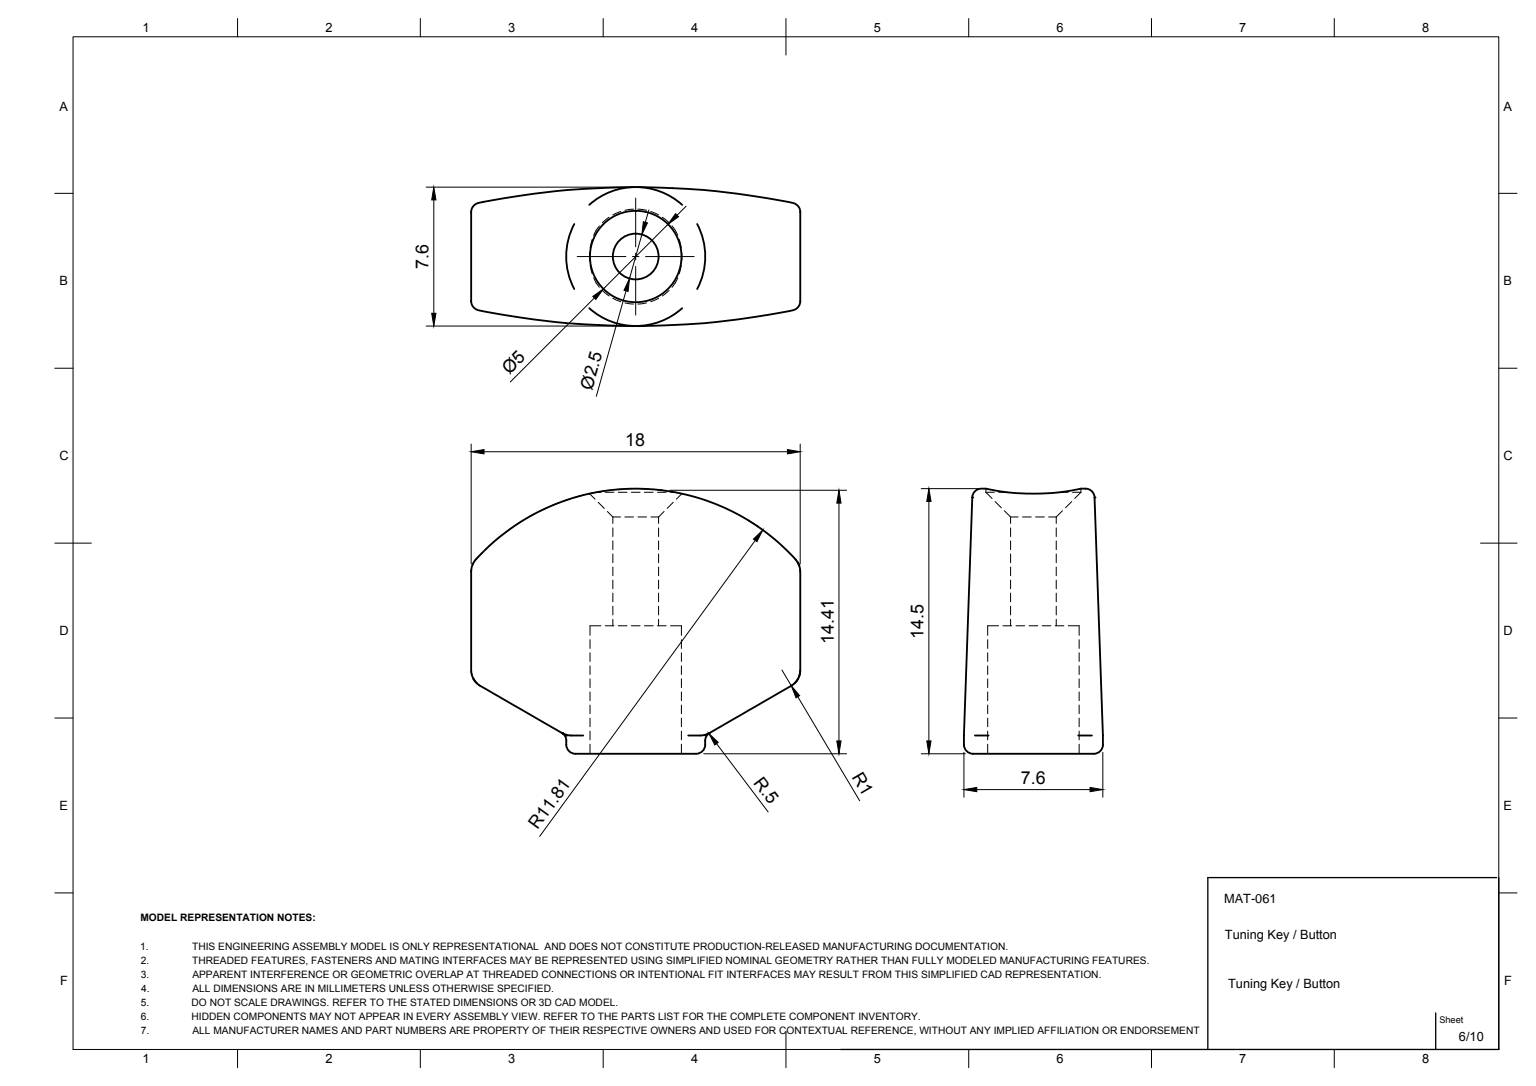
ISO-10303-21;
HEADER;
/* Generated by software containing ST-Developer
 * from STEP Tools, Inc. (www.steptools.com) 
 */

FILE_DESCRIPTION(
/* description */ ('', 'CAx-IF Rec.Pracs.---Representation and Presentation of Product Manufa
cturing Information (PMI)---4.0---2014-10-13'),
/* implementation_level */ '2;1');

FILE_NAME(
/* name */ 'Tuning Key _ Button.step',
/* time_stamp */ '2026-10-28T14:45:12+01:00',
/* author */ (''),
/* organization */ (''),
/* preprocessor_version */ 'ST-DEVELOPER v20.2',
/* originating_system */ 'Autodesk Translation Framework v15.17.0.0',
/* authorisation */ '');

FILE_SCHEMA (('AP242_MANAGED_MODEL_BASED_3D_ENGINEERING_MIM_LF { 1 0 10303 442 2 1 4 }'));
ENDSEC;

DATA;
#10=MECHANICAL_DESIGN_GEOMETRIC_PRESENTATION_REPRESENTATION('',(#263),#52164);
#84=ELLIPSE('',#9778,3.41583409365519,0.299010553745989);
#85=ELLIPSE('',#9779,1.15925578938865,0.129764384341253);
#86=ELLIPSE('',#9810,58.0067380360385,50.6192841142981);
#87=ELLIPSE('',#9813,1.18656669130194,0.53832789407732);
#88=ELLIPSE('',#9814,2.36619692333918,0.2327676175482);
#89=ELLIPSE('',#9837,58.0426595105096,50.6800723424155);
#90=ELLIPSE('',#9844,57.8529892126302,50.3590102148563);
#91=ELLIPSE('',#9882,57.6813518726037,50.0696217347841);
#128=(
BOUNDED_SURFACE()
B_SPLINE_SURFACE(3,3,((#29423,#29424,#29425,#29426,#29427,#29428,#29429,
#29430,#29431,#29432,#29433),(#29434,#29435,#29436,#29437,#29438,#29439,
#29440,#29441,#29442,#29443,#29444),(#29445,#29446,#29447,#29448,#29449,
#29450,#29451,#29452,#29453,#29454,#29455),(#29456,#29457,#29458,#29459,
#29460,#29461,#29462,#29463,#29464,#29465,#29466)),.UNSPECIFIED.,.F.,.F.,
 .F.)
B_SPLINE_SURFACE_WITH_KNOTS((4,4),(4,1,1,1,1,1,1,1,4),(0.,1.),(-0.02986974742742,
0.,0.1596527875626,0.3152888236561,0.4716393647845,0.6325142775716,0.8056128321368,
1.,1.030037265102),.UNSPECIFIED.)
GEOMETRIC_REPRESENTATION_ITEM()
RATIONAL_B_SPLINE_SURFACE(((1.021500558569,1.021500558569,1.021500558569,
1.021500558569,1.021500558569,1.021500558569,1.021500558569,1.021500558569,
1.021500558569,1.021500558569,1.021500558569),(0.9928331471435,0.9928331471435,
0.9928331471435,0.9928331471435,0.9928331471435,0.9928331471435,0.9928331471435,
0.9928331471435,0.9928331471435,0.9928331471435,0.9928331471435),(0.9928331471435,
0.9928331471435,0.9928331471435,0.9928331471435,0.9928331471435,0.9928331471435,
0.9928331471435,0.9928331471435,0.9928331471435,0.9928331471435,0.9928331471435),
(1.021500558569,1.021500558569,1.021500558569,1.021500558569,1.021500558569,
1.021500558569,1.021500558569,1.021500558569,1.021500558569,1.021500558569,
1.021500558569)))
REPRESENTATION_ITEM('')
SURFACE()
);
#129=(
BOUNDED_SURFACE()
B_SPLINE_SURFACE(3,3,((#29522,#29523,#29524,#29525,#29526,#29527,#29528,
#29529,#29530),(#29531,#29532,#29533,#29534,#29535,#29536,#29537,#29538,
#29539),(#29540,#29541,#29542,#29543,#29544,#29545,#29546,#29547,#29548),
(#29549,#29550,#29551,#29552,#29553,#29554,#29555,#29556,#29557)),
 .UNSPECIFIED.,.F.,.F.,.F.)
B_SPLINE_SURFACE_WITH_KNOTS((4,4),(4,1,1,1,1,1,4),(0.,1.),(-0.01572041923322,
0.,0.2489956052111,0.4846339404094,0.7277879443756,1.,1.015767529497),
 .UNSPECIFIED.)
GEOMETRIC_REPRESENTATION_ITEM()
RATIONAL_B_SPLINE_SURFACE(((1.20167030075,1.20167030075,1.20167030075,1.20167030075,
1.20167030075,1.20167030075,1.20167030075,1.20167030075,1.20167030075),
(0.9327765664168,0.9327765664168,0.9327765664168,0.9327765664168,0.9327765664168,
0.9327765664168,0.9327765664168,0.9327765664168,0.9327765664168),(0.9327765664168,
0.9327765664168,0.9327765664168,0.9327765664168,0.9327765664168,0.9327765664168,
0.9327765664168,0.9327765664168,0.9327765664168),(1.20167030075,1.20167030075,
1.20167030075,1.20167030075,1.20167030075,1.20167030075,1.20167030075,1.20167030075,
1.20167030075)))
REPRESENTATION_ITEM('')
SURFACE()
);
#130=(
BOUNDED_SURFACE()
B_SPLINE_SURFACE(3,3,((#29629,#29630,#29631,#29632,#29633,#29634,#29635,
#29636,#29637),(#29638,#29639,#29640,#29641,#29642,#29643,#29644,#29645,
#29646),(#29647,#29648,#29649,#29650,#29651,#29652,#29653,#29654,#29655),
(#29656,#29657,#29658,#29659,#29660,#29661,#29662,#29663,#29664)),
 .UNSPECIFIED.,.F.,.F.,.F.)
B_SPLINE_SURFACE_WITH_KNOTS((4,4),(4,1,1,1,1,1,4),(0.,1.),(-0.05556040640744,
0.,0.2510807745895,0.5005021153997,0.7496749190056,1.,1.055704479788),
 .UNSPECIFIED.)
GEOMETRIC_REPRESENTATION_ITEM()
RATIONAL_B_SPLINE_SURFACE(((1.211236736652,1.211236736652,1.211236736652,
1.211236736652,1.211236736652,1.211236736652,1.211236736652,1.211236736652,
1.211236736652),(0.9295877544494,0.9295877544494,0.9295877544494,0.9295877544494,
0.9295877544494,0.9295877544494,0.9295877544494,0.9295877544494,0.9295877544494),
(0.9295877544494,0.9295877544494,0.9295877544494,0.9295877544494,0.9295877544494,
0.9295877544494,0.9295877544494,0.9295877544494,0.9295877544494),(1.211236736652,
1.211236736652,1.211236736652,1.211236736652,1.211236736652,1.211236736652,
1.211236736652,1.211236736652,1.211236736652)))
REPRESENTATION_ITEM('')
SURFACE()
);
#131=(
BOUNDED_SURFACE()
B_SPLINE_SURFACE(3,3,((#29668,#29669,#29670,#29671,#29672,#29673,#29674,
#29675),(#29676,#29677,#29678,#29679,#29680,#29681,#29682,#29683),(#29684,
#29685,#29686,#29687,#29688,#29689,#29690,#29691),(#29692,#29693,#29694,
#29695,#29696,#29697,#29698,#29699)),.UNSPECIFIED.,.F.,.F.,.F.)
B_SPLINE_SURFACE_WITH_KNOTS((4,4),(4,1,1,1,1,4),(0.,1.),(0.8911674115136,
0.9072696780606,0.9355241084298,0.9657104248281,1.,1.001077582608),
 .UNSPECIFIED.)
GEOMETRIC_REPRESENTATION_ITEM()
RATIONAL_B_SPLINE_SURFACE(((1.199526961773,1.199526961773,1.199526961773,
1.199526961773,1.199526961773,1.199526961773,1.199526961773,1.199526961773),
(0.9334910127424,0.9334910127424,0.9334910127424,0.9334910127424,0.9334910127424,
0.9334910127424,0.9334910127424,0.9334910127424),(0.9334910127424,0.9334910127424,
0.9334910127424,0.9334910127424,0.9334910127424,0.9334910127424,0.9334910127424,
0.9334910127424),(1.199526961773,1.199526961773,1.199526961773,1.199526961773,
1.199526961773,1.199526961773,1.199526961773,1.199526961773)))
REPRESENTATION_ITEM('')
SURFACE()
);
#132=(
BOUNDED_SURFACE()
B_SPLINE_SURFACE(3,3,((#29815,#29816,#29817,#29818,#29819,#29820,#29821,
#29822,#29823,#29824,#29825),(#29826,#29827,#29828,#29829,#29830,#29831,
#29832,#29833,#29834,#29835,#29836),(#29837,#29838,#29839,#29840,#29841,
#29842,#29843,#29844,#29845,#29846,#29847),(#29848,#29849,#29850,#29851,
#29852,#29853,#29854,#29855,#29856,#29857,#29858)),.UNSPECIFIED.,.F.,.F.,
 .F.)
B_SPLINE_SURFACE_WITH_KNOTS((4,4),(4,1,1,1,1,1,1,1,4),(0.,1.),(-0.05042394646536,
0.,0.169599833297,0.3375196990485,0.507342039377,0.6686225111424,0.8285344877041,
1.,1.040577583792),.UNSPECIFIED.)
GEOMETRIC_REPRESENTATION_ITEM()
RATIONAL_B_SPLINE_SURFACE(((1.008087174025,1.008087174025,1.008087174025,
1.008087174025,1.008087174025,1.008087174025,1.008087174025,1.008087174025,
1.008087174025,1.008087174025,1.008087174025),(0.9973042753251,0.9973042753251,
0.9973042753251,0.9973042753251,0.9973042753251,0.9973042753251,0.9973042753251,
0.9973042753251,0.9973042753251,0.9973042753251,0.9973042753251),(0.9973042753251,
0.9973042753251,0.9973042753251,0.9973042753251,0.9973042753251,0.9973042753251,
0.9973042753251,0.9973042753251,0.9973042753251,0.9973042753251,0.9973042753251),
(1.008087174025,1.008087174025,1.008087174025,1.008087174025,1.008087174025,
1.008087174025,1.008087174025,1.008087174025,1.008087174025,1.008087174025,
1.008087174025)))
REPRESENTATION_ITEM('')
SURFACE()
);
#133=(
BOUNDED_SURFACE()
B_SPLINE_SURFACE(3,3,((#29905,#29906,#29907,#29908,#29909,#29910,#29911),
(#29912,#29913,#29914,#29915,#29916,#29917,#29918),(#29919,#29920,#29921,
#29922,#29923,#29924,#29925),(#29926,#29927,#29928,#29929,#29930,#29931,
#29932)),.UNSPECIFIED.,.F.,.F.,.F.)
B_SPLINE_SURFACE_WITH_KNOTS((4,4),(4,1,1,1,4),(0.,1.),(0.112613801722,0.3198611143952,
0.6533271535514,1.,1.02662543373),.UNSPECIFIED.)
GEOMETRIC_REPRESENTATION_ITEM()
RATIONAL_B_SPLINE_SURFACE(((1.133923634678,1.133923634678,1.133923634678,
1.133923634678,1.133923634678,1.133923634678,1.133923634678),(0.9553587884407,
0.9553587884407,0.9553587884407,0.9553587884407,0.9553587884407,0.9553587884407,
0.9553587884407),(0.9553587884407,0.9553587884407,0.9553587884407,0.9553587884407,
0.9553587884407,0.9553587884407,0.9553587884407),(1.133923634678,1.133923634678,
1.133923634678,1.133923634678,1.133923634678,1.133923634678,1.133923634678)))
REPRESENTATION_ITEM('')
SURFACE()
);
#134=(
BOUNDED_SURFACE()
B_SPLINE_SURFACE(3,3,((#30489,#30490,#30491,#30492,#30493,#30494,#30495,
#30496,#30497,#30498,#30499,#30500,#30501,#30502,#30503,#30504,#30505,#30506,
#30507),(#30508,#30509,#30510,#30511,#30512,#30513,#30514,#30515,#30516,
#30517,#30518,#30519,#30520,#30521,#30522,#30523,#30524,#30525,#30526),
(#30527,#30528,#30529,#30530,#30531,#30532,#30533,#30534,#30535,#30536,
#30537,#30538,#30539,#30540,#30541,#30542,#30543,#30544,#30545),(#30546,
#30547,#30548,#30549,#30550,#30551,#30552,#30553,#30554,#30555,#30556,#30557,
#30558,#30559,#30560,#30561,#30562,#30563,#30564)),.UNSPECIFIED.,.F.,.F.,
 .F.)
B_SPLINE_SURFACE_WITH_KNOTS((4,4),(4,1,1,1,1,1,1,1,1,1,1,1,1,1,1,1,4),(0.,
1.),(-0.01076426746052,0.,0.04152389901163,0.08394379225383,0.1302342687653,
0.1804523447143,0.2349355052965,0.2939338029968,0.3580057487009,0.4275129366519,
0.5025423241298,0.5839356639567,0.6731830882241,0.771794295847,0.880557504522,
1.,1.009808133051),.UNSPECIFIED.)
GEOMETRIC_REPRESENTATION_ITEM()
RATIONAL_B_SPLINE_SURFACE(((1.088372924818,1.088372924818,1.088372924818,
1.088372924818,1.088372924818,1.088372924818,1.088372924818,1.088372924818,
1.088372924818,1.088372924818,1.088372924818,1.088372924818,1.088372924818,
1.088372924818,1.088372924818,1.088372924818,1.088372924818,1.088372924818,
1.088372924818),(0.9705423583942,0.9705423583942,0.9705423583942,0.9705423583942,
0.9705423583942,0.9705423583942,0.9705423583942,0.9705423583942,0.9705423583942,
0.9705423583942,0.9705423583942,0.9705423583942,0.9705423583942,0.9705423583942,
0.9705423583942,0.9705423583942,0.9705423583942,0.9705423583942,0.9705423583942),
(0.9705423583942,0.9705423583942,0.9705423583942,0.9705423583942,0.9705423583942,
0.9705423583942,0.9705423583942,0.9705423583942,0.9705423583942,0.9705423583942,
0.9705423583942,0.9705423583942,0.9705423583942,0.9705423583942,0.9705423583942,
0.9705423583942,0.9705423583942,0.9705423583942,0.9705423583942),(1.088372924818,
1.088372924818,1.088372924818,1.088372924818,1.088372924818,1.088372924818,
1.088372924818,1.088372924818,1.088372924818,1.088372924818,1.088372924818,
1.088372924818,1.088372924818,1.088372924818,1.088372924818,1.088372924818,
1.088372924818,1.088372924818,1.088372924818)))
REPRESENTATION_ITEM('')
SURFACE()
);
#135=(
BOUNDED_SURFACE()
B_SPLINE_SURFACE(3,3,((#30667,#30668,#30669,#30670,#30671,#30672,#30673,
#30674,#30675,#30676),(#30677,#30678,#30679,#30680,#30681,#30682,#30683,
#30684,#30685,#30686),(#30687,#30688,#30689,#30690,#30691,#30692,#30693,
#30694,#30695,#30696),(#30697,#30698,#30699,#30700,#30701,#30702,#30703,
#30704,#30705,#30706)),.UNSPECIFIED.,.F.,.F.,.F.)
B_SPLINE_SURFACE_WITH_KNOTS((4,4),(4,1,1,1,1,1,1,4),(0.,1.),(0.03540281776569,
0.1234679415061,0.2632035734035,0.4203296727883,0.5957836491344,0.7892685013705,
1.,1.00911688994),.UNSPECIFIED.)
GEOMETRIC_REPRESENTATION_ITEM()
RATIONAL_B_SPLINE_SURFACE(((1.211236248281,1.211236248281,1.211236248281,
1.211236248281,1.211236248281,1.211236248281,1.211236248281,1.211236248281,
1.211236248281,1.211236248281),(0.9295879172397,0.9295879172397,0.9295879172397,
0.9295879172397,0.9295879172397,0.9295879172397,0.9295879172397,0.9295879172397,
0.9295879172397,0.9295879172397),(0.9295879172397,0.9295879172397,0.9295879172397,
0.9295879172397,0.9295879172397,0.9295879172397,0.9295879172397,0.9295879172397,
0.9295879172397,0.9295879172397),(1.211236248281,1.211236248281,1.211236248281,
1.211236248281,1.211236248281,1.211236248281,1.211236248281,1.211236248281,
1.211236248281,1.211236248281)))
REPRESENTATION_ITEM('')
SURFACE()
);
#136=(
BOUNDED_SURFACE()
B_SPLINE_SURFACE(3,3,((#30720,#30721,#30722,#30723,#30724,#30725,#30726,
#30727,#30728,#30729,#30730,#30731),(#30732,#30733,#30734,#30735,#30736,
#30737,#30738,#30739,#30740,#30741,#30742,#30743),(#30744,#30745,#30746,
#30747,#30748,#30749,#30750,#30751,#30752,#30753,#30754,#30755),(#30756,
#30757,#30758,#30759,#30760,#30761,#30762,#30763,#30764,#30765,#30766,#30767)),
 .UNSPECIFIED.,.F.,.F.,.F.)
B_SPLINE_SURFACE_WITH_KNOTS((4,4),(4,1,1,1,1,1,1,1,1,4),(0.,1.),(-0.1526180119247,
0.,0.1440925301464,0.2801219903111,0.411439159359,0.5434056701394,0.683264528579,
0.8346596058499,1.,1.152833582057),.UNSPECIFIED.)
GEOMETRIC_REPRESENTATION_ITEM()
RATIONAL_B_SPLINE_SURFACE(((1.000094023891,1.000094023891,1.000094023891,
1.000094023891,1.000094023891,1.000094023891,1.000094023891,1.000094023891,
1.000094023891,1.000094023891,1.000094023891,1.000094023891),(0.9999686587029,
0.9999686587029,0.9999686587029,0.9999686587029,0.9999686587029,0.9999686587029,
0.9999686587029,0.9999686587029,0.9999686587029,0.9999686587029,0.9999686587029,
0.9999686587029),(0.9999686587029,0.9999686587029,0.9999686587029,0.9999686587029,
0.9999686587029,0.9999686587029,0.9999686587029,0.9999686587029,0.9999686587029,
0.9999686587029,0.9999686587029,0.9999686587029),(1.000094023891,1.000094023891,
1.000094023891,1.000094023891,1.000094023891,1.000094023891,1.000094023891,
1.000094023891,1.000094023891,1.000094023891,1.000094023891,1.000094023891)))
REPRESENTATION_ITEM('')
SURFACE()
);
#137=(
BOUNDED_SURFACE()
B_SPLINE_SURFACE(3,3,((#30792,#30793,#30794,#30795,#30796,#30797,#30798,
#30799,#30800,#30801),(#30802,#30803,#30804,#30805,#30806,#30807,#30808,
#30809,#30810,#30811),(#30812,#30813,#30814,#30815,#30816,#30817,#30818,
#30819,#30820,#30821),(#30822,#30823,#30824,#30825,#30826,#30827,#30828,
#30829,#30830,#30831)),.UNSPECIFIED.,.F.,.F.,.F.)
B_SPLINE_SURFACE_WITH_KNOTS((4,4),(4,1,1,1,1,1,1,4),(0.,1.),(-0.009053405764055,
0.,0.2128253131464,0.406710340465,0.5817418357976,0.7383188923361,0.8773475428248,
0.9585687317144),.UNSPECIFIED.)
GEOMETRIC_REPRESENTATION_ITEM()
RATIONAL_B_SPLINE_SURFACE(((1.211237524847,1.211237524847,1.211237524847,
1.211237524847,1.211237524847,1.211237524847,1.211237524847,1.211237524847,
1.211237524847,1.211237524847),(0.9295874917176,0.9295874917176,0.9295874917176,
0.9295874917176,0.9295874917176,0.9295874917176,0.9295874917176,0.9295874917176,
0.9295874917176,0.9295874917176),(0.9295874917176,0.9295874917176,0.9295874917176,
0.9295874917176,0.9295874917176,0.9295874917176,0.9295874917176,0.9295874917176,
0.9295874917176,0.9295874917176),(1.211237524847,1.211237524847,1.211237524847,
1.211237524847,1.211237524847,1.211237524847,1.211237524847,1.211237524847,
1.211237524847,1.211237524847)))
REPRESENTATION_ITEM('')
SURFACE()
);
#138=(
BOUNDED_SURFACE()
B_SPLINE_SURFACE(3,3,((#30920,#30921,#30922,#30923,#30924,#30925,#30926,
#30927,#30928,#30929,#30930,#30931,#30932,#30933,#30934,#30935,#30936,#30937),
(#30938,#30939,#30940,#30941,#30942,#30943,#30944,#30945,#30946,#30947,
#30948,#30949,#30950,#30951,#30952,#30953,#30954,#30955),(#30956,#30957,
#30958,#30959,#30960,#30961,#30962,#30963,#30964,#30965,#30966,#30967,#30968,
#30969,#30970,#30971,#30972,#30973),(#30974,#30975,#30976,#30977,#30978,
#30979,#30980,#30981,#30982,#30983,#30984,#30985,#30986,#30987,#30988,#30989,
#30990,#30991)),.UNSPECIFIED.,.F.,.F.,.F.)
B_SPLINE_SURFACE_WITH_KNOTS((4,4),(4,1,1,1,1,1,1,1,1,1,1,1,1,1,1,4),(0.,
1.),(-0.009797090891185,0.,0.1252864769206,0.2381332273305,0.3395214867104,
0.4311702756132,0.514794596407,0.5913458810939,0.661337900673,0.7254151205028,
0.7843391271164,0.8380935847788,0.8886737238569,0.9411160876018,1.,1.010696795736),
 .UNSPECIFIED.)
GEOMETRIC_REPRESENTATION_ITEM()
RATIONAL_B_SPLINE_SURFACE(((1.088374512803,1.088374512803,1.088374512803,
1.088374512803,1.088374512803,1.088374512803,1.088374512803,1.088374512803,
1.088374512803,1.088374512803,1.088374512803,1.088374512803,1.088374512803,
1.088374512803,1.088374512803,1.088374512803,1.088374512803,1.088374512803),
(0.9705418290656,0.9705418290656,0.9705418290656,0.9705418290656,0.9705418290656,
0.9705418290656,0.9705418290656,0.9705418290655,0.9705418290656,0.9705418290656,
0.9705418290656,0.9705418290656,0.9705418290655,0.9705418290656,0.9705418290656,
0.9705418290655,0.9705418290656,0.9705418290656),(0.9705418290656,0.9705418290656,
0.9705418290656,0.9705418290656,0.9705418290656,0.9705418290656,0.9705418290656,
0.9705418290655,0.9705418290656,0.9705418290656,0.9705418290656,0.9705418290656,
0.9705418290655,0.9705418290656,0.9705418290656,0.9705418290655,0.9705418290656,
0.9705418290656),(1.088374512803,1.088374512803,1.088374512803,1.088374512803,
1.088374512803,1.088374512803,1.088374512803,1.088374512803,1.088374512803,
1.088374512803,1.088374512803,1.088374512803,1.088374512803,1.088374512803,
1.088374512803,1.088374512803,1.088374512803,1.088374512803)))
REPRESENTATION_ITEM('')
SURFACE()
);
#139=(
BOUNDED_SURFACE()
B_SPLINE_SURFACE(3,3,((#30993,#30994,#30995,#30996,#30997,#30998,#30999,
#31000,#31001),(#31002,#31003,#31004,#31005,#31006,#31007,#31008,#31009,
#31010),(#31011,#31012,#31013,#31014,#31015,#31016,#31017,#31018,#31019),
(#31020,#31021,#31022,#31023,#31024,#31025,#31026,#31027,#31028)),
 .UNSPECIFIED.,.F.,.F.,.F.)
B_SPLINE_SURFACE_WITH_KNOTS((4,4),(4,1,1,1,1,1,4),(0.,1.),(-0.01572041923323,
0.,0.2489956052094,0.4846339404077,0.7277879443747,1.,1.015767529497),
 .UNSPECIFIED.)
GEOMETRIC_REPRESENTATION_ITEM()
RATIONAL_B_SPLINE_SURFACE(((1.20167030075,1.20167030075,1.20167030075,1.20167030075,
1.20167030075,1.20167030075,1.20167030075,1.20167030075,1.20167030075),
(0.9327765664168,0.9327765664168,0.9327765664168,0.9327765664168,0.9327765664168,
0.9327765664168,0.9327765664168,0.9327765664168,0.9327765664168),(0.9327765664168,
0.9327765664168,0.9327765664168,0.9327765664168,0.9327765664168,0.9327765664168,
0.9327765664168,0.9327765664168,0.9327765664168),(1.20167030075,1.20167030075,
1.20167030075,1.20167030075,1.20167030075,1.20167030075,1.20167030075,1.20167030075,
1.20167030075)))
REPRESENTATION_ITEM('')
SURFACE()
);
#140=(
BOUNDED_SURFACE()
B_SPLINE_SURFACE(3,3,((#31065,#31066,#31067,#31068,#31069,#31070,#31071,
#31072,#31073),(#31074,#31075,#31076,#31077,#31078,#31079,#31080,#31081,
#31082),(#31083,#31084,#31085,#31086,#31087,#31088,#31089,#31090,#31091),
(#31092,#31093,#31094,#31095,#31096,#31097,#31098,#31099,#31100)),
 .UNSPECIFIED.,.F.,.F.,.F.)
B_SPLINE_SURFACE_WITH_KNOTS((4,4),(4,1,1,1,1,1,4),(0.,1.),(-0.05556027674448,
0.,0.2486256441043,0.4972385660022,0.747219976182,1.,1.055704281495),
 .UNSPECIFIED.)
GEOMETRIC_REPRESENTATION_ITEM()
RATIONAL_B_SPLINE_SURFACE(((1.211236736616,1.211236736616,1.211236736616,
1.211236736616,1.211236736616,1.211236736616,1.211236736616,1.211236736616,
1.211236736616),(0.9295877544614,0.9295877544614,0.9295877544614,0.9295877544614,
0.9295877544614,0.9295877544614,0.9295877544614,0.9295877544614,0.9295877544614),
(0.9295877544614,0.9295877544614,0.9295877544614,0.9295877544614,0.9295877544614,
0.9295877544614,0.9295877544614,0.9295877544614,0.9295877544614),(1.211236736616,
1.211236736616,1.211236736616,1.211236736616,1.211236736616,1.211236736616,
1.211236736616,1.211236736616,1.211236736616)))
REPRESENTATION_ITEM('')
SURFACE()
);
#141=(
BOUNDED_SURFACE()
B_SPLINE_SURFACE(3,3,((#31104,#31105,#31106,#31107,#31108,#31109,#31110,
#31111),(#31112,#31113,#31114,#31115,#31116,#31117,#31118,#31119),(#31120,
#31121,#31122,#31123,#31124,#31125,#31126,#31127),(#31128,#31129,#31130,
#31131,#31132,#31133,#31134,#31135)),.UNSPECIFIED.,.F.,.F.,.F.)
B_SPLINE_SURFACE_WITH_KNOTS((4,4),(4,1,1,1,1,4),(0.,1.),(0.8864361758264,
0.9023348460698,0.9320880776135,0.9638776326039,1.,1.001124438805),
 .UNSPECIFIED.)
GEOMETRIC_REPRESENTATION_ITEM()
RATIONAL_B_SPLINE_SURFACE(((1.199526961777,1.199526961777,1.199526961777,
1.199526961777,1.199526961777,1.199526961777,1.199526961777,1.199526961777),
(0.933491012741,0.933491012741,0.933491012741,0.933491012741,0.933491012741,
0.933491012741,0.933491012741,0.933491012741),(0.933491012741,0.933491012741,
0.933491012741,0.933491012741,0.933491012741,0.933491012741,0.933491012741,
0.933491012741),(1.199526961777,1.199526961777,1.199526961777,1.199526961777,
1.199526961777,1.199526961777,1.199526961777,1.199526961777)))
REPRESENTATION_ITEM('')
SURFACE()
);
#142=(
BOUNDED_SURFACE()
B_SPLINE_SURFACE(3,3,((#31139,#31140,#31141,#31142,#31143,#31144,#31145,
#31146,#31147,#31148),(#31149,#31150,#31151,#31152,#31153,#31154,#31155,
#31156,#31157,#31158),(#31159,#31160,#31161,#31162,#31163,#31164,#31165,
#31166,#31167,#31168),(#31169,#31170,#31171,#31172,#31173,#31174,#31175,
#31176,#31177,#31178)),.UNSPECIFIED.,.F.,.F.,.F.)
B_SPLINE_SURFACE_WITH_KNOTS((4,4),(4,1,1,1,1,1,1,4),(0.,1.),(-0.02782802324678,
0.,0.206830483526,0.4072723973775,0.5982739087583,0.7917037265225,1.,1.028080129965),
 .UNSPECIFIED.)
GEOMETRIC_REPRESENTATION_ITEM()
RATIONAL_B_SPLINE_SURFACE(((1.187634479555,1.187634479555,1.187634479555,
1.187634479555,1.187634479555,1.187634479555,1.187634479555,1.187634479555,
1.187634479555,1.187634479555),(0.9374551734818,0.9374551734818,0.9374551734818,
0.9374551734818,0.9374551734818,0.9374551734818,0.9374551734818,0.9374551734818,
0.9374551734818,0.9374551734818),(0.9374551734818,0.9374551734818,0.9374551734818,
0.9374551734818,0.9374551734818,0.9374551734818,0.9374551734818,0.9374551734818,
0.9374551734818,0.9374551734818),(1.187634479555,1.187634479555,1.187634479555,
1.187634479555,1.187634479555,1.187634479555,1.187634479555,1.187634479555,
1.187634479555,1.187634479555)))
REPRESENTATION_ITEM('')
SURFACE()
);
#143=(
BOUNDED_SURFACE()
B_SPLINE_SURFACE(3,3,((#31284,#31285,#31286,#31287,#31288,#31289,#31290,
#31291,#31292,#31293),(#31294,#31295,#31296,#31297,#31298,#31299,#31300,
#31301,#31302,#31303),(#31304,#31305,#31306,#31307,#31308,#31309,#31310,
#31311,#31312,#31313),(#31314,#31315,#31316,#31317,#31318,#31319,#31320,
#31321,#31322,#31323)),.UNSPECIFIED.,.F.,.F.,.F.)
B_SPLINE_SURFACE_WITH_KNOTS((4,4),(4,1,1,1,1,1,1,4),(0.,1.),(-0.02810100933582,
0.,0.2037887769512,0.4025777380169,0.5941765368876,0.7898232262628,1.,1.027817051165),
 .UNSPECIFIED.)
GEOMETRIC_REPRESENTATION_ITEM()
RATIONAL_B_SPLINE_SURFACE(((1.18763448144,1.18763448144,1.18763448144,1.18763448144,
1.18763448144,1.18763448144,1.18763448144,1.18763448144,1.18763448144,1.18763448144),
(0.9374551728533,0.9374551728533,0.9374551728533,0.9374551728533,0.9374551728533,
0.9374551728533,0.9374551728533,0.9374551728533,0.9374551728533,0.9374551728533),
(0.9374551728533,0.9374551728533,0.9374551728533,0.9374551728533,0.9374551728533,
0.9374551728533,0.9374551728533,0.9374551728533,0.9374551728533,0.9374551728533),
(1.18763448144,1.18763448144,1.18763448144,1.18763448144,1.18763448144,
1.18763448144,1.18763448144,1.18763448144,1.18763448144,1.18763448144)))
REPRESENTATION_ITEM('')
SURFACE()
);
#144=(
BOUNDED_SURFACE()
B_SPLINE_SURFACE(3,3,((#31368,#31369,#31370,#31371,#31372,#31373,#31374,
#31375),(#31376,#31377,#31378,#31379,#31380,#31381,#31382,#31383),(#31384,
#31385,#31386,#31387,#31388,#31389,#31390,#31391),(#31392,#31393,#31394,
#31395,#31396,#31397,#31398,#31399)),.UNSPECIFIED.,.F.,.F.,.F.)
B_SPLINE_SURFACE_WITH_KNOTS((4,4),(4,1,1,1,1,4),(0.,1.),(-0.001124474187882,
0.,0.0292220127923,0.0587438887651,0.09152259808643,0.1135644482631),
 .UNSPECIFIED.)
GEOMETRIC_REPRESENTATION_ITEM()
RATIONAL_B_SPLINE_SURFACE(((1.199526978638,1.199526978638,1.199526978638,
1.199526978638,1.199526978638,1.199526978638,1.199526978638,1.199526978638),
(0.9334910071206,0.9334910071206,0.9334910071206,0.9334910071206,0.9334910071206,
0.9334910071206,0.9334910071206,0.9334910071206),(0.9334910071206,0.9334910071206,
0.9334910071206,0.9334910071206,0.9334910071206,0.9334910071206,0.9334910071206,
0.9334910071206),(1.199526978638,1.199526978638,1.199526978638,1.199526978638,
1.199526978638,1.199526978638,1.199526978638,1.199526978638)))
REPRESENTATION_ITEM('')
SURFACE()
);
#145=(
BOUNDED_SURFACE()
B_SPLINE_SURFACE(3,3,((#31403,#31404,#31405,#31406,#31407,#31408,#31409,
#31410,#31411,#31412,#31413,#31414),(#31415,#31416,#31417,#31418,#31419,
#31420,#31421,#31422,#31423,#31424,#31425,#31426),(#31427,#31428,#31429,
#31430,#31431,#31432,#31433,#31434,#31435,#31436,#31437,#31438),(#31439,
#31440,#31441,#31442,#31443,#31444,#31445,#31446,#31447,#31448,#31449,#31450)),
 .UNSPECIFIED.,.F.,.F.,.F.)
B_SPLINE_SURFACE_WITH_KNOTS((4,4),(4,1,1,1,1,1,1,1,1,4),(0.,1.),(0.01735834385764,
0.1111047299147,0.222221140213,0.3333544708185,0.4444847206802,0.5555988587856,
0.6667216990803,0.777841116212,0.8889364520316,0.9880643576882),
 .UNSPECIFIED.)
GEOMETRIC_REPRESENTATION_ITEM()
RATIONAL_B_SPLINE_SURFACE(((1.211236726429,1.211236726429,1.211236726429,
1.211236726429,1.211236726429,1.211236726429,1.211236726429,1.211236726429,
1.211236726429,1.211236726429,1.211236726429,1.211236726429),(0.929587757857,
0.929587757857,0.929587757857,0.929587757857,0.929587757857,0.929587757857,
0.929587757857,0.929587757857,0.929587757857,0.929587757857,0.929587757857,
0.929587757857),(0.929587757857,0.929587757857,0.929587757857,0.929587757857,
0.929587757857,0.929587757857,0.929587757857,0.929587757857,0.929587757857,
0.929587757857,0.929587757857,0.929587757857),(1.211236726429,1.211236726429,
1.211236726429,1.211236726429,1.211236726429,1.211236726429,1.211236726429,
1.211236726429,1.211236726429,1.211236726429,1.211236726429,1.211236726429)))
REPRESENTATION_ITEM('')
SURFACE()
);
#146=(
BOUNDED_SURFACE()
B_SPLINE_SURFACE(3,3,((#31488,#31489,#31490,#31491,#31492,#31493,#31494,
#31495,#31496),(#31497,#31498,#31499,#31500,#31501,#31502,#31503,#31504,
#31505),(#31506,#31507,#31508,#31509,#31510,#31511,#31512,#31513,#31514),
(#31515,#31516,#31517,#31518,#31519,#31520,#31521,#31522,#31523)),
 .UNSPECIFIED.,.F.,.F.,.F.)
B_SPLINE_SURFACE_WITH_KNOTS((4,4),(4,1,1,1,1,1,4),(0.,1.),(-0.01575975614392,
0.,0.2456294260624,0.4801888085378,0.72700648837,1.,1.015733967826),
 .UNSPECIFIED.)
GEOMETRIC_REPRESENTATION_ITEM()
RATIONAL_B_SPLINE_SURFACE(((1.201670188537,1.201670188537,1.201670188537,
1.201670188537,1.201670188537,1.201670188537,1.201670188537,1.201670188537,
1.201670188537),(0.9327766038211,0.9327766038211,0.9327766038211,0.9327766038211,
0.9327766038211,0.9327766038211,0.9327766038211,0.9327766038211,0.9327766038211),
(0.9327766038211,0.9327766038211,0.9327766038211,0.9327766038211,0.9327766038211,
0.9327766038211,0.9327766038211,0.9327766038211,0.9327766038211),(1.201670188537,
1.201670188537,1.201670188537,1.201670188537,1.201670188537,1.201670188537,
1.201670188537,1.201670188537,1.201670188537)))
REPRESENTATION_ITEM('')
SURFACE()
);
#147=(
BOUNDED_SURFACE()
B_SPLINE_SURFACE(3,3,((#31570,#31571,#31572,#31573,#31574,#31575,#31576,
#31577,#31578,#31579),(#31580,#31581,#31582,#31583,#31584,#31585,#31586,
#31587,#31588,#31589),(#31590,#31591,#31592,#31593,#31594,#31595,#31596,
#31597,#31598,#31599),(#31600,#31601,#31602,#31603,#31604,#31605,#31606,
#31607,#31608,#31609)),.UNSPECIFIED.,.F.,.F.,.F.)
B_SPLINE_SURFACE_WITH_KNOTS((4,4),(4,1,1,1,1,1,1,4),(0.,1.),(-0.02987479217279,
0.,0.1922564273876,0.376033241946,0.5650637118402,0.769737337347,1.,1.030040321285),
 .UNSPECIFIED.)
GEOMETRIC_REPRESENTATION_ITEM()
RATIONAL_B_SPLINE_SURFACE(((1.02150055857,1.02150055857,1.02150055857,1.02150055857,
1.02150055857,1.02150055857,1.02150055857,1.02150055857,1.02150055857,1.02150055857),
(0.9928331471434,0.9928331471434,0.9928331471434,0.9928331471434,0.9928331471434,
0.9928331471434,0.9928331471434,0.9928331471434,0.9928331471434,0.9928331471434),
(0.9928331471434,0.9928331471434,0.9928331471434,0.9928331471434,0.9928331471434,
0.9928331471434,0.9928331471434,0.9928331471434,0.9928331471434,0.9928331471434),
(1.02150055857,1.02150055857,1.02150055857,1.02150055857,1.02150055857,
1.02150055857,1.02150055857,1.02150055857,1.02150055857,1.02150055857)))
REPRESENTATION_ITEM('')
SURFACE()
);
#148=(
BOUNDED_SURFACE()
B_SPLINE_SURFACE(3,3,((#31612,#31613,#31614,#31615,#31616,#31617,#31618,
#31619,#31620),(#31621,#31622,#31623,#31624,#31625,#31626,#31627,#31628,
#31629),(#31630,#31631,#31632,#31633,#31634,#31635,#31636,#31637,#31638),
(#31639,#31640,#31641,#31642,#31643,#31644,#31645,#31646,#31647)),
 .UNSPECIFIED.,.F.,.F.,.F.)
B_SPLINE_SURFACE_WITH_KNOTS((4,4),(4,1,1,1,1,1,4),(0.,1.),(-0.05038062996365,
0.,0.2351349496917,0.4696037900664,0.7241664476852,1.,1.040579001464),
 .UNSPECIFIED.)
GEOMETRIC_REPRESENTATION_ITEM()
RATIONAL_B_SPLINE_SURFACE(((1.008087784169,1.008087784169,1.008087784169,
1.008087784169,1.008087784169,1.008087784169,1.008087784169,1.008087784169,
1.008087784169),(0.9973040719437,0.9973040719437,0.9973040719437,0.9973040719437,
0.9973040719437,0.9973040719437,0.9973040719437,0.9973040719437,0.9973040719437),
(0.9973040719437,0.9973040719437,0.9973040719437,0.9973040719437,0.9973040719437,
0.9973040719437,0.9973040719437,0.9973040719437,0.9973040719437),(1.008087784169,
1.008087784169,1.008087784169,1.008087784169,1.008087784169,1.008087784169,
1.008087784169,1.008087784169,1.008087784169)))
REPRESENTATION_ITEM('')
SURFACE()
);
#149=(
BOUNDED_SURFACE()
B_SPLINE_SURFACE(3,3,((#31685,#31686,#31687,#31688,#31689,#31690,#31691),
(#31692,#31693,#31694,#31695,#31696,#31697,#31698),(#31699,#31700,#31701,
#31702,#31703,#31704,#31705),(#31706,#31707,#31708,#31709,#31710,#31711,
#31712)),.UNSPECIFIED.,.F.,.F.,.F.)
B_SPLINE_SURFACE_WITH_KNOTS((4,4),(4,1,1,1,4),(0.,1.),(-0.02191865670978,
0.,0.3711108307934,0.7030029884295,0.8666418147817),.UNSPECIFIED.)
GEOMETRIC_REPRESENTATION_ITEM()
RATIONAL_B_SPLINE_SURFACE(((1.201671391236,1.201671391236,1.201671391236,
1.201671391236,1.201671391236,1.201671391236,1.201671391236),(0.9327762029212,
0.9327762029212,0.9327762029212,0.9327762029212,0.9327762029212,0.9327762029212,
0.9327762029212),(0.9327762029212,0.9327762029212,0.9327762029212,0.9327762029212,
0.9327762029212,0.9327762029212,0.9327762029212),(1.201671391236,1.201671391236,
1.201671391236,1.201671391236,1.201671391236,1.201671391236,1.201671391236)))
REPRESENTATION_ITEM('')
SURFACE()
);
#150=(
BOUNDED_SURFACE()
B_SPLINE_SURFACE(3,3,((#31714,#31715,#31716,#31717,#31718,#31719,#31720,
#31721),(#31722,#31723,#31724,#31725,#31726,#31727,#31728,#31729),(#31730,
#31731,#31732,#31733,#31734,#31735,#31736,#31737),(#31738,#31739,#31740,
#31741,#31742,#31743,#31744,#31745)),.UNSPECIFIED.,.F.,.F.,.F.)
B_SPLINE_SURFACE_WITH_KNOTS((4,4),(4,1,1,1,1,4),(0.,1.),(-0.01121526784147,
0.,0.3190655160223,0.6396471045238,1.,1.011194064343),.UNSPECIFIED.)
GEOMETRIC_REPRESENTATION_ITEM()
RATIONAL_B_SPLINE_SURFACE(((1.095350229527,1.095350229527,1.095350229527,
1.095350229527,1.095350229527,1.095350229527,1.095350229527,1.095350229527),
(0.9682165901577,0.9682165901577,0.9682165901577,0.9682165901577,0.9682165901577,
0.9682165901577,0.9682165901577,0.9682165901577),(0.9682165901577,0.9682165901577,
0.9682165901577,0.9682165901577,0.9682165901577,0.9682165901577,0.9682165901577,
0.9682165901577),(1.095350229527,1.095350229527,1.095350229527,1.095350229527,
1.095350229527,1.095350229527,1.095350229527,1.095350229527)))
REPRESENTATION_ITEM('')
SURFACE()
);
#151=(
BOUNDED_SURFACE()
B_SPLINE_SURFACE(3,3,((#31747,#31748,#31749,#31750,#31751,#31752,#31753,
#31754),(#31755,#31756,#31757,#31758,#31759,#31760,#31761,#31762),(#31763,
#31764,#31765,#31766,#31767,#31768,#31769,#31770),(#31771,#31772,#31773,
#31774,#31775,#31776,#31777,#31778)),.UNSPECIFIED.,.F.,.F.,.F.)
B_SPLINE_SURFACE_WITH_KNOTS((4,4),(4,1,1,1,1,4),(0.,1.),(-0.01123151966199,
0.,0.3226423274774,0.6411748598112,1.,1.011214131254),.UNSPECIFIED.)
GEOMETRIC_REPRESENTATION_ITEM()
RATIONAL_B_SPLINE_SURFACE(((1.095350237894,1.095350237894,1.095350237894,
1.095350237894,1.095350237894,1.095350237894,1.095350237894,1.095350237894),
(0.9682165873688,0.9682165873688,0.9682165873688,0.9682165873688,0.9682165873688,
0.9682165873688,0.9682165873688,0.9682165873688),(0.9682165873688,0.9682165873688,
0.9682165873688,0.9682165873688,0.9682165873688,0.9682165873688,0.9682165873688,
0.9682165873688),(1.095350237894,1.095350237894,1.095350237894,1.095350237894,
1.095350237894,1.095350237894,1.095350237894,1.095350237894)))
REPRESENTATION_ITEM('')
SURFACE()
);
#152=(
BOUNDED_SURFACE()
B_SPLINE_SURFACE(3,3,((#31780,#31781,#31782,#31783,#31784,#31785,#31786),
(#31787,#31788,#31789,#31790,#31791,#31792,#31793),(#31794,#31795,#31796,
#31797,#31798,#31799,#31800),(#31801,#31802,#31803,#31804,#31805,#31806,
#31807)),.UNSPECIFIED.,.F.,.F.,.F.)
B_SPLINE_SURFACE_WITH_KNOTS((4,4),(4,1,1,1,4),(0.,1.),(0.1126138017486,
0.319861120519,0.6533271596459,1.,1.026625433703),.UNSPECIFIED.)
GEOMETRIC_REPRESENTATION_ITEM()
RATIONAL_B_SPLINE_SURFACE(((1.133923637937,1.133923637937,1.133923637937,
1.133923637937,1.133923637937,1.133923637937,1.133923637937),(0.9553587873545,
0.9553587873545,0.9553587873545,0.9553587873545,0.9553587873545,0.9553587873545,
0.9553587873545),(0.9553587873545,0.9553587873545,0.9553587873545,0.9553587873545,
0.9553587873545,0.9553587873545,0.9553587873545),(1.133923637937,1.133923637937,
1.133923637937,1.133923637937,1.133923637937,1.133923637937,1.133923637937)))
REPRESENTATION_ITEM('')
SURFACE()
);
#153=(
BOUNDED_SURFACE()
B_SPLINE_SURFACE(3,3,((#31844,#31845,#31846,#31847,#31848,#31849,#31850,
#31851,#31852,#31853,#31854),(#31855,#31856,#31857,#31858,#31859,#31860,
#31861,#31862,#31863,#31864,#31865),(#31866,#31867,#31868,#31869,#31870,
#31871,#31872,#31873,#31874,#31875,#31876),(#31877,#31878,#31879,#31880,
#31881,#31882,#31883,#31884,#31885,#31886,#31887)),.UNSPECIFIED.,.F.,.F.,
 .F.)
B_SPLINE_SURFACE_WITH_KNOTS((4,4),(4,1,1,1,1,1,1,1,4),(0.,1.),(-0.04051174551792,
0.,0.1601684695697,0.3176853418238,0.4756542837724,0.6362846105788,0.8070461231236,
1.,1.048408689707),.UNSPECIFIED.)
GEOMETRIC_REPRESENTATION_ITEM()
RATIONAL_B_SPLINE_SURFACE(((1.008087174024,1.008087174024,1.008087174024,
1.008087174024,1.008087174024,1.008087174024,1.008087174024,1.008087174024,
1.008087174024,1.008087174024,1.008087174024),(0.9973042753252,0.9973042753252,
0.9973042753252,0.9973042753252,0.9973042753252,0.9973042753252,0.9973042753252,
0.9973042753252,0.9973042753252,0.9973042753252,0.9973042753252),(0.9973042753252,
0.9973042753252,0.9973042753252,0.9973042753252,0.9973042753252,0.9973042753252,
0.9973042753252,0.9973042753252,0.9973042753252,0.9973042753252,0.9973042753252),
(1.008087174024,1.008087174024,1.008087174024,1.008087174024,1.008087174024,
1.008087174024,1.008087174024,1.008087174024,1.008087174024,1.008087174024,
1.008087174024)))
REPRESENTATION_ITEM('')
SURFACE()
);
#154=(
BOUNDED_SURFACE()
B_SPLINE_SURFACE(3,3,((#31889,#31890,#31891,#31892,#31893,#31894,#31895,
#31896,#31897),(#31898,#31899,#31900,#31901,#31902,#31903,#31904,#31905,
#31906),(#31907,#31908,#31909,#31910,#31911,#31912,#31913,#31914,#31915),
(#31916,#31917,#31918,#31919,#31920,#31921,#31922,#31923,#31924)),
 .UNSPECIFIED.,.F.,.F.,.F.)
B_SPLINE_SURFACE_WITH_KNOTS((4,4),(4,1,1,1,1,1,4),(0.,1.),(-0.02991897955271,
0.,0.2239749897618,0.4574668129281,0.7131740843088,1.,1.029884092175),
 .UNSPECIFIED.)
GEOMETRIC_REPRESENTATION_ITEM()
RATIONAL_B_SPLINE_SURFACE(((1.021500558577,1.021500558577,1.021500558577,
1.021500558577,1.021500558577,1.021500558577,1.021500558577,1.021500558577,
1.021500558577),(0.992833147141,0.992833147141,0.992833147141,0.992833147141,
0.992833147141,0.992833147141,0.992833147141,0.992833147141,0.992833147141),
(0.992833147141,0.992833147141,0.992833147141,0.992833147141,0.992833147141,
0.992833147141,0.992833147141,0.992833147141,0.992833147141),(1.021500558577,
1.021500558577,1.021500558577,1.021500558577,1.021500558577,1.021500558577,
1.021500558577,1.021500558577,1.021500558577)))
REPRESENTATION_ITEM('')
SURFACE()
);
#155=(
BOUNDED_SURFACE()
B_SPLINE_SURFACE(3,3,((#31992,#31993,#31994,#31995,#31996,#31997,#31998,
#31999,#32000,#32001,#32002),(#32003,#32004,#32005,#32006,#32007,#32008,
#32009,#32010,#32011,#32012,#32013),(#32014,#32015,#32016,#32017,#32018,
#32019,#32020,#32021,#32022,#32023,#32024),(#32025,#32026,#32027,#32028,
#32029,#32030,#32031,#32032,#32033,#32034,#32035)),.UNSPECIFIED.,.F.,.F.,
 .F.)
B_SPLINE_SURFACE_WITH_KNOTS((4,4),(4,1,1,1,1,1,1,1,4),(0.,1.),(-0.02991442636641,
0.,0.1652192384749,0.3271780455741,0.486578186817,0.6458635561448,0.8144083932013,
1.,1.029876740826),.UNSPECIFIED.)
GEOMETRIC_REPRESENTATION_ITEM()
RATIONAL_B_SPLINE_SURFACE(((1.021500558569,1.021500558569,1.021500558569,
1.021500558569,1.021500558569,1.021500558569,1.021500558569,1.021500558569,
1.021500558569,1.021500558569,1.021500558569),(0.9928331471435,0.9928331471435,
0.9928331471435,0.9928331471435,0.9928331471435,0.9928331471435,0.9928331471435,
0.9928331471435,0.9928331471435,0.9928331471435,0.9928331471435),(0.9928331471435,
0.9928331471435,0.9928331471435,0.9928331471435,0.9928331471435,0.9928331471435,
0.9928331471435,0.9928331471435,0.9928331471435,0.9928331471435,0.9928331471435),
(1.021500558569,1.021500558569,1.021500558569,1.021500558569,1.021500558569,
1.021500558569,1.021500558569,1.021500558569,1.021500558569,1.021500558569,
1.021500558569)))
REPRESENTATION_ITEM('')
SURFACE()
);
#156=(
BOUNDED_SURFACE()
B_SPLINE_SURFACE(3,3,((#32040,#32041,#32042,#32043,#32044,#32045,#32046,
#32047,#32048,#32049,#32050,#32051),(#32052,#32053,#32054,#32055,#32056,
#32057,#32058,#32059,#32060,#32061,#32062,#32063),(#32064,#32065,#32066,
#32067,#32068,#32069,#32070,#32071,#32072,#32073,#32074,#32075),(#32076,
#32077,#32078,#32079,#32080,#32081,#32082,#32083,#32084,#32085,#32086,#32087)),
 .UNSPECIFIED.,.F.,.F.,.F.)
B_SPLINE_SURFACE_WITH_KNOTS((4,4),(4,1,1,1,1,1,1,1,1,4),(0.,1.),(0.0119111100004,
0.111104700859,0.2222213328836,0.3333553389617,0.4444873410571,0.5556025705647,
0.6667268893849,0.7778458691404,0.888938349439,0.9826188152285),
 .UNSPECIFIED.)
GEOMETRIC_REPRESENTATION_ITEM()
RATIONAL_B_SPLINE_SURFACE(((1.211236726733,1.211236726733,1.211236726733,
1.211236726733,1.211236726733,1.211236726733,1.211236726733,1.211236726733,
1.211236726733,1.211236726733,1.211236726733,1.211236726733),(0.9295877577556,
0.9295877577556,0.9295877577556,0.9295877577556,0.9295877577556,0.9295877577556,
0.9295877577556,0.9295877577556,0.9295877577556,0.9295877577556,0.9295877577556,
0.9295877577556),(0.9295877577556,0.9295877577556,0.9295877577556,0.9295877577556,
0.9295877577556,0.9295877577556,0.9295877577556,0.9295877577556,0.9295877577556,
0.9295877577556,0.9295877577556,0.9295877577556),(1.211236726733,1.211236726733,
1.211236726733,1.211236726733,1.211236726733,1.211236726733,1.211236726733,
1.211236726733,1.211236726733,1.211236726733,1.211236726733,1.211236726733)))
REPRESENTATION_ITEM('')
SURFACE()
);
#157=(
BOUNDED_SURFACE()
B_SPLINE_SURFACE(3,3,((#32123,#32124,#32125,#32126,#32127,#32128,#32129,
#32130,#32131),(#32132,#32133,#32134,#32135,#32136,#32137,#32138,#32139,
#32140),(#32141,#32142,#32143,#32144,#32145,#32146,#32147,#32148,#32149),
(#32150,#32151,#32152,#32153,#32154,#32155,#32156,#32157,#32158)),
 .UNSPECIFIED.,.F.,.F.,.F.)
B_SPLINE_SURFACE_WITH_KNOTS((4,4),(4,1,1,1,1,1,4),(0.,1.),(-0.01575975614391,
0.,0.2456294260624,0.4801888085378,0.7270064883701,1.,1.015733967826),
 .UNSPECIFIED.)
GEOMETRIC_REPRESENTATION_ITEM()
RATIONAL_B_SPLINE_SURFACE(((1.201670188537,1.201670188537,1.201670188537,
1.201670188537,1.201670188537,1.201670188537,1.201670188537,1.201670188537,
1.201670188537),(0.9327766038211,0.9327766038211,0.9327766038211,0.9327766038211,
0.9327766038211,0.9327766038211,0.9327766038211,0.9327766038211,0.9327766038211),
(0.9327766038211,0.9327766038211,0.9327766038211,0.9327766038211,0.9327766038211,
0.9327766038211,0.9327766038211,0.9327766038211,0.9327766038211),(1.201670188537,
1.201670188537,1.201670188537,1.201670188537,1.201670188537,1.201670188537,
1.201670188537,1.201670188537,1.201670188537)))
REPRESENTATION_ITEM('')
SURFACE()
);
#158=(
BOUNDED_SURFACE()
B_SPLINE_SURFACE(3,3,((#32368,#32369,#32370,#32371,#32372,#32373,#32374,
#32375),(#32376,#32377,#32378,#32379,#32380,#32381,#32382,#32383),(#32384,
#32385,#32386,#32387,#32388,#32389,#32390,#32391),(#32392,#32393,#32394,
#32395,#32396,#32397,#32398,#32399)),.UNSPECIFIED.,.F.,.F.,.F.)
B_SPLINE_SURFACE_WITH_KNOTS((4,4),(4,1,1,1,1,4),(0.,1.),(-0.02000000006299,
0.,0.3331237554216,0.6664570887615,1.,1.020000003967),.UNSPECIFIED.)
GEOMETRIC_REPRESENTATION_ITEM()
RATIONAL_B_SPLINE_SURFACE(((1.158475807259,1.158475807259,1.158475807259,
1.158475807259,1.158475807259,1.158475807259,1.158475807259,1.158475807259),
(0.9471747309136,0.9471747309136,0.9471747309136,0.9471747309136,0.9471747309136,
0.9471747309136,0.9471747309136,0.9471747309136),(0.9471747309136,0.9471747309136,
0.9471747309136,0.9471747309136,0.9471747309136,0.9471747309136,0.9471747309136,
0.9471747309136),(1.158475807259,1.158475807259,1.158475807259,1.158475807259,
1.158475807259,1.158475807259,1.158475807259,1.158475807259)))
REPRESENTATION_ITEM('')
SURFACE()
);
#159=(
BOUNDED_SURFACE()
B_SPLINE_SURFACE(3,3,((#32407,#32408,#32409,#32410,#32411,#32412,#32413,
#32414),(#32415,#32416,#32417,#32418,#32419,#32420,#32421,#32422),(#32423,
#32424,#32425,#32426,#32427,#32428,#32429,#32430),(#32431,#32432,#32433,
#32434,#32435,#32436,#32437,#32438)),.UNSPECIFIED.,.F.,.F.,.F.)
B_SPLINE_SURFACE_WITH_KNOTS((4,4),(4,1,1,1,1,4),(0.,1.),(-0.02,0.,0.3335430444131,
0.666876377753,1.,1.019999999985),.UNSPECIFIED.)
GEOMETRIC_REPRESENTATION_ITEM()
RATIONAL_B_SPLINE_SURFACE(((1.158475807259,1.158475807259,1.158475807259,
1.158475807259,1.158475807259,1.158475807259,1.158475807259,1.158475807259),
(0.9471747309136,0.9471747309136,0.9471747309136,0.9471747309136,0.9471747309136,
0.9471747309136,0.9471747309136,0.9471747309136),(0.9471747309136,0.9471747309136,
0.9471747309136,0.9471747309136,0.9471747309136,0.9471747309136,0.9471747309136,
0.9471747309136),(1.158475807259,1.158475807259,1.158475807259,1.158475807259,
1.158475807259,1.158475807259,1.158475807259,1.158475807259)))
REPRESENTATION_ITEM('')
SURFACE()
);
#160=(
BOUNDED_SURFACE()
B_SPLINE_SURFACE(3,3,((#32665,#32666,#32667,#32668,#32669,#32670,#32671,
#32672,#32673,#32674),(#32675,#32676,#32677,#32678,#32679,#32680,#32681,
#32682,#32683,#32684),(#32685,#32686,#32687,#32688,#32689,#32690,#32691,
#32692,#32693,#32694),(#32695,#32696,#32697,#32698,#32699,#32700,#32701,
#32702,#32703,#32704)),.UNSPECIFIED.,.F.,.F.,.F.)
B_SPLINE_SURFACE_WITH_KNOTS((4,4),(4,1,1,1,1,1,1,4),(0.,1.),(-0.02782793672778,
0.,0.2061198945833,0.405852717027,0.5969792694224,0.7914070803093,1.,1.028079856947),
 .UNSPECIFIED.)
GEOMETRIC_REPRESENTATION_ITEM()
RATIONAL_B_SPLINE_SURFACE(((1.187634479517,1.187634479517,1.187634479517,
1.187634479517,1.187634479517,1.187634479517,1.187634479517,1.187634479517,
1.187634479517,1.187634479517),(0.9374551734942,0.9374551734942,0.9374551734942,
0.9374551734942,0.9374551734942,0.9374551734942,0.9374551734942,0.9374551734942,
0.9374551734942,0.9374551734942),(0.9374551734942,0.9374551734942,0.9374551734942,
0.9374551734942,0.9374551734942,0.9374551734942,0.9374551734942,0.9374551734942,
0.9374551734942,0.9374551734942),(1.187634479517,1.187634479517,1.187634479517,
1.187634479517,1.187634479517,1.187634479517,1.187634479517,1.187634479517,
1.187634479517,1.187634479517)))
REPRESENTATION_ITEM('')
SURFACE()
);
#161=(
BOUNDED_SURFACE()
B_SPLINE_SURFACE(3,3,((#32793,#32794,#32795,#32796,#32797,#32798,#32799,
#32800,#32801,#32802),(#32803,#32804,#32805,#32806,#32807,#32808,#32809,
#32810,#32811,#32812),(#32813,#32814,#32815,#32816,#32817,#32818,#32819,
#32820,#32821,#32822),(#32823,#32824,#32825,#32826,#32827,#32828,#32829,
#32830,#32831,#32832)),.UNSPECIFIED.,.F.,.F.,.F.)
B_SPLINE_SURFACE_WITH_KNOTS((4,4),(4,1,1,1,1,1,1,4),(0.,1.),(-0.02810083996936,
0.,0.2044929737017,0.4039878177866,0.5954658095825,0.7901158902839,1.,1.027817073056),
 .UNSPECIFIED.)
GEOMETRIC_REPRESENTATION_ITEM()
RATIONAL_B_SPLINE_SURFACE(((1.187634481559,1.187634481559,1.187634481559,
1.187634481559,1.187634481559,1.187634481559,1.187634481559,1.187634481559,
1.187634481559,1.187634481559),(0.9374551728136,0.9374551728136,0.9374551728136,
0.9374551728136,0.9374551728136,0.9374551728136,0.9374551728136,0.9374551728136,
0.9374551728136,0.9374551728136),(0.9374551728136,0.9374551728136,0.9374551728136,
0.9374551728136,0.9374551728136,0.9374551728136,0.9374551728136,0.9374551728136,
0.9374551728136,0.9374551728136),(1.187634481559,1.187634481559,1.187634481559,
1.187634481559,1.187634481559,1.187634481559,1.187634481559,1.187634481559,
1.187634481559,1.187634481559)))
REPRESENTATION_ITEM('')
SURFACE()
);
#162=(
BOUNDED_SURFACE()
B_SPLINE_SURFACE(3,3,((#32835,#32836,#32837,#32838,#32839,#32840,#32841,
#32842),(#32843,#32844,#32845,#32846,#32847,#32848,#32849,#32850),(#32851,
#32852,#32853,#32854,#32855,#32856,#32857,#32858),(#32859,#32860,#32861,
#32862,#32863,#32864,#32865,#32866)),.UNSPECIFIED.,.F.,.F.,.F.)
B_SPLINE_SURFACE_WITH_KNOTS((4,4),(4,1,1,1,1,4),(0.,1.),(-0.001077616544647,
0.,0.0278179355033,0.0559228241955,0.08712239292215,0.1088331409388),
 .UNSPECIFIED.)
GEOMETRIC_REPRESENTATION_ITEM()
RATIONAL_B_SPLINE_SURFACE(((1.199526979016,1.199526979016,1.199526979016,
1.199526979016,1.199526979016,1.199526979016,1.199526979016,1.199526979016),
(0.9334910069946,0.9334910069946,0.9334910069946,0.9334910069946,0.9334910069946,
0.9334910069946,0.9334910069946,0.9334910069946),(0.9334910069946,0.9334910069946,
0.9334910069946,0.9334910069946,0.9334910069946,0.9334910069946,0.9334910069946,
0.9334910069946),(1.199526979016,1.199526979016,1.199526979016,1.199526979016,
1.199526979016,1.199526979016,1.199526979016,1.199526979016)))
REPRESENTATION_ITEM('')
SURFACE()
);
#163=(
BOUNDED_SURFACE()
B_SPLINE_SURFACE(3,3,((#32867,#32868,#32869,#32870,#32871,#32872,#32873,
#32874),(#32875,#32876,#32877,#32878,#32879,#32880,#32881,#32882),(#32883,
#32884,#32885,#32886,#32887,#32888,#32889,#32890),(#32891,#32892,#32893,
#32894,#32895,#32896,#32897,#32898)),.UNSPECIFIED.,.F.,.F.,.F.)
B_SPLINE_SURFACE_WITH_KNOTS((4,4),(4,1,1,1,1,4),(0.,1.),(-0.02,0.,0.3335430447055,
0.6668763780453,1.,1.019999999985),.UNSPECIFIED.)
GEOMETRIC_REPRESENTATION_ITEM()
RATIONAL_B_SPLINE_SURFACE(((1.158475807259,1.158475807259,1.158475807259,
1.158475807259,1.158475807259,1.158475807259,1.158475807259,1.158475807259),
(0.9471747309136,0.9471747309136,0.9471747309136,0.9471747309136,0.9471747309136,
0.9471747309136,0.9471747309136,0.9471747309136),(0.9471747309136,0.9471747309136,
0.9471747309136,0.9471747309136,0.9471747309136,0.9471747309136,0.9471747309136,
0.9471747309136),(1.158475807259,1.158475807259,1.158475807259,1.158475807259,
1.158475807259,1.158475807259,1.158475807259,1.158475807259)))
REPRESENTATION_ITEM('')
SURFACE()
);
#164=(
BOUNDED_SURFACE()
B_SPLINE_SURFACE(3,3,((#32906,#32907,#32908,#32909,#32910,#32911,#32912,
#32913),(#32914,#32915,#32916,#32917,#32918,#32919,#32920,#32921),(#32922,
#32923,#32924,#32925,#32926,#32927,#32928,#32929),(#32930,#32931,#32932,
#32933,#32934,#32935,#32936,#32937)),.UNSPECIFIED.,.F.,.F.,.F.)
B_SPLINE_SURFACE_WITH_KNOTS((4,4),(4,1,1,1,1,4),(0.,1.),(-0.02000000007603,
0.,0.3331237556924,0.6664570890323,1.,1.020000004632),.UNSPECIFIED.)
GEOMETRIC_REPRESENTATION_ITEM()
RATIONAL_B_SPLINE_SURFACE(((1.158475807259,1.158475807259,1.158475807259,
1.158475807259,1.158475807259,1.158475807259,1.158475807259,1.158475807259),
(0.9471747309136,0.9471747309136,0.9471747309136,0.9471747309136,0.9471747309136,
0.9471747309136,0.9471747309136,0.9471747309136),(0.9471747309136,0.9471747309136,
0.9471747309136,0.9471747309136,0.9471747309136,0.9471747309136,0.9471747309136,
0.9471747309136),(1.158475807259,1.158475807259,1.158475807259,1.158475807259,
1.158475807259,1.158475807259,1.158475807259,1.158475807259)))
REPRESENTATION_ITEM('')
SURFACE()
);
#165=(
BOUNDED_SURFACE()
B_SPLINE_SURFACE(3,3,((#32939,#32940,#32941,#32942,#32943,#32944,#32945,
#32946,#32947),(#32948,#32949,#32950,#32951,#32952,#32953,#32954,#32955,
#32956),(#32957,#32958,#32959,#32960,#32961,#32962,#32963,#32964,#32965),
(#32966,#32967,#32968,#32969,#32970,#32971,#32972,#32973,#32974)),
 .UNSPECIFIED.,.F.,.F.,.F.)
B_SPLINE_SURFACE_WITH_KNOTS((4,4),(4,1,1,1,1,1,4),(0.,1.),(-0.03990139320459,
0.,0.2383747185699,0.4794833111693,0.7307955330181,1.,1.039731692604),
 .UNSPECIFIED.)
GEOMETRIC_REPRESENTATION_ITEM()
RATIONAL_B_SPLINE_SURFACE(((1.163827495202,1.163827495202,1.163827495202,
1.163827495202,1.163827495202,1.163827495202,1.163827495202,1.163827495202,
1.163827495202),(0.9453908349325,0.9453908349325,0.9453908349325,0.9453908349325,
0.9453908349325,0.9453908349325,0.9453908349325,0.9453908349325,0.9453908349325),
(0.9453908349325,0.9453908349325,0.9453908349325,0.9453908349325,0.9453908349325,
0.9453908349325,0.9453908349325,0.9453908349325,0.9453908349325),(1.163827495202,
1.163827495202,1.163827495202,1.163827495202,1.163827495202,1.163827495202,
1.163827495202,1.163827495202,1.163827495202)))
REPRESENTATION_ITEM('')
SURFACE()
);
#166=(
BOUNDED_SURFACE()
B_SPLINE_SURFACE(3,3,((#33033,#33034,#33035,#33036,#33037,#33038,#33039,
#33040,#33041),(#33042,#33043,#33044,#33045,#33046,#33047,#33048,#33049,
#33050),(#33051,#33052,#33053,#33054,#33055,#33056,#33057,#33058,#33059),
(#33060,#33061,#33062,#33063,#33064,#33065,#33066,#33067,#33068)),
 .UNSPECIFIED.,.F.,.F.,.F.)
B_SPLINE_SURFACE_WITH_KNOTS((4,4),(4,1,1,1,1,1,4),(0.,1.),(-0.03973821722907,
0.,0.2388826440098,0.4802432095543,0.7314080978693,1.,1.039877733719),
 .UNSPECIFIED.)
GEOMETRIC_REPRESENTATION_ITEM()
RATIONAL_B_SPLINE_SURFACE(((1.163827493612,1.163827493612,1.163827493612,
1.163827493612,1.163827493612,1.163827493612,1.163827493612,1.163827493612,
1.163827493612),(0.9453908354627,0.9453908354627,0.9453908354627,0.9453908354627,
0.9453908354627,0.9453908354627,0.9453908354627,0.9453908354627,0.9453908354627),
(0.9453908354627,0.9453908354627,0.9453908354627,0.9453908354627,0.9453908354627,
0.9453908354627,0.9453908354627,0.9453908354627,0.9453908354627),(1.163827493612,
1.163827493612,1.163827493612,1.163827493612,1.163827493612,1.163827493612,
1.163827493612,1.163827493612,1.163827493612)))
REPRESENTATION_ITEM('')
SURFACE()
);
#167=(
BOUNDED_SURFACE()
B_SPLINE_SURFACE(3,3,((#33070,#33071,#33072,#33073,#33074,#33075,#33076,
#33077,#33078,#33079,#33080,#33081,#33082,#33083,#33084,#33085,#33086,#33087,
#33088,#33089,#33090,#33091,#33092,#33093,#33094,#33095,#33096,#33097,#33098,
#33099,#33100,#33101),(#33102,#33103,#33104,#33105,#33106,#33107,#33108,
#33109,#33110,#33111,#33112,#33113,#33114,#33115,#33116,#33117,#33118,#33119,
#33120,#33121,#33122,#33123,#33124,#33125,#33126,#33127,#33128,#33129,#33130,
#33131,#33132,#33133),(#33134,#33135,#33136,#33137,#33138,#33139,#33140,
#33141,#33142,#33143,#33144,#33145,#33146,#33147,#33148,#33149,#33150,#33151,
#33152,#33153,#33154,#33155,#33156,#33157,#33158,#33159,#33160,#33161,#33162,
#33163,#33164,#33165),(#33166,#33167,#33168,#33169,#33170,#33171,#33172,
#33173,#33174,#33175,#33176,#33177,#33178,#33179,#33180,#33181,#33182,#33183,
#33184,#33185,#33186,#33187,#33188,#33189,#33190,#33191,#33192,#33193,#33194,
#33195,#33196,#33197)),.UNSPECIFIED.,.F.,.F.,.F.)
B_SPLINE_SURFACE_WITH_KNOTS((4,4),(4,1,1,1,1,1,1,1,1,1,1,1,1,1,1,1,1,1,
1,1,1,1,1,1,1,1,1,1,1,4),(0.,1.),(-0.009989617270159,0.,0.0587369296208,
0.111068550249,0.1581000808001,0.2003396839717,0.2384448290796,0.2747221985793,
0.3117544904028,0.3494937277553,0.3869465899255,0.4242215507061,0.4615931261968,
0.499066395259,0.5364199609172,0.5733902772176,0.6100694635878,0.6464467903499,
0.6809974474155,0.7120024196009,0.7411742705344,0.7707771184994,0.8006196344549,
0.8302940356761,0.8602243035839,0.8909644083677,0.9237463930732,0.9597502743101,
1.,1.009989117017),.UNSPECIFIED.)
GEOMETRIC_REPRESENTATION_ITEM()
RATIONAL_B_SPLINE_SURFACE(((1.192397230944,1.192397230944,1.192397230944,
1.192397230944,1.192397230944,1.192397230944,1.192397230944,1.192397230944,
1.192397230944,1.192397230944,1.192397230944,1.192397230944,1.192397230944,
1.192397230944,1.192397230944,1.192397230944,1.192397230944,1.192397230944,
1.192397230944,1.192397230944,1.192397230944,1.192397230944,1.192397230944,
1.192397230944,1.192397230944,1.192397230944,1.192397230944,1.192397230944,
1.192397230944,1.192397230944,1.192397230944,1.192397230944),(0.9358675896855,
0.9358675896855,0.9358675896855,0.9358675896855,0.9358675896855,0.9358675896855,
0.9358675896855,0.9358675896855,0.9358675896855,0.9358675896855,0.9358675896855,
0.9358675896855,0.9358675896855,0.9358675896855,0.9358675896855,0.9358675896855,
0.9358675896855,0.9358675896855,0.9358675896855,0.9358675896855,0.9358675896855,
0.9358675896855,0.9358675896855,0.9358675896855,0.9358675896855,0.9358675896855,
0.9358675896855,0.9358675896855,0.9358675896855,0.9358675896855,0.9358675896855,
0.9358675896855),(0.9358675896855,0.9358675896855,0.9358675896855,0.9358675896855,
0.9358675896855,0.9358675896855,0.9358675896855,0.9358675896855,0.9358675896855,
0.9358675896855,0.9358675896855,0.9358675896855,0.9358675896855,0.9358675896855,
0.9358675896855,0.9358675896855,0.9358675896855,0.9358675896855,0.9358675896855,
0.9358675896855,0.9358675896855,0.9358675896855,0.9358675896855,0.9358675896855,
0.9358675896855,0.9358675896855,0.9358675896855,0.9358675896855,0.9358675896855,
0.9358675896855,0.9358675896855,0.9358675896855),(1.192397230944,1.192397230944,
1.192397230944,1.192397230944,1.192397230944,1.192397230944,1.192397230944,
1.192397230944,1.192397230944,1.192397230944,1.192397230944,1.192397230944,
1.192397230944,1.192397230944,1.192397230944,1.192397230944,1.192397230944,
1.192397230944,1.192397230944,1.192397230944,1.192397230944,1.192397230944,
1.192397230944,1.192397230944,1.192397230944,1.192397230944,1.192397230944,
1.192397230944,1.192397230944,1.192397230944,1.192397230944,1.192397230944)))
REPRESENTATION_ITEM('')
SURFACE()
);
#168=(
BOUNDED_SURFACE()
B_SPLINE_SURFACE(3,3,((#33666,#33667,#33668,#33669,#33670,#33671,#33672,
#33673,#33674,#33675,#33676,#33677,#33678,#33679,#33680,#33681,#33682,#33683,
#33684,#33685,#33686,#33687,#33688,#33689,#33690,#33691,#33692,#33693,#33694,
#33695,#33696,#33697),(#33698,#33699,#33700,#33701,#33702,#33703,#33704,
#33705,#33706,#33707,#33708,#33709,#33710,#33711,#33712,#33713,#33714,#33715,
#33716,#33717,#33718,#33719,#33720,#33721,#33722,#33723,#33724,#33725,#33726,
#33727,#33728,#33729),(#33730,#33731,#33732,#33733,#33734,#33735,#33736,
#33737,#33738,#33739,#33740,#33741,#33742,#33743,#33744,#33745,#33746,#33747,
#33748,#33749,#33750,#33751,#33752,#33753,#33754,#33755,#33756,#33757,#33758,
#33759,#33760,#33761),(#33762,#33763,#33764,#33765,#33766,#33767,#33768,
#33769,#33770,#33771,#33772,#33773,#33774,#33775,#33776,#33777,#33778,#33779,
#33780,#33781,#33782,#33783,#33784,#33785,#33786,#33787,#33788,#33789,#33790,
#33791,#33792,#33793)),.UNSPECIFIED.,.F.,.F.,.F.)
B_SPLINE_SURFACE_WITH_KNOTS((4,4),(4,1,1,1,1,1,1,1,1,1,1,1,1,1,1,1,1,1,
1,1,1,1,1,1,1,1,1,1,1,4),(0.,1.),(-0.009989616921005,0.,0.05872646932563,
0.1110508073303,0.1580780876269,0.2003155443802,0.2384155963746,0.2746745689611,
0.3116781024864,0.3493943002845,0.3868271443784,0.4240772685742,0.4614186760705,
0.4988604389596,0.5361879081759,0.5731414127621,0.6098108086259,0.6461939396313,
0.6807803323384,0.7118281019108,0.7410274548133,0.7706525155955,0.8005231162647,
0.8302238307092,0.8601755167066,0.89093194483,0.9237248042115,0.9597384770757,
1.,1.009989116574),.UNSPECIFIED.)
GEOMETRIC_REPRESENTATION_ITEM()
RATIONAL_B_SPLINE_SURFACE(((1.192397251387,1.192397251387,1.192397251387,
1.192397251387,1.192397251387,1.192397251387,1.192397251387,1.192397251387,
1.192397251387,1.192397251387,1.192397251387,1.192397251387,1.192397251387,
1.192397251387,1.192397251387,1.192397251387,1.192397251387,1.192397251387,
1.192397251387,1.192397251387,1.192397251387,1.192397251387,1.192397251387,
1.192397251387,1.192397251387,1.192397251387,1.192397251387,1.192397251387,
1.192397251387,1.192397251387,1.192397251387,1.192397251387),(0.935867582871,
0.935867582871,0.935867582871,0.935867582871,0.935867582871,0.935867582871,
0.935867582871,0.935867582871,0.935867582871,0.935867582871,0.935867582871,
0.935867582871,0.935867582871,0.935867582871,0.935867582871,0.935867582871,
0.935867582871,0.935867582871,0.935867582871,0.935867582871,0.935867582871,
0.935867582871,0.935867582871,0.935867582871,0.935867582871,0.935867582871,
0.935867582871,0.935867582871,0.935867582871,0.935867582871,0.935867582871,
0.935867582871),(0.935867582871,0.935867582871,0.935867582871,0.935867582871,
0.935867582871,0.935867582871,0.935867582871,0.935867582871,0.935867582871,
0.935867582871,0.935867582871,0.935867582871,0.935867582871,0.935867582871,
0.935867582871,0.935867582871,0.935867582871,0.935867582871,0.935867582871,
0.935867582871,0.935867582871,0.935867582871,0.935867582871,0.935867582871,
0.935867582871,0.935867582871,0.935867582871,0.935867582871,0.935867582871,
0.935867582871,0.935867582871,0.935867582871),(1.192397251387,1.192397251387,
1.192397251387,1.192397251387,1.192397251387,1.192397251387,1.192397251387,
1.192397251387,1.192397251387,1.192397251387,1.192397251387,1.192397251387,
1.192397251387,1.192397251387,1.192397251387,1.192397251387,1.192397251387,
1.192397251387,1.192397251387,1.192397251387,1.192397251387,1.192397251387,
1.192397251387,1.192397251387,1.192397251387,1.192397251387,1.192397251387,
1.192397251387,1.192397251387,1.192397251387,1.192397251387,1.192397251387)))
REPRESENTATION_ITEM('')
SURFACE()
);
#169=(
BOUNDED_SURFACE()
B_SPLINE_SURFACE(3,3,((#33795,#33796,#33797,#33798,#33799,#33800,#33801,
#33802,#33803),(#33804,#33805,#33806,#33807,#33808,#33809,#33810,#33811,
#33812),(#33813,#33814,#33815,#33816,#33817,#33818,#33819,#33820,#33821),
(#33822,#33823,#33824,#33825,#33826,#33827,#33828,#33829,#33830)),
 .UNSPECIFIED.,.F.,.F.,.F.)
B_SPLINE_SURFACE_WITH_KNOTS((4,4),(4,1,1,1,1,1,4),(0.,1.),(-0.03973820027638,
0.,0.238622357915,0.4800568473432,0.731387517944,1.,1.03987771478),
 .UNSPECIFIED.)
GEOMETRIC_REPRESENTATION_ITEM()
RATIONAL_B_SPLINE_SURFACE(((1.163827493602,1.163827493602,1.163827493602,
1.163827493602,1.163827493602,1.163827493602,1.163827493602,1.163827493602,
1.163827493602),(0.9453908354662,0.9453908354662,0.9453908354662,0.9453908354662,
0.9453908354662,0.9453908354662,0.9453908354662,0.9453908354662,0.9453908354662),
(0.9453908354662,0.9453908354662,0.9453908354662,0.9453908354662,0.9453908354662,
0.9453908354662,0.9453908354662,0.9453908354662,0.9453908354662),(1.163827493602,
1.163827493602,1.163827493602,1.163827493602,1.163827493602,1.163827493602,
1.163827493602,1.163827493602,1.163827493602)))
REPRESENTATION_ITEM('')
SURFACE()
);
#170=(
BOUNDED_SURFACE()
B_SPLINE_SURFACE(3,3,((#33888,#33889,#33890,#33891,#33892,#33893,#33894,
#33895,#33896),(#33897,#33898,#33899,#33900,#33901,#33902,#33903,#33904,
#33905),(#33906,#33907,#33908,#33909,#33910,#33911,#33912,#33913,#33914),
(#33915,#33916,#33917,#33918,#33919,#33920,#33921,#33922,#33923)),
 .UNSPECIFIED.,.F.,.F.,.F.)
B_SPLINE_SURFACE_WITH_KNOTS((4,4),(4,1,1,1,1,1,4),(0.,1.),(-0.03990137353967,
0.,0.2386413019669,0.4796774710128,0.7308215928377,1.,1.039731675547),
 .UNSPECIFIED.)
GEOMETRIC_REPRESENTATION_ITEM()
RATIONAL_B_SPLINE_SURFACE(((1.163827495208,1.163827495208,1.163827495208,
1.163827495208,1.163827495208,1.163827495208,1.163827495208,1.163827495208,
1.163827495208),(0.9453908349308,0.9453908349308,0.9453908349308,0.9453908349308,
0.9453908349308,0.9453908349308,0.9453908349308,0.9453908349308,0.9453908349308),
(0.9453908349308,0.9453908349308,0.9453908349308,0.9453908349308,0.9453908349308,
0.9453908349308,0.9453908349308,0.9453908349308,0.9453908349308),(1.163827495208,
1.163827495208,1.163827495208,1.163827495208,1.163827495208,1.163827495208,
1.163827495208,1.163827495208,1.163827495208)))
REPRESENTATION_ITEM('')
SURFACE()
);
#171=(
BOUNDED_SURFACE()
B_SPLINE_SURFACE(3,3,((#33924,#33925,#33926,#33927,#33928,#33929,#33930,
#33931,#33932,#33933),(#33934,#33935,#33936,#33937,#33938,#33939,#33940,
#33941,#33942,#33943),(#33944,#33945,#33946,#33947,#33948,#33949,#33950,
#33951,#33952,#33953),(#33954,#33955,#33956,#33957,#33958,#33959,#33960,
#33961,#33962,#33963)),.UNSPECIFIED.,.F.,.F.,.F.)
B_SPLINE_SURFACE_WITH_KNOTS((4,4),(4,1,1,1,1,1,1,4),(0.,1.),(0.03540281776569,
0.1234679415063,0.2632035734038,0.4203296727887,0.5957836491349,0.789268501371,
1.,1.00911688994),.UNSPECIFIED.)
GEOMETRIC_REPRESENTATION_ITEM()
RATIONAL_B_SPLINE_SURFACE(((1.211236248281,1.211236248281,1.211236248281,
1.211236248281,1.211236248281,1.211236248281,1.211236248281,1.211236248281,
1.211236248281,1.211236248281),(0.9295879172397,0.9295879172397,0.9295879172397,
0.9295879172397,0.9295879172397,0.9295879172397,0.9295879172397,0.9295879172397,
0.9295879172397,0.9295879172397),(0.9295879172397,0.9295879172397,0.9295879172397,
0.9295879172397,0.9295879172397,0.9295879172397,0.9295879172397,0.9295879172397,
0.9295879172397,0.9295879172397),(1.211236248281,1.211236248281,1.211236248281,
1.211236248281,1.211236248281,1.211236248281,1.211236248281,1.211236248281,
1.211236248281,1.211236248281)))
REPRESENTATION_ITEM('')
SURFACE()
);
#172=(
BOUNDED_SURFACE()
B_SPLINE_SURFACE(3,3,((#34041,#34042,#34043,#34044,#34045,#34046,#34047,
#34048,#34049,#34050,#34051,#34052,#34053,#34054,#34055,#34056,#34057,#34058,
#34059),(#34060,#34061,#34062,#34063,#34064,#34065,#34066,#34067,#34068,
#34069,#34070,#34071,#34072,#34073,#34074,#34075,#34076,#34077,#34078),
(#34079,#34080,#34081,#34082,#34083,#34084,#34085,#34086,#34087,#34088,
#34089,#34090,#34091,#34092,#34093,#34094,#34095,#34096,#34097),(#34098,
#34099,#34100,#34101,#34102,#34103,#34104,#34105,#34106,#34107,#34108,#34109,
#34110,#34111,#34112,#34113,#34114,#34115,#34116)),.UNSPECIFIED.,.F.,.F.,
 .F.)
B_SPLINE_SURFACE_WITH_KNOTS((4,4),(4,1,1,1,1,1,1,1,1,1,1,1,1,1,1,1,4),(0.,
1.),(-0.01076426746053,0.,0.04152389901166,0.08394379225387,0.1302342687654,
0.1804523447143,0.2349355052966,0.2939338029969,0.3580057487009,0.4275129366519,
0.5025423241297,0.5839356639565,0.6731830882238,0.7717942958468,0.8805575045219,
1.,1.009808133051),.UNSPECIFIED.)
GEOMETRIC_REPRESENTATION_ITEM()
RATIONAL_B_SPLINE_SURFACE(((1.088372924818,1.088372924818,1.088372924818,
1.088372924818,1.088372924818,1.088372924818,1.088372924818,1.088372924818,
1.088372924818,1.088372924818,1.088372924818,1.088372924818,1.088372924818,
1.088372924818,1.088372924818,1.088372924818,1.088372924818,1.088372924818,
1.088372924818),(0.9705423583942,0.9705423583942,0.9705423583942,0.9705423583942,
0.9705423583942,0.9705423583942,0.9705423583942,0.9705423583942,0.9705423583942,
0.9705423583942,0.9705423583942,0.9705423583942,0.9705423583942,0.9705423583942,
0.9705423583942,0.9705423583942,0.9705423583942,0.9705423583942,0.9705423583942),
(0.9705423583942,0.9705423583942,0.9705423583942,0.9705423583942,0.9705423583942,
0.9705423583942,0.9705423583942,0.9705423583942,0.9705423583942,0.9705423583942,
0.9705423583942,0.9705423583942,0.9705423583942,0.9705423583942,0.9705423583942,
0.9705423583942,0.9705423583942,0.9705423583942,0.9705423583942),(1.088372924818,
1.088372924818,1.088372924818,1.088372924818,1.088372924818,1.088372924818,
1.088372924818,1.088372924818,1.088372924818,1.088372924818,1.088372924818,
1.088372924818,1.088372924818,1.088372924818,1.088372924818,1.088372924818,
1.088372924818,1.088372924818,1.088372924818)))
REPRESENTATION_ITEM('')
SURFACE()
);
#173=(
BOUNDED_SURFACE()
B_SPLINE_SURFACE(3,3,((#34117,#34118,#34119,#34120,#34121,#34122,#34123,
#34124,#34125,#34126,#34127,#34128),(#34129,#34130,#34131,#34132,#34133,
#34134,#34135,#34136,#34137,#34138,#34139,#34140),(#34141,#34142,#34143,
#34144,#34145,#34146,#34147,#34148,#34149,#34150,#34151,#34152),(#34153,
#34154,#34155,#34156,#34157,#34158,#34159,#34160,#34161,#34162,#34163,#34164)),
 .UNSPECIFIED.,.F.,.F.,.F.)
B_SPLINE_SURFACE_WITH_KNOTS((4,4),(4,1,1,1,1,1,1,1,1,4),(0.,1.),(-0.152618011925,
0.,0.1440925301842,0.2801219903658,0.4114391594101,0.5434056701778,0.6832645286048,
0.8346596058642,1.,1.152833582056),.UNSPECIFIED.)
GEOMETRIC_REPRESENTATION_ITEM()
RATIONAL_B_SPLINE_SURFACE(((1.000094023891,1.000094023891,1.000094023891,
1.000094023891,1.000094023891,1.000094023891,1.000094023891,1.000094023891,
1.000094023891,1.000094023891,1.000094023891,1.000094023891),(0.9999686587029,
0.9999686587029,0.9999686587029,0.9999686587029,0.9999686587029,0.9999686587029,
0.9999686587029,0.9999686587029,0.9999686587029,0.9999686587029,0.9999686587029,
0.9999686587029),(0.9999686587029,0.9999686587029,0.9999686587029,0.9999686587029,
0.9999686587029,0.9999686587029,0.9999686587029,0.9999686587029,0.9999686587029,
0.9999686587029,0.9999686587029,0.9999686587029),(1.000094023891,1.000094023891,
1.000094023891,1.000094023891,1.000094023891,1.000094023891,1.000094023891,
1.000094023891,1.000094023891,1.000094023891,1.000094023891,1.000094023891)))
REPRESENTATION_ITEM('')
SURFACE()
);
#174=(
BOUNDED_SURFACE()
B_SPLINE_SURFACE(3,3,((#34166,#34167,#34168,#34169,#34170,#34171,#34172,
#34173,#34174,#34175),(#34176,#34177,#34178,#34179,#34180,#34181,#34182,
#34183,#34184,#34185),(#34186,#34187,#34188,#34189,#34190,#34191,#34192,
#34193,#34194,#34195),(#34196,#34197,#34198,#34199,#34200,#34201,#34202,
#34203,#34204,#34205)),.UNSPECIFIED.,.F.,.F.,.F.)
B_SPLINE_SURFACE_WITH_KNOTS((4,4),(4,1,1,1,1,1,1,4),(0.,1.),(-0.009053405764054,
0.,0.2128253131466,0.4067103404652,0.5817418357977,0.7383188923361,0.8773475428248,
0.9585687317144),.UNSPECIFIED.)
GEOMETRIC_REPRESENTATION_ITEM()
RATIONAL_B_SPLINE_SURFACE(((1.211237524847,1.211237524847,1.211237524847,
1.211237524847,1.211237524847,1.211237524847,1.211237524847,1.211237524847,
1.211237524847,1.211237524847),(0.9295874917176,0.9295874917176,0.9295874917176,
0.9295874917176,0.9295874917176,0.9295874917176,0.9295874917176,0.9295874917176,
0.9295874917176,0.9295874917176),(0.9295874917176,0.9295874917176,0.9295874917176,
0.9295874917176,0.9295874917176,0.9295874917176,0.9295874917176,0.9295874917176,
0.9295874917176,0.9295874917176),(1.211237524847,1.211237524847,1.211237524847,
1.211237524847,1.211237524847,1.211237524847,1.211237524847,1.211237524847,
1.211237524847,1.211237524847)))
REPRESENTATION_ITEM('')
SURFACE()
);
#175=(
BOUNDED_SURFACE()
B_SPLINE_SURFACE(3,3,((#34282,#34283,#34284,#34285,#34286,#34287,#34288,
#34289,#34290,#34291,#34292,#34293,#34294,#34295,#34296,#34297,#34298,#34299),
(#34300,#34301,#34302,#34303,#34304,#34305,#34306,#34307,#34308,#34309,
#34310,#34311,#34312,#34313,#34314,#34315,#34316,#34317),(#34318,#34319,
#34320,#34321,#34322,#34323,#34324,#34325,#34326,#34327,#34328,#34329,#34330,
#34331,#34332,#34333,#34334,#34335),(#34336,#34337,#34338,#34339,#34340,
#34341,#34342,#34343,#34344,#34345,#34346,#34347,#34348,#34349,#34350,#34351,
#34352,#34353)),.UNSPECIFIED.,.F.,.F.,.F.)
B_SPLINE_SURFACE_WITH_KNOTS((4,4),(4,1,1,1,1,1,1,1,1,1,1,1,1,1,1,4),(0.,
1.),(-0.009797090891202,0.,0.1252864769222,0.2381332273333,0.3395214867139,
0.4311702756169,0.5147945964105,0.5913458810972,0.6613379006761,0.7254151205055,
0.7843391271186,0.8380935847805,0.8886737238581,0.9411160876025,1.,1.010696795736),
 .UNSPECIFIED.)
GEOMETRIC_REPRESENTATION_ITEM()
RATIONAL_B_SPLINE_SURFACE(((1.088374512803,1.088374512803,1.088374512803,
1.088374512803,1.088374512803,1.088374512803,1.088374512803,1.088374512803,
1.088374512803,1.088374512803,1.088374512803,1.088374512803,1.088374512803,
1.088374512803,1.088374512803,1.088374512803,1.088374512803,1.088374512803),
(0.9705418290655,0.9705418290655,0.9705418290655,0.9705418290655,0.9705418290655,
0.9705418290655,0.9705418290655,0.9705418290655,0.9705418290655,0.9705418290655,
0.9705418290655,0.9705418290655,0.9705418290655,0.9705418290655,0.9705418290655,
0.9705418290655,0.9705418290655,0.9705418290655),(0.9705418290655,0.9705418290655,
0.9705418290655,0.9705418290655,0.9705418290655,0.9705418290655,0.9705418290655,
0.9705418290655,0.9705418290655,0.9705418290655,0.9705418290655,0.9705418290655,
0.9705418290655,0.9705418290655,0.9705418290655,0.9705418290655,0.9705418290655,
0.9705418290655),(1.088374512803,1.088374512803,1.088374512803,1.088374512803,
1.088374512803,1.088374512803,1.088374512803,1.088374512803,1.088374512803,
1.088374512803,1.088374512803,1.088374512803,1.088374512803,1.088374512803,
1.088374512803,1.088374512803,1.088374512803,1.088374512803)))
REPRESENTATION_ITEM('')
SURFACE()
);
#176=(
BOUNDED_SURFACE()
B_SPLINE_SURFACE(3,3,((#34354,#34355,#34356,#34357,#34358,#34359,#34360,
#34361,#34362,#34363,#34364),(#34365,#34366,#34367,#34368,#34369,#34370,
#34371,#34372,#34373,#34374,#34375),(#34376,#34377,#34378,#34379,#34380,
#34381,#34382,#34383,#34384,#34385,#34386),(#34387,#34388,#34389,#34390,
#34391,#34392,#34393,#34394,#34395,#34396,#34397)),.UNSPECIFIED.,.F.,.F.,
 .F.)
B_SPLINE_SURFACE_WITH_KNOTS((4,4),(4,1,1,1,1,1,1,1,4),(0.,1.),(-0.04050719629992,
0.,0.2121825428154,0.403201234845,0.5756502932434,0.7316337186034,0.8727661988069,
1.,1.048418925808),.UNSPECIFIED.)
GEOMETRIC_REPRESENTATION_ITEM()
RATIONAL_B_SPLINE_SURFACE(((1.008087784168,1.008087784168,1.008087784168,
1.008087784168,1.008087784168,1.008087784168,1.008087784168,1.008087784168,
1.008087784168,1.008087784168,1.008087784168),(0.997304071944,0.997304071944,
0.997304071944,0.997304071944,0.997304071944,0.997304071944,0.997304071944,
0.997304071944,0.997304071944,0.997304071944,0.997304071944),(0.997304071944,
0.997304071944,0.997304071944,0.997304071944,0.997304071944,0.997304071944,
0.997304071944,0.997304071944,0.997304071944,0.997304071944,0.997304071944),
(1.008087784168,1.008087784168,1.008087784168,1.008087784168,1.008087784168,
1.008087784168,1.008087784168,1.008087784168,1.008087784168,1.008087784168,
1.008087784168)))
REPRESENTATION_ITEM('')
SURFACE()
);
#177=(
BOUNDED_SURFACE()
B_SPLINE_SURFACE(3,3,((#34432,#34433,#34434,#34435,#34436,#34437,#34438),
(#34439,#34440,#34441,#34442,#34443,#34444,#34445),(#34446,#34447,#34448,
#34449,#34450,#34451,#34452),(#34453,#34454,#34455,#34456,#34457,#34458,
#34459)),.UNSPECIFIED.,.F.,.F.,.F.)
B_SPLINE_SURFACE_WITH_KNOTS((4,4),(4,1,1,1,4),(0.,1.),(-0.02191865670977,
0.,0.3711108308406,0.7030029886383,0.86664181477),.UNSPECIFIED.)
GEOMETRIC_REPRESENTATION_ITEM()
RATIONAL_B_SPLINE_SURFACE(((1.201671391236,1.201671391236,1.201671391236,
1.201671391236,1.201671391236,1.201671391236,1.201671391236),(0.9327762029212,
0.9327762029212,0.9327762029212,0.9327762029212,0.9327762029212,0.9327762029212,
0.9327762029212),(0.9327762029212,0.9327762029212,0.9327762029212,0.9327762029212,
0.9327762029212,0.9327762029212,0.9327762029212),(1.201671391236,1.201671391236,
1.201671391236,1.201671391236,1.201671391236,1.201671391236,1.201671391236)))
REPRESENTATION_ITEM('')
SURFACE()
);
#178=(
BOUNDED_SURFACE()
B_SPLINE_SURFACE(3,3,((#34461,#34462,#34463,#34464,#34465,#34466,#34467,
#34468),(#34469,#34470,#34471,#34472,#34473,#34474,#34475,#34476),(#34477,
#34478,#34479,#34480,#34481,#34482,#34483,#34484),(#34485,#34486,#34487,
#34488,#34489,#34490,#34491,#34492)),.UNSPECIFIED.,.F.,.F.,.F.)
B_SPLINE_SURFACE_WITH_KNOTS((4,4),(4,1,1,1,1,4),(0.,1.),(-0.01121526815079,
0.,0.3190669955162,0.6396376709117,1.,1.01119406465),.UNSPECIFIED.)
GEOMETRIC_REPRESENTATION_ITEM()
RATIONAL_B_SPLINE_SURFACE(((1.095350229537,1.095350229537,1.095350229537,
1.095350229537,1.095350229537,1.095350229537,1.095350229537,1.095350229537),
(0.9682165901542,0.9682165901542,0.9682165901542,0.9682165901542,0.9682165901542,
0.9682165901542,0.9682165901542,0.9682165901542),(0.9682165901542,0.9682165901542,
0.9682165901542,0.9682165901542,0.9682165901542,0.9682165901542,0.9682165901542,
0.9682165901542),(1.095350229537,1.095350229537,1.095350229537,1.095350229537,
1.095350229537,1.095350229537,1.095350229537,1.095350229537)))
REPRESENTATION_ITEM('')
SURFACE()
);
#179=(
BOUNDED_SURFACE()
B_SPLINE_SURFACE(3,3,((#34494,#34495,#34496,#34497,#34498,#34499,#34500,
#34501),(#34502,#34503,#34504,#34505,#34506,#34507,#34508,#34509),(#34510,
#34511,#34512,#34513,#34514,#34515,#34516,#34517),(#34518,#34519,#34520,
#34521,#34522,#34523,#34524,#34525)),.UNSPECIFIED.,.F.,.F.,.F.)
B_SPLINE_SURFACE_WITH_KNOTS((4,4),(4,1,1,1,1,4),(0.,1.),(-0.01123151971552,
0.,0.3226324635879,0.6411683732307,1.,1.011214131133),.UNSPECIFIED.)
GEOMETRIC_REPRESENTATION_ITEM()
RATIONAL_B_SPLINE_SURFACE(((1.095350237893,1.095350237893,1.095350237893,
1.095350237893,1.095350237893,1.095350237893,1.095350237893,1.095350237893),
(0.9682165873689,0.9682165873689,0.9682165873689,0.9682165873689,0.9682165873689,
0.9682165873689,0.9682165873689,0.9682165873689),(0.9682165873689,0.9682165873689,
0.9682165873689,0.9682165873689,0.9682165873689,0.9682165873689,0.9682165873689,
0.9682165873689),(1.095350237893,1.095350237893,1.095350237893,1.095350237893,
1.095350237893,1.095350237893,1.095350237893,1.095350237893)))
REPRESENTATION_ITEM('')
SURFACE()
);
#202=CONICAL_SURFACE('',#9881,49.77255842762,0.0349065850398866);
#203=CONICAL_SURFACE('',#9886,49.77255839012,0.0349065850398866);
#204=CONICAL_SURFACE('',#9904,1.925,0.785398163397448);
#210=TOROIDAL_SURFACE('',#9799,4.3,0.5);
#211=TOROIDAL_SURFACE('',#9804,49.4822348431,0.5);
#212=TOROIDAL_SURFACE('',#9832,49.4822348431,0.5);
#213=TOROIDAL_SURFACE('',#9848,49.4822348431,0.5);
#214=TOROIDAL_SURFACE('',#9853,4.3,0.5);
#215=TOROIDAL_SURFACE('',#9863,4.3,0.5);
#216=TOROIDAL_SURFACE('',#9865,3.3,0.5);
#217=TOROIDAL_SURFACE('',#9869,4.3,0.5);
#218=TOROIDAL_SURFACE('',#9879,49.4822348431,0.5);
#237=SHAPE_REPRESENTATION_RELATIONSHIP('SRR','None',#52216,#250);
#250=ADVANCED_BREP_SHAPE_REPRESENTATION('',(#276),#52156);
#263=STYLED_ITEM('',(#52318),#276);
#276=MANIFOLD_SOLID_BREP('Body1',#9123);
#300=FACE_BOUND('',#1400,.T.);
#301=FACE_BOUND('',#1406,.T.);
#302=FACE_BOUND('',#1409,.T.);
#458=PLANE('',#9777);
#459=PLANE('',#9783);
#460=PLANE('',#9786);
#461=PLANE('',#9789);
#462=PLANE('',#9792);
#463=PLANE('',#9812);
#464=PLANE('',#9884);
#465=PLANE('',#9892);
#466=PLANE('',#9909);
#467=PLANE('',#9913);
#781=FACE_OUTER_BOUND('',#1330,.T.);
#782=FACE_OUTER_BOUND('',#1331,.T.);
#783=FACE_OUTER_BOUND('',#1332,.T.);
#784=FACE_OUTER_BOUND('',#1333,.T.);
#785=FACE_OUTER_BOUND('',#1334,.T.);
#786=FACE_OUTER_BOUND('',#1335,.T.);
#787=FACE_OUTER_BOUND('',#1336,.T.);
#788=FACE_OUTER_BOUND('',#1337,.T.);
#789=FACE_OUTER_BOUND('',#1338,.T.);
#790=FACE_OUTER_BOUND('',#1339,.T.);
#791=FACE_OUTER_BOUND('',#1340,.T.);
#792=FACE_OUTER_BOUND('',#1341,.T.);
#793=FACE_OUTER_BOUND('',#1342,.T.);
#794=FACE_OUTER_BOUND('',#1343,.T.);
#795=FACE_OUTER_BOUND('',#1344,.T.);
#796=FACE_OUTER_BOUND('',#1345,.T.);
#797=FACE_OUTER_BOUND('',#1346,.T.);
#798=FACE_OUTER_BOUND('',#1347,.T.);
#799=FACE_OUTER_BOUND('',#1348,.T.);
#800=FACE_OUTER_BOUND('',#1349,.T.);
#801=FACE_OUTER_BOUND('',#1350,.T.);
#802=FACE_OUTER_BOUND('',#1351,.T.);
#803=FACE_OUTER_BOUND('',#1352,.T.);
#804=FACE_OUTER_BOUND('',#1353,.T.);
#805=FACE_OUTER_BOUND('',#1354,.T.);
#806=FACE_OUTER_BOUND('',#1355,.T.);
#807=FACE_OUTER_BOUND('',#1356,.T.);
#808=FACE_OUTER_BOUND('',#1357,.T.);
#809=FACE_OUTER_BOUND('',#1358,.T.);
#810=FACE_OUTER_BOUND('',#1359,.T.);
#811=FACE_OUTER_BOUND('',#1360,.T.);
#812=FACE_OUTER_BOUND('',#1361,.T.);
#813=FACE_OUTER_BOUND('',#1362,.T.);
#814=FACE_OUTER_BOUND('',#1363,.T.);
#815=FACE_OUTER_BOUND('',#1364,.T.);
#816=FACE_OUTER_BOUND('',#1365,.T.);
#817=FACE_OUTER_BOUND('',#1366,.T.);
#818=FACE_OUTER_BOUND('',#1367,.T.);
#819=FACE_OUTER_BOUND('',#1368,.T.);
#820=FACE_OUTER_BOUND('',#1369,.T.);
#821=FACE_OUTER_BOUND('',#1370,.T.);
#822=FACE_OUTER_BOUND('',#1371,.T.);
#823=FACE_OUTER_BOUND('',#1372,.T.);
#824=FACE_OUTER_BOUND('',#1373,.T.);
#825=FACE_OUTER_BOUND('',#1374,.T.);
#826=FACE_OUTER_BOUND('',#1375,.T.);
#827=FACE_OUTER_BOUND('',#1376,.T.);
#828=FACE_OUTER_BOUND('',#1377,.T.);
#829=FACE_OUTER_BOUND('',#1378,.T.);
#830=FACE_OUTER_BOUND('',#1379,.T.);
#831=FACE_OUTER_BOUND('',#1380,.T.);
#832=FACE_OUTER_BOUND('',#1381,.T.);
#833=FACE_OUTER_BOUND('',#1382,.T.);
#834=FACE_OUTER_BOUND('',#1383,.T.);
#835=FACE_OUTER_BOUND('',#1384,.T.);
#836=FACE_OUTER_BOUND('',#1385,.T.);
#837=FACE_OUTER_BOUND('',#1386,.T.);
#838=FACE_OUTER_BOUND('',#1387,.T.);
#839=FACE_OUTER_BOUND('',#1388,.T.);
#840=FACE_OUTER_BOUND('',#1389,.T.);
#841=FACE_OUTER_BOUND('',#1390,.T.);
#842=FACE_OUTER_BOUND('',#1391,.T.);
#843=FACE_OUTER_BOUND('',#1392,.T.);
#844=FACE_OUTER_BOUND('',#1393,.T.);
#845=FACE_OUTER_BOUND('',#1394,.T.);
#846=FACE_OUTER_BOUND('',#1395,.T.);
#847=FACE_OUTER_BOUND('',#1396,.T.);
#848=FACE_OUTER_BOUND('',#1397,.T.);
#849=FACE_OUTER_BOUND('',#1398,.T.);
#850=FACE_OUTER_BOUND('',#1399,.T.);
#851=FACE_OUTER_BOUND('',#1401,.T.);
#852=FACE_OUTER_BOUND('',#1402,.T.);
#853=FACE_OUTER_BOUND('',#1403,.T.);
#854=FACE_OUTER_BOUND('',#1404,.T.);
#855=FACE_OUTER_BOUND('',#1405,.T.);
#856=FACE_OUTER_BOUND('',#1407,.T.);
#857=FACE_OUTER_BOUND('',#1408,.T.);
#858=FACE_OUTER_BOUND('',#1410,.T.);
#859=FACE_OUTER_BOUND('',#1411,.T.);
#860=FACE_OUTER_BOUND('',#1412,.T.);
#861=FACE_OUTER_BOUND('',#1413,.T.);
#862=FACE_OUTER_BOUND('',#1414,.T.);
#863=FACE_OUTER_BOUND('',#1415,.T.);
#864=FACE_OUTER_BOUND('',#1416,.T.);
#865=FACE_OUTER_BOUND('',#1417,.T.);
#866=FACE_OUTER_BOUND('',#1418,.T.);
#867=FACE_OUTER_BOUND('',#1419,.T.);
#868=FACE_OUTER_BOUND('',#1420,.T.);
#869=FACE_OUTER_BOUND('',#1421,.T.);
#870=FACE_OUTER_BOUND('',#1422,.T.);
#871=FACE_OUTER_BOUND('',#1423,.T.);
#1330=EDGE_LOOP('',(#7054,#7055,#7056,#7057,#7058,#7059,#7060,#7061,#7062,
#7063,#7064));
#1331=EDGE_LOOP('',(#7065,#7066,#7067,#7068));
#1332=EDGE_LOOP('',(#7069,#7070,#7071));
#1333=EDGE_LOOP('',(#7072,#7073,#7074));
#1334=EDGE_LOOP('',(#7075,#7076,#7077));
#1335=EDGE_LOOP('',(#7078,#7079,#7080));
#1336=EDGE_LOOP('',(#7081,#7082,#7083,#7084));
#1337=EDGE_LOOP('',(#7085,#7086,#7087,#7088));
#1338=EDGE_LOOP('',(#7089,#7090,#7091,#7092,#7093));
#1339=EDGE_LOOP('',(#7094,#7095,#7096,#7097));
#1340=EDGE_LOOP('',(#7098,#7099,#7100,#7101,#7102));
#1341=EDGE_LOOP('',(#7103,#7104,#7105,#7106));
#1342=EDGE_LOOP('',(#7107,#7108,#7109,#7110));
#1343=EDGE_LOOP('',(#7111,#7112,#7113,#7114,#7115,#7116,#7117,#7118,#7119,
#7120,#7121));
#1344=EDGE_LOOP('',(#7122,#7123,#7124));
#1345=EDGE_LOOP('',(#7125,#7126,#7127,#7128));
#1346=EDGE_LOOP('',(#7129,#7130,#7131,#7132,#7133,#7134));
#1347=EDGE_LOOP('',(#7135,#7136,#7137,#7138,#7139,#7140));
#1348=EDGE_LOOP('',(#7141,#7142,#7143,#7144,#7145));
#1349=EDGE_LOOP('',(#7146,#7147,#7148,#7149,#7150,#7151));
#1350=EDGE_LOOP('',(#7152,#7153,#7154));
#1351=EDGE_LOOP('',(#7155,#7156,#7157,#7158));
#1352=EDGE_LOOP('',(#7159,#7160,#7161,#7162));
#1353=EDGE_LOOP('',(#7163,#7164,#7165,#7166));
#1354=EDGE_LOOP('',(#7167,#7168,#7169));
#1355=EDGE_LOOP('',(#7170,#7171,#7172,#7173));
#1356=EDGE_LOOP('',(#7174,#7175,#7176,#7177,#7178));
#1357=EDGE_LOOP('',(#7179,#7180,#7181,#7182));
#1358=EDGE_LOOP('',(#7183,#7184,#7185,#7186));
#1359=EDGE_LOOP('',(#7187,#7188,#7189,#7190));
#1360=EDGE_LOOP('',(#7191,#7192,#7193,#7194));
#1361=EDGE_LOOP('',(#7195,#7196,#7197,#7198));
#1362=EDGE_LOOP('',(#7199,#7200,#7201,#7202));
#1363=EDGE_LOOP('',(#7203,#7204,#7205,#7206));
#1364=EDGE_LOOP('',(#7207,#7208,#7209,#7210,#7211));
#1365=EDGE_LOOP('',(#7212,#7213,#7214,#7215));
#1366=EDGE_LOOP('',(#7216,#7217,#7218,#7219,#7220));
#1367=EDGE_LOOP('',(#7221,#7222,#7223,#7224));
#1368=EDGE_LOOP('',(#7225,#7226,#7227));
#1369=EDGE_LOOP('',(#7228,#7229,#7230,#7231));
#1370=EDGE_LOOP('',(#7232,#7233,#7234,#7235));
#1371=EDGE_LOOP('',(#7236,#7237,#7238,#7239));
#1372=EDGE_LOOP('',(#7240,#7241,#7242,#7243));
#1373=EDGE_LOOP('',(#7244,#7245,#7246));
#1374=EDGE_LOOP('',(#7247,#7248,#7249,#7250));
#1375=EDGE_LOOP('',(#7251,#7252,#7253,#7254,#7255));
#1376=EDGE_LOOP('',(#7256,#7257,#7258,#7259,#7260,#7261,#7262,#7263,#7264,
#7265,#7266,#7267));
#1377=EDGE_LOOP('',(#7268,#7269,#7270,#7271,#7272));
#1378=EDGE_LOOP('',(#7273,#7274,#7275,#7276));
#1379=EDGE_LOOP('',(#7277,#7278,#7279,#7280));
#1380=EDGE_LOOP('',(#7281,#7282,#7283,#7284));
#1381=EDGE_LOOP('',(#7285,#7286,#7287,#7288,#7289));
#1382=EDGE_LOOP('',(#7290,#7291,#7292,#7293));
#1383=EDGE_LOOP('',(#7294,#7295,#7296,#7297,#7298,#7299,#7300,#7301,#7302,
#7303,#7304,#7305,#7306,#7307,#7308,#7309));
#1384=EDGE_LOOP('',(#7310,#7311,#7312,#7313));
#1385=EDGE_LOOP('',(#7314,#7315,#7316,#7317));
#1386=EDGE_LOOP('',(#7318,#7319,#7320,#7321));
#1387=EDGE_LOOP('',(#7322,#7323,#7324,#7325,#7326,#7327,#7328,#7329,#7330,
#7331,#7332,#7333,#7334,#7335,#7336,#7337));
#1388=EDGE_LOOP('',(#7338,#7339,#7340,#7341));
#1389=EDGE_LOOP('',(#7342,#7343,#7344,#7345));
#1390=EDGE_LOOP('',(#7346,#7347,#7348,#7349));
#1391=EDGE_LOOP('',(#7350,#7351,#7352,#7353));
#1392=EDGE_LOOP('',(#7354,#7355,#7356,#7357));
#1393=EDGE_LOOP('',(#7358,#7359,#7360,#7361));
#1394=EDGE_LOOP('',(#7362,#7363,#7364,#7365));
#1395=EDGE_LOOP('',(#7366,#7367,#7368,#7369));
#1396=EDGE_LOOP('',(#7370,#7371,#7372,#7373));
#1397=EDGE_LOOP('',(#7374,#7375,#7376,#7377));
#1398=EDGE_LOOP('',(#7378,#7379,#7380,#7381));
#1399=EDGE_LOOP('',(#7382,#7383,#7384,#7385));
#1400=EDGE_LOOP('',(#7386,#7387,#7388,#7389));
#1401=EDGE_LOOP('',(#7390,#7391,#7392));
#1402=EDGE_LOOP('',(#7393,#7394));
#1403=EDGE_LOOP('',(#7395,#7396,#7397,#7398,#7399,#7400,#7401,#7402,#7403));
#1404=EDGE_LOOP('',(#7404,#7405,#7406,#7407,#7408));
#1405=EDGE_LOOP('',(#7409));
#1406=EDGE_LOOP('',(#7410));
#1407=EDGE_LOOP('',(#7411,#7412,#7413,#7414));
#1408=EDGE_LOOP('',(#7415));
#1409=EDGE_LOOP('',(#7416));
#1410=EDGE_LOOP('',(#7417,#7418,#7419,#7420));
#1411=EDGE_LOOP('',(#7421,#7422,#7423,#7424));
#1412=EDGE_LOOP('',(#7425,#7426,#7427,#7428));
#1413=EDGE_LOOP('',(#7429,#7430,#7431,#7432));
#1414=EDGE_LOOP('',(#7433,#7434,#7435,#7436));
#1415=EDGE_LOOP('',(#7437,#7438,#7439));
#1416=EDGE_LOOP('',(#7440,#7441,#7442,#7443));
#1417=EDGE_LOOP('',(#7444,#7445,#7446,#7447));
#1418=EDGE_LOOP('',(#7448,#7449,#7450));
#1419=EDGE_LOOP('',(#7451,#7452,#7453));
#1420=EDGE_LOOP('',(#7454,#7455,#7456,#7457));
#1421=EDGE_LOOP('',(#7458,#7459,#7460,#7461));
#1422=EDGE_LOOP('',(#7462,#7463,#7464,#7465));
#1423=EDGE_LOOP('',(#7466,#7467,#7468,#7469));
#1888=CIRCLE('',#9781,1.00153545743576);
#1889=CIRCLE('',#9782,1.);
#1890=CIRCLE('',#9784,4.3);
#1891=CIRCLE('',#9785,49.4822348431);
#1892=CIRCLE('',#9787,49.4822348431);
#1893=CIRCLE('',#9788,4.3);
#1894=CIRCLE('',#9790,4.3);
#1895=CIRCLE('',#9791,49.4822348431);
#1896=CIRCLE('',#9793,49.4822348431);
#1897=CIRCLE('',#9794,4.3);
#1898=CIRCLE('',#9796,1.0015363217743);
#1899=CIRCLE('',#9797,1.);
#1900=CIRCLE('',#9798,1.000000000559);
#1901=CIRCLE('',#9800,0.5);
#1902=CIRCLE('',#9801,3.8);
#1903=CIRCLE('',#9802,0.5);
#1904=CIRCLE('',#9803,0.5000047256893);
#1905=CIRCLE('',#9805,0.5);
#1906=CIRCLE('',#9806,0.5);
#1907=CIRCLE('',#9807,49.98193025661);
#1908=CIRCLE('',#9808,0.5);
#1909=CIRCLE('',#9809,0.512087492200193);
#1910=CIRCLE('',#9811,0.5);
#1911=CIRCLE('',#9815,0.5);
#1912=CIRCLE('',#9817,3.8);
#1913=CIRCLE('',#9819,3.8);
#1914=CIRCLE('',#9821,3.8);
#1915=CIRCLE('',#9823,3.8);
#1916=CIRCLE('',#9824,3.8);
#1917=CIRCLE('',#9825,0.4999999975627);
#1918=CIRCLE('',#9826,0.5);
#1919=CIRCLE('',#9827,0.5);
#1920=CIRCLE('',#9828,0.5);
#1921=CIRCLE('',#9829,0.5);
#1922=CIRCLE('',#9830,0.5000047256893);
#1923=CIRCLE('',#9831,0.5);
#1924=CIRCLE('',#9833,0.5);
#1925=CIRCLE('',#9834,49.98193025661);
#1926=CIRCLE('',#9835,0.5);
#1927=CIRCLE('',#9836,0.512090006867649);
#1928=CIRCLE('',#9838,0.5);
#1929=CIRCLE('',#9839,0.5);
#1930=CIRCLE('',#9841,0.5);
#1931=CIRCLE('',#9842,0.5);
#1932=CIRCLE('',#9843,0.5);
#1933=CIRCLE('',#9845,0.5);
#1934=CIRCLE('',#9846,1.00152854151208);
#1935=CIRCLE('',#9847,0.512097491395091);
#1936=CIRCLE('',#9849,49.98193025661);
#1937=CIRCLE('',#9850,0.5);
#1938=CIRCLE('',#9851,0.4999999975627);
#1939=CIRCLE('',#9852,0.4999999999921);
#1940=CIRCLE('',#9854,3.8);
#1941=CIRCLE('',#9855,0.5);
#1942=CIRCLE('',#9856,1.);
#1943=CIRCLE('',#9857,0.9999999994882);
#1944=CIRCLE('',#9858,0.5000000000015);
#1945=CIRCLE('',#9859,0.5);
#1946=CIRCLE('',#9860,0.5);
#1947=CIRCLE('',#9861,0.5);
#1948=CIRCLE('',#9862,1.000001436707);
#1949=CIRCLE('',#9864,3.8);
#1950=CIRCLE('',#9866,3.3);
#1951=CIRCLE('',#9867,0.5);
#1952=CIRCLE('',#9868,3.8);
#1953=CIRCLE('',#9870,0.4999999999921);
#1954=CIRCLE('',#9871,0.5);
#1955=CIRCLE('',#9872,1.000000783793);
#1956=CIRCLE('',#9873,1.);
#1957=CIRCLE('',#9875,1.00152887460701);
#1958=CIRCLE('',#9876,0.5);
#1959=CIRCLE('',#9877,0.5);
#1960=CIRCLE('',#9878,0.512097487101245);
#1961=CIRCLE('',#9880,49.98193025661);
#1962=CIRCLE('',#9883,0.5);
#1963=CIRCLE('',#9885,0.5);
#1964=CIRCLE('',#9887,0.5);
#1965=CIRCLE('',#9889,0.5);
#1966=CIRCLE('',#9890,0.5);
#1967=CIRCLE('',#9891,0.5);
#1968=CIRCLE('',#9893,0.5);
#1969=CIRCLE('',#9894,0.5);
#1970=CIRCLE('',#9896,0.5);
#1971=CIRCLE('',#9897,0.5);
#1972=CIRCLE('',#9900,2.6);
#1973=CIRCLE('',#9901,2.6);
#1974=CIRCLE('',#9903,2.6);
#1975=CIRCLE('',#9905,1.25);
#1976=CIRCLE('',#9906,1.25);
#1977=CIRCLE('',#9908,1.25);
#1978=CIRCLE('',#9910,2.5);
#1979=CIRCLE('',#9912,2.5);
#1980=CIRCLE('',#9914,0.5);
#1981=CIRCLE('',#9916,0.5);
#1982=CIRCLE('',#9917,0.5);
#1983=CIRCLE('',#9918,0.5000000000015);
#1984=CIRCLE('',#9919,0.5);
#2260=B_SPLINE_CURVE_WITH_KNOTS('',3,(#29282,#29283,#29284,#29285,#29286,
#29287,#29288,#29289,#29290,#29291,#29292,#29293,#29294,#29295,#29296,#29297,
#29298,#29299,#29300,#29301,#29302,#29303,#29304,#29305,#29306,#29307,#29308,
#29309,#29310,#29311,#29312),.UNSPECIFIED.,.F.,.F.,(4,3,3,3,3,3,3,3,3,3,
4),(5.17641734719844E-7,0.14139019525698,0.25,0.358065836273581,0.426319266401807,
0.5,0.614905428338237,0.713376508714083,0.75,0.93244192277557,1.),
 .UNSPECIFIED.);
#2261=B_SPLINE_CURVE_WITH_KNOTS('',3,(#29316,#29317,#29318,#29319,#29320,
#29321,#29322,#29323,#29324,#29325,#29326,#29327,#29328,#29329,#29330,#29331,
#29332,#29333,#29334,#29335,#29336,#29337,#29338,#29339,#29340,#29341,#29342,
#29343,#29344,#29345,#29346,#29347,#29348,#29349),.UNSPECIFIED.,.F.,.F.,
(4,3,3,3,3,3,3,3,3,3,3,4),(0.,0.128147294183543,0.25,0.279011458040339,
0.376318535302566,0.47243392503047,0.5,0.557339358509396,0.736991852961168,
0.75,0.835809619334612,1.),.UNSPECIFIED.);
#2262=B_SPLINE_CURVE_WITH_KNOTS('',3,(#29353,#29354,#29355,#29356,#29357,
#29358,#29359,#29360),.UNSPECIFIED.,.F.,.F.,(4,1,1,1,1,4),(0.,0.2,0.4,0.6,
0.8,0.999996095345817),.UNSPECIFIED.);
#2263=B_SPLINE_CURVE_WITH_KNOTS('',3,(#29364,#29365,#29366,#29367,#29368,
#29369),.UNSPECIFIED.,.F.,.F.,(4,1,1,4),(0.,0.3333333333333,0.6666666666667,
1.),.UNSPECIFIED.);
#2264=B_SPLINE_CURVE_WITH_KNOTS('',3,(#29371,#29372,#29373,#29374,#29375,
#29376),.UNSPECIFIED.,.F.,.F.,(4,1,1,4),(0.,0.3333333333333,0.6666666666667,
1.),.UNSPECIFIED.);
#2265=B_SPLINE_CURVE_WITH_KNOTS('',3,(#29379,#29380,#29381,#29382,#29383,
#29384,#29385),.UNSPECIFIED.,.F.,.F.,(4,1,1,1,4),(1.0492165877707E-5,0.25,
0.5,0.75,1.),.UNSPECIFIED.);
#2266=B_SPLINE_CURVE_WITH_KNOTS('',3,(#29468,#29469,#29470,#29471,#29472,
#29473,#29474,#29475,#29476,#29477,#29478,#29479,#29480,#29481,#29482,#29483,
#29484,#29485,#29486,#29487,#29488,#29489,#29490,#29491,#29492,#29493,#29494,
#29495,#29496,#29497,#29498,#29499,#29500,#29501,#29502,#29503,#29504),
 .UNSPECIFIED.,.F.,.F.,(4,3,3,3,3,3,3,3,3,3,3,3,4),(0.,0.1666666666667,
0.317615628299898,0.3333333333333,0.5,0.621047457925827,0.6666666666667,
0.768173703229194,0.8333333333333,0.833338977671904,0.909209388752102,0.977689001959099,
1.),.UNSPECIFIED.);
#2267=B_SPLINE_CURVE_WITH_KNOTS('',3,(#29506,#29507,#29508,#29509,#29510,
#29511,#29512,#29513,#29514),.UNSPECIFIED.,.F.,.F.,(4,1,1,1,1,1,4),(0.,
0.1666666666667,0.3333333333333,0.5,0.6666666666667,0.8333333333333,1.),
 .UNSPECIFIED.);
#2268=B_SPLINE_CURVE_WITH_KNOTS('',3,(#29559,#29560,#29561,#29562,#29563,
#29564,#29565,#29566,#29567,#29568,#29569,#29570,#29571,#29572,#29573,#29574,
#29575,#29576,#29577,#29578,#29579,#29580,#29581,#29582,#29583,#29584,#29585,
#29586,#29587,#29588,#29589),.UNSPECIFIED.,.F.,.F.,(4,3,3,3,3,3,3,3,3,3,
4),(1.57239443157975E-10,2.54069330995437E-6,0.15920203487198,0.25,0.376732535787111,
0.5,0.617341130244543,0.727443674691681,0.75,0.883645545754053,1.),
 .UNSPECIFIED.);
#2269=B_SPLINE_CURVE_WITH_KNOTS('',3,(#29591,#29592,#29593,#29594,#29595,
#29596,#29597,#29598,#29599,#29600,#29601,#29602,#29603,#29604,#29605,#29606,
#29607,#29608,#29609,#29610,#29611,#29612,#29613,#29614,#29615,#29616,#29617,
#29618,#29619,#29620,#29621),.UNSPECIFIED.,.F.,.F.,(4,3,3,3,3,3,3,3,3,3,
4),(3.44246750622568E-7,0.142587328061966,0.25,0.357451835441428,0.461548389909148,
0.5,0.597060204860859,0.688202468765424,0.75,0.874999999835037,0.999999999670074),
 .UNSPECIFIED.);
#2270=B_SPLINE_CURVE_WITH_KNOTS('',3,(#29704,#29705,#29706,#29707,#29708,
#29709,#29710,#29711,#29712,#29713,#29714,#29715,#29716,#29717,#29718,#29719,
#29720,#29721,#29722,#29723,#29724,#29725,#29726,#29727,#29728,#29729,#29730,
#29731,#29732,#29733,#29734,#29735,#29736,#29737),.UNSPECIFIED.,.F.,.F.,
(4,3,3,3,3,3,3,3,3,3,3,4),(5.14909641649198E-7,0.142170359375927,0.149743956654906,
0.25,0.357544559632778,0.431986036232602,0.5,0.614360513761462,0.716215156847761,
0.75,0.931218230535921,1.),.UNSPECIFIED.);
#2271=B_SPLINE_CURVE_WITH_KNOTS('',3,(#29740,#29741,#29742,#29743,#29744,
#29745,#29746,#29747,#29748,#29749,#29750,#29751,#29752,#29753,#29754,#29755,
#29756,#29757,#29758),.UNSPECIFIED.,.F.,.F.,(4,3,3,3,3,3,4),(1.66946584494145E-6,
0.1666666666667,0.3333333333333,0.5,0.6666666666667,0.8333333333333,1.),
 .UNSPECIFIED.);
#2272=B_SPLINE_CURVE_WITH_KNOTS('',3,(#29762,#29763,#29764,#29765,#29766,
#29767,#29768,#29769,#29770,#29771,#29772,#29773,#29774,#29775,#29776,#29777,
#29778,#29779,#29780,#29781,#29782,#29783,#29784,#29785,#29786,#29787,#29788,
#29789,#29790,#29791,#29792,#29793,#29794,#29795),.UNSPECIFIED.,.F.,.F.,
(4,3,3,3,3,3,3,3,3,3,3,4),(0.,0.128038283757864,0.25,0.277400491536672,
0.374623655828288,0.47065024139002,0.5,0.554195902331565,0.734425066600767,
0.75,0.831053386463994,1.),.UNSPECIFIED.);
#2273=B_SPLINE_CURVE_WITH_KNOTS('',3,(#29803,#29804,#29805,#29806,#29807,
#29808),.UNSPECIFIED.,.F.,.F.,(4,1,1,4),(0.,0.3333333333333,0.6666666666667,
1.),.UNSPECIFIED.);
#2274=B_SPLINE_CURVE_WITH_KNOTS('',3,(#29809,#29810,#29811,#29812,#29813,
#29814),.UNSPECIFIED.,.F.,.F.,(4,1,1,4),(0.,0.3333333333333,0.6666666666667,
1.),.UNSPECIFIED.);
#2275=B_SPLINE_CURVE_WITH_KNOTS('',3,(#29859,#29860,#29861,#29862,#29863,
#29864,#29865,#29866,#29867,#29868,#29869,#29870,#29871,#29872,#29873,#29874,
#29875,#29876,#29877,#29878,#29879,#29880,#29881,#29882,#29883,#29884,#29885,
#29886,#29887,#29888,#29889,#29890,#29891,#29892,#29893,#29894,#29895,#29896,
#29897,#29898,#29899,#29900,#29901,#29902,#29903,#29904),.UNSPECIFIED.,
 .F.,.F.,(4,3,3,3,3,3,3,3,3,3,3,3,3,3,3,4),(8.27094905990464E-7,3.66882272956542E-6,
0.0936078800827675,0.1666666666667,0.166676616624577,0.262875045155572,
0.3333333333333,0.4504794091647,0.499997157412759,0.5,0.610602034441991,
0.6666666666667,0.794049388469593,0.8333333333333,0.974910700247656,1.),
 .UNSPECIFIED.);
#2276=B_SPLINE_CURVE_WITH_KNOTS('',3,(#29935,#29936,#29937,#29938,#29939,
#29940),.UNSPECIFIED.,.F.,.F.,(4,1,1,4),(0.,0.3333333333333,0.6666666666667,
1.),.UNSPECIFIED.);
#2277=B_SPLINE_CURVE_WITH_KNOTS('',3,(#29944,#29945,#29946,#29947,#29948,
#29949,#29950,#29951,#29952,#29953,#29954,#29955,#29956,#29957,#29958,#29959,
#29960,#29961,#29962,#29963,#29964,#29965,#29966,#29967,#29968,#29969,#29970,
#29971,#29972,#29973,#29974,#29975,#29976,#29977,#29978,#29979,#29980,#29981,
#29982,#29983,#29984,#29985,#29986,#29987,#29988,#29989,#29990,#29991,#29992,
#29993,#29994,#29995,#29996,#29997,#29998,#29999,#30000,#30001,#30002,#30003,
#30004),.UNSPECIFIED.,.F.,.F.,(4,3,3,3,3,3,3,3,3,3,3,3,3,3,3,3,3,3,3,3,
4),(7.22383553753882E-7,0.07142857142857,0.130487248165375,0.1428571428571,
0.2142857142857,0.2857142857143,0.3571428571429,0.4285714285714,0.5,0.5714285714286,
0.6428571428571,0.704095964850392,0.7142857142857,0.771286832638653,0.7857142857143,
0.849372160563138,0.8571428571429,0.917671280130346,0.9285714285714,0.994058581712345,
0.999999942257354),.UNSPECIFIED.);
#2278=B_SPLINE_CURVE_WITH_KNOTS('',3,(#30006,#30007,#30008,#30009,#30010,
#30011,#30012,#30013,#30014,#30015,#30016,#30017,#30018,#30019,#30020,#30021,
#30022,#30023,#30024,#30025,#30026,#30027,#30028,#30029,#30030),
 .UNSPECIFIED.,.F.,.F.,(4,3,3,3,3,3,3,3,4),(0.,0.125,0.25,0.375,0.5,0.625,
0.75,0.875,0.999990443023589),.UNSPECIFIED.);
#2279=B_SPLINE_CURVE_WITH_KNOTS('',3,(#30032,#30033,#30034,#30035,#30036,
#30037,#30038,#30039,#30040,#30041,#30042,#30043,#30044,#30045,#30046,#30047,
#30048,#30049,#30050,#30051,#30052,#30053,#30054,#30055,#30056,#30057,#30058,
#30059,#30060,#30061,#30062,#30063,#30064,#30065,#30066,#30067,#30068,#30069,
#30070,#30071,#30072,#30073,#30074,#30075,#30076,#30077,#30078,#30079,#30080,
#30081,#30082,#30083,#30084,#30085,#30086,#30087,#30088,#30089,#30090,#30091,
#30092),.UNSPECIFIED.,.F.,.F.,(4,3,3,3,3,3,3,3,3,3,3,3,3,3,3,3,3,3,3,3,
4),(0.,0.0663146289378614,0.07692307692308,0.136515469134231,0.1538461538462,
0.211741372047688,0.2307692307692,0.290800694414924,0.3076923076923,0.379751797937426,
0.3846153846154,0.4615384615385,0.5384615384615,0.6153846153846,0.6923076923077,
0.7692307692308,0.828610667313207,0.8461538461538,0.906927705756478,0.9230769230769,
1.),.UNSPECIFIED.);
#2280=B_SPLINE_CURVE_WITH_KNOTS('',3,(#30094,#30095,#30096,#30097,#30098,
#30099,#30100,#30101,#30102,#30103,#30104,#30105,#30106,#30107,#30108,#30109,
#30110,#30111,#30112,#30113,#30114,#30115,#30116,#30117,#30118,#30119,#30120,
#30121),.UNSPECIFIED.,.F.,.F.,(4,3,3,3,3,3,3,3,3,4),(5.14241135831679E-7,
0.160029392004496,0.25,0.375,0.5,0.61640254692559,0.729407831456665,0.75,
0.909028757457081,0.999999999352541),.UNSPECIFIED.);
#2281=B_SPLINE_CURVE_WITH_KNOTS('',3,(#30124,#30125,#30126,#30127,#30128,
#30129,#30130,#30131,#30132,#30133,#30134,#30135,#30136,#30137,#30138,#30139,
#30140,#30141,#30142,#30143,#30144,#30145,#30146,#30147,#30148,#30149,#30150,
#30151),.UNSPECIFIED.,.F.,.F.,(4,3,3,3,3,3,3,3,3,4),(1.70307404208227E-6,
0.148032548383099,0.25,0.362172850239079,0.475120550633577,0.5,0.643652911896944,
0.75,0.936626754284207,1.),.UNSPECIFIED.);
#2282=B_SPLINE_CURVE_WITH_KNOTS('',3,(#30154,#30155,#30156,#30157,#30158,
#30159,#30160,#30161,#30162,#30163,#30164,#30165,#30166,#30167,#30168,#30169,
#30170,#30171,#30172,#30173,#30174,#30175,#30176,#30177,#30178,#30179,#30180,
#30181,#30182,#30183,#30184,#30185,#30186,#30187,#30188,#30189,#30190,#30191,
#30192,#30193,#30194,#30195,#30196,#30197,#30198,#30199,#30200,#30201,#30202,
#30203,#30204,#30205,#30206,#30207,#30208,#30209,#30210,#30211,#30212,#30213,
#30214),.UNSPECIFIED.,.F.,.F.,(4,3,3,3,3,3,3,3,3,3,3,3,3,3,3,3,3,3,3,3,
4),(0.,0.0663146233673017,0.07692307692308,0.136515470169846,0.1538461538462,
0.211741371816719,0.2307692307692,0.290800694481253,0.3076923076923,0.379751797892978,
0.3846153846154,0.4615384615385,0.5384615384615,0.6153846153846,0.6923076923077,
0.7692307692308,0.828610667312714,0.8461538461538,0.906927705758623,0.9230769230769,
1.),.UNSPECIFIED.);
#2283=B_SPLINE_CURVE_WITH_KNOTS('',3,(#30218,#30219,#30220,#30221,#30222,
#30223,#30224,#30225,#30226,#30227,#30228,#30229,#30230,#30231,#30232,#30233,
#30234,#30235,#30236,#30237,#30238,#30239,#30240,#30241,#30242,#30243,#30244,
#30245),.UNSPECIFIED.,.F.,.F.,(4,3,3,3,3,3,3,3,3,4),(1.70307636311285E-6,
0.148032548423123,0.25,0.362172850244707,0.475120550644421,0.5,0.643652911892531,
0.75,0.93662675425471,1.),.UNSPECIFIED.);
#2284=B_SPLINE_CURVE_WITH_KNOTS('',3,(#30247,#30248,#30249,#30250,#30251,
#30252,#30253,#30254,#30255,#30256,#30257,#30258,#30259,#30260,#30261,#30262,
#30263,#30264,#30265,#30266,#30267,#30268,#30269,#30270,#30271,#30272,#30273,
#30274,#30275,#30276,#30277,#30278,#30279,#30280,#30281,#30282,#30283,#30284,
#30285,#30286,#30287,#30288,#30289,#30290,#30291,#30292,#30293,#30294,#30295,
#30296,#30297,#30298,#30299,#30300,#30301,#30302,#30303,#30304,#30305,#30306,
#30307),.UNSPECIFIED.,.F.,.F.,(4,3,3,3,3,3,3,3,3,3,3,3,3,3,3,3,3,3,3,3,
4),(7.22383709612999E-7,0.07142857142857,0.130487248165143,0.1428571428571,
0.2142857142857,0.2857142857143,0.3571428571429,0.4285714285714,0.5,0.5714285714286,
0.6428571428571,0.704095964849231,0.7142857142857,0.77128683263805,0.7857142857143,
0.84937216056434,0.8571428571429,0.917671280131225,0.9285714285714,0.994058581660706,
0.999999946816668),.UNSPECIFIED.);
#2285=B_SPLINE_CURVE_WITH_KNOTS('',3,(#30308,#30309,#30310,#30311,#30312,
#30313,#30314,#30315,#30316,#30317,#30318,#30319,#30320,#30321,#30322,#30323,
#30324,#30325,#30326,#30327,#30328,#30329,#30330,#30331,#30332),
 .UNSPECIFIED.,.F.,.F.,(4,3,3,3,3,3,3,3,4),(0.,0.125,0.25,0.375,0.5,0.625,
0.75,0.875,0.999990443208001),.UNSPECIFIED.);
#2286=B_SPLINE_CURVE_WITH_KNOTS('',3,(#30337,#30338,#30339,#30340,#30341,
#30342,#30343,#30344,#30345,#30346,#30347,#30348,#30349,#30350,#30351,#30352,
#30353,#30354,#30355,#30356,#30357,#30358,#30359,#30360,#30361,#30362,#30363,
#30364,#30365,#30366,#30367),.UNSPECIFIED.,.F.,.F.,(4,3,3,3,3,3,3,3,3,3,
4),(0.,0.125954731287076,0.252411781724506,0.3333333333333,0.430346749055281,
0.526998647703799,0.621788354340608,0.6666666666667,0.794729988522482,0.918392607343539,
0.999999999718069),.UNSPECIFIED.);
#2287=B_SPLINE_CURVE_WITH_KNOTS('',3,(#30369,#30370,#30371,#30372,#30373,
#30374,#30375,#30376,#30377,#30378,#30379,#30380,#30381,#30382,#30383,#30384,
#30385,#30386,#30387,#30388,#30389,#30390,#30391,#30392,#30393,#30394,#30395,
#30396,#30397,#30398,#30399),.UNSPECIFIED.,.F.,.F.,(4,3,3,3,3,3,3,3,3,3,
4),(0.,0.130818468687397,0.261953697017434,0.3333333333333,0.434213916421035,
0.534690323235047,0.633387339807912,0.6666666666667,0.795921234651223,0.92144431339159,
1.),.UNSPECIFIED.);
#2288=B_SPLINE_CURVE_WITH_KNOTS('',3,(#30400,#30401,#30402,#30403,#30404,
#30405),.UNSPECIFIED.,.F.,.F.,(4,1,1,4),(3.63423291666588E-7,0.3333333333333,
0.6666666666667,1.),.UNSPECIFIED.);
#2289=B_SPLINE_CURVE_WITH_KNOTS('',3,(#30409,#30410,#30411,#30412,#30413,
#30414,#30415,#30416,#30417,#30418,#30419,#30420,#30421,#30422,#30423,#30424,
#30425,#30426,#30427,#30428,#30429,#30430,#30431,#30432,#30433,#30434,#30435,
#30436,#30437,#30438,#30439),.UNSPECIFIED.,.F.,.F.,(4,3,3,3,3,3,3,3,3,3,
4),(0.,0.130847171763814,0.262009658964655,0.3333333333333,0.434235825723054,
0.534733660584684,0.633452212258911,0.6666666666667,0.795945015121965,0.921493668359201,
1.),.UNSPECIFIED.);
#2290=B_SPLINE_CURVE_WITH_KNOTS('',3,(#30441,#30442,#30443,#30444,#30445,
#30446),.UNSPECIFIED.,.F.,.F.,(4,1,1,4),(3.63422558971584E-7,0.3333333333333,
0.6666666666667,0.999990003239561),.UNSPECIFIED.);
#2291=B_SPLINE_CURVE_WITH_KNOTS('',3,(#30452,#30453,#30454,#30455,#30456,
#30457),.UNSPECIFIED.,.F.,.F.,(4,1,1,4),(0.,0.3333333333333,0.6666666666667,
1.),.UNSPECIFIED.);
#2292=B_SPLINE_CURVE_WITH_KNOTS('',3,(#30458,#30459,#30460,#30461,#30462,
#30463,#30464,#30465,#30466,#30467,#30468,#30469,#30470,#30471,#30472,#30473,
#30474,#30475,#30476,#30477,#30478,#30479,#30480,#30481,#30482,#30483,#30484,
#30485,#30486,#30487,#30488),.UNSPECIFIED.,.F.,.F.,(4,3,3,3,3,3,3,3,3,3,
4),(0.,0.1259452709169,0.252394138339945,0.3333333333333,0.43034115248585,
0.526987994119367,0.621773123421767,0.6666666666667,0.794723073389028,0.918379100763244,
0.999999999718263),.UNSPECIFIED.);
#2293=B_SPLINE_CURVE_WITH_KNOTS('',3,(#30566,#30567,#30568,#30569,#30570,
#30571,#30572,#30573,#30574,#30575,#30576,#30577,#30578,#30579,#30580,#30581,
#30582,#30583,#30584,#30585,#30586,#30587,#30588,#30589,#30590,#30591,#30592,
#30593,#30594,#30595,#30596,#30597,#30598,#30599,#30600,#30601,#30602,#30603,
#30604,#30605,#30606,#30607,#30608,#30609,#30610,#30611,#30612,#30613,#30614,
#30615,#30616,#30617,#30618,#30619,#30620,#30621,#30622,#30623,#30624,#30625,
#30626,#30627,#30628,#30629,#30630,#30631,#30632,#30633,#30634,#30635,#30636,
#30637,#30638,#30639,#30640,#30641,#30642,#30643,#30644,#30645,#30646,#30647,
#30648,#30649,#30650,#30651,#30652,#30653,#30654,#30655,#30656,#30657,#30658,
#30659,#30660,#30661,#30662,#30663,#30664,#30665),.UNSPECIFIED.,.F.,.F.,
(4,3,3,3,3,3,3,3,3,3,3,3,3,3,3,3,3,3,3,3,3,3,3,3,3,3,3,3,3,3,3,3,3,4),(1.69542913732478E-6,
5.55774553963063E-6,0.0506373367285727,0.06666666666667,0.0714682425632464,
0.115276661695045,0.1333333333333,0.142868118980489,0.2,0.214286769582239,
0.2666666666667,0.28571683247243,0.3333333333333,0.357160916416442,0.4,
0.428567710291777,0.4666666666667,0.499988290679686,0.5333333333333,0.571448700847799,
0.6,0.642858260431062,0.6666666666667,0.714263915658083,0.7333333333333,
0.785692727180372,0.8,0.857135318884438,0.8666666666667,0.919354891573766,
0.928569821196086,0.9333333333333,0.978447646356298,0.999999941726635),
 .UNSPECIFIED.);
#2294=B_SPLINE_CURVE_WITH_KNOTS('',3,(#30710,#30711,#30712,#30713,#30714,
#30715,#30716,#30717,#30718),.UNSPECIFIED.,.F.,.F.,(4,1,1,1,1,1,4),(0.,
0.1666666666667,0.3333333333333,0.5,0.6666666666667,0.8333333333333,1.),
 .UNSPECIFIED.);
#2295=B_SPLINE_CURVE_WITH_KNOTS('',3,(#30769,#30770,#30771,#30772,#30773,
#30774,#30775,#30776,#30777,#30778,#30779,#30780,#30781,#30782,#30783,#30784,
#30785,#30786,#30787,#30788,#30789,#30790),.UNSPECIFIED.,.F.,.F.,(4,3,3,
3,3,3,3,4),(1.1084212699507E-8,0.1428571428571,0.2857142857143,0.4285714285714,
0.5714285714286,0.7142857142857,0.8571428571429,1.),.UNSPECIFIED.);
#2296=B_SPLINE_CURVE_WITH_KNOTS('',3,(#30833,#30834,#30835,#30836,#30837,
#30838,#30839,#30840,#30841,#30842,#30843,#30844,#30845,#30846,#30847,#30848,
#30849,#30850,#30851,#30852,#30853,#30854,#30855,#30856,#30857,#30858,#30859,
#30860,#30861,#30862,#30863,#30864,#30865,#30866,#30867,#30868,#30869,#30870,
#30871,#30872,#30873,#30874,#30875,#30876,#30877,#30878,#30879,#30880,#30881,
#30882,#30883,#30884,#30885,#30886,#30887,#30888,#30889,#30890,#30891,#30892,
#30893,#30894,#30895,#30896,#30897,#30898,#30899,#30900,#30901,#30902,#30903,
#30904,#30905,#30906,#30907,#30908),.UNSPECIFIED.,.F.,.F.,(4,3,3,3,3,3,
3,3,3,3,3,3,3,3,3,3,3,3,3,3,3,3,3,3,3,4),(0.,0.0592153996085023,0.07692307692308,
0.137971746780227,0.1538461538462,0.156168787894468,0.216720874791267,0.2307692307692,
0.298403926768459,0.3076923076923,0.331220102378383,0.3846153846154,0.4615384615385,
0.521400106932983,0.5384615384615,0.6153846153846,0.6923076923077,0.723395663582115,
0.7692307692308,0.816611805544586,0.8461538461538,0.884333781161934,0.9186849174366,
0.9230769230769,0.96998386836785,1.),.UNSPECIFIED.);
#2297=B_SPLINE_CURVE_WITH_KNOTS('',3,(#30910,#30911,#30912,#30913,#30914,
#30915,#30916,#30917,#30918),.UNSPECIFIED.,.F.,.F.,(4,1,1,1,1,1,4),(0.,
0.1666666666667,0.3333333333333,0.5,0.6666666666667,0.8333333333333,1.),
 .UNSPECIFIED.);
#2298=B_SPLINE_CURVE_WITH_KNOTS('',3,(#31029,#31030,#31031,#31032,#31033,
#31034,#31035,#31036,#31037,#31038,#31039,#31040,#31041,#31042,#31043,#31044,
#31045,#31046,#31047,#31048,#31049,#31050,#31051,#31052,#31053,#31054,#31055,
#31056,#31057,#31058,#31059),.UNSPECIFIED.,.F.,.F.,(4,3,3,3,3,3,3,3,3,3,
4),(1.57239599141992E-10,2.54069328459158E-6,0.159202034791914,0.25,0.376732535786759,
0.5,0.617341130243194,0.727443674690462,0.75,0.883645545812357,1.),
 .UNSPECIFIED.);
#2299=B_SPLINE_CURVE_WITH_KNOTS('',3,(#31180,#31181,#31182,#31183,#31184,
#31185,#31186,#31187,#31188,#31189,#31190,#31191,#31192,#31193,#31194,#31195,
#31196,#31197,#31198,#31199,#31200,#31201,#31202,#31203,#31204,#31205,#31206,
#31207,#31208,#31209,#31210,#31211,#31212,#31213,#31214,#31215,#31216,#31217,
#31218,#31219),.UNSPECIFIED.,.F.,.F.,(4,3,3,3,3,3,3,3,3,3,3,3,3,4),(2.2699531152341E-8,
0.103311520700458,0.2,0.286201587337603,0.372168890942023,0.4,0.476223324327245,
0.553399886495743,0.6,0.677580084830424,0.75318919947951,0.8,0.9,1.),
 .UNSPECIFIED.);
#2300=B_SPLINE_CURVE_WITH_KNOTS('',3,(#31221,#31222,#31223,#31224,#31225,
#31226,#31227,#31228,#31229,#31230,#31231,#31232,#31233,#31234,#31235,#31236),
 .UNSPECIFIED.,.F.,.F.,(4,3,3,3,3,4),(6.47517031980386E-8,0.2,0.4,0.6,0.8,
1.),.UNSPECIFIED.);
#2301=B_SPLINE_CURVE_WITH_KNOTS('',3,(#31240,#31241,#31242,#31243,#31244,
#31245,#31246,#31247,#31248,#31249,#31250,#31251,#31252,#31253,#31254,#31255,
#31256,#31257,#31258,#31259,#31260,#31261,#31262,#31263,#31264,#31265,#31266,
#31267,#31268,#31269,#31270,#31271,#31272,#31273,#31274,#31275,#31276,#31277,
#31278,#31279,#31280,#31281,#31282),.UNSPECIFIED.,.F.,.F.,(4,3,3,3,3,3,
3,3,3,3,3,3,3,3,4),(0.,0.13680594551161,0.2,0.285955328618731,0.372421439212899,
0.4,0.479957503419453,0.560598442976324,0.6,0.6842803069857,0.766645874408388,
0.8,0.892157249049824,0.983321048433859,1.),.UNSPECIFIED.);
#2302=B_SPLINE_CURVE_WITH_KNOTS('',3,(#31327,#31328,#31329,#31330,#31331,
#31332,#31333,#31334,#31335,#31336,#31337,#31338,#31339,#31340,#31341,#31342,
#31343,#31344,#31345,#31346,#31347,#31348,#31349,#31350,#31351,#31352,#31353,
#31354,#31355,#31356,#31357,#31358,#31359,#31360,#31361,#31362,#31363,#31364,
#31365,#31366),.UNSPECIFIED.,.F.,.F.,(4,3,3,3,3,3,3,3,3,3,3,3,3,4),(0.,
0.0880591607118253,0.178417667099241,0.2,0.3,0.4,0.489234741416802,0.579519070321251,
0.6,0.702140086482547,0.8,0.9,0.994158707978447,1.),.UNSPECIFIED.);
#2303=B_SPLINE_CURVE_WITH_KNOTS('',3,(#31460,#31461,#31462,#31463,#31464,
#31465,#31466,#31467,#31468,#31469,#31470,#31471,#31472,#31473,#31474,#31475,
#31476,#31477,#31478,#31479,#31480,#31481,#31482,#31483,#31484,#31485,#31486,
#31487),.UNSPECIFIED.,.F.,.F.,(4,3,3,3,3,3,3,3,3,4),(1.21821800129127E-6,
0.160266398966175,0.25,0.364545774686354,0.481323316787605,0.5,0.656740249234776,
0.75,0.933155046279077,1.),.UNSPECIFIED.);
#2304=B_SPLINE_CURVE_WITH_KNOTS('',3,(#31528,#31529,#31530,#31531,#31532,
#31533,#31534,#31535,#31536,#31537,#31538,#31539,#31540,#31541,#31542,#31543,
#31544,#31545,#31546,#31547,#31548,#31549,#31550,#31551,#31552,#31553,#31554,
#31555,#31556,#31557,#31558,#31559,#31560,#31561,#31562,#31563,#31564,#31565,
#31566,#31567),.UNSPECIFIED.,.F.,.F.,(4,3,3,3,3,3,3,3,3,3,3,3,3,4),(0.,
0.174080255493949,0.2,0.333088302546735,0.4,0.539879197218967,0.6,0.715691417056306,
0.8,0.800008541116262,0.881499130100446,0.954334364786703,0.999998056106661,
1.),.UNSPECIFIED.);
#2305=B_SPLINE_CURVE_WITH_KNOTS('',3,(#31648,#31649,#31650,#31651,#31652,
#31653,#31654,#31655,#31656,#31657,#31658,#31659,#31660,#31661,#31662,#31663,
#31664,#31665,#31666,#31667,#31668,#31669,#31670,#31671,#31672,#31673,#31674,
#31675,#31676,#31677,#31678,#31679,#31680,#31681,#31682,#31683,#31684),
 .UNSPECIFIED.,.F.,.F.,(4,3,3,3,3,3,3,3,3,3,3,3,4),(1.14108591780362E-6,
0.115739668942159,0.231444518862999,0.249995974733526,0.25,0.355385370734019,
0.467872041751315,0.5,0.500003046647521,0.684307366792377,0.75,0.933806640317145,
0.999999643059945),.UNSPECIFIED.);
#2306=B_SPLINE_CURVE_WITH_KNOTS('',3,(#31809,#31810,#31811,#31812,#31813,
#31814,#31815,#31816,#31817,#31818,#31819,#31820,#31821,#31822,#31823,#31824,
#31825,#31826,#31827,#31828,#31829,#31830,#31831,#31832,#31833,#31834,#31835,
#31836,#31837,#31838,#31839,#31840,#31841,#31842),.UNSPECIFIED.,.F.,.F.,
(4,3,3,3,3,3,3,3,3,3,3,4),(0.,0.1666666666667,0.3333333333333,0.457241527305633,
0.5,0.634566199399875,0.6666666666667,0.753406160986073,0.8333333333333,
0.842232829732858,0.93919897654023,1.),.UNSPECIFIED.);
#2307=B_SPLINE_CURVE_WITH_KNOTS('',3,(#31925,#31926,#31927,#31928,#31929,
#31930,#31931,#31932,#31933,#31934,#31935,#31936,#31937,#31938,#31939,#31940,
#31941,#31942,#31943,#31944,#31945,#31946,#31947,#31948,#31949,#31950,#31951,
#31952),.UNSPECIFIED.,.F.,.F.,(4,3,3,3,3,3,3,3,3,4),(2.03304784235694E-6,
0.143958436059573,0.24999198002735,0.25,0.428963387921959,0.5,0.674742399991522,
0.75,0.926384911213618,0.999999999165273),.UNSPECIFIED.);
#2308=B_SPLINE_CURVE_WITH_KNOTS('',3,(#31962,#31963,#31964,#31965,#31966,
#31967,#31968,#31969,#31970,#31971,#31972,#31973,#31974,#31975,#31976,#31977,
#31978,#31979,#31980,#31981,#31982,#31983,#31984,#31985,#31986,#31987,#31988,
#31989),.UNSPECIFIED.,.F.,.F.,(4,3,3,3,3,3,3,3,3,4),(8.41153876261982E-7,
0.139660100393563,0.1666666666667,0.3333333333333,0.5,0.644637832867149,
0.6666666666667,0.81340796009515,0.8333333333333,0.999999999532787),
 .UNSPECIFIED.);
#2309=B_SPLINE_CURVE_WITH_KNOTS('',3,(#32095,#32096,#32097,#32098,#32099,
#32100,#32101,#32102,#32103,#32104,#32105,#32106,#32107,#32108,#32109,#32110,
#32111,#32112,#32113,#32114,#32115,#32116,#32117,#32118,#32119,#32120,#32121,
#32122),.UNSPECIFIED.,.F.,.F.,(4,3,3,3,3,3,3,3,3,4),(1.21821525451887E-6,
0.160266398961143,0.25,0.364545774692073,0.481323316799271,0.5,0.656740249229234,
0.75,0.933155046291152,1.),.UNSPECIFIED.);
#2310=B_SPLINE_CURVE_WITH_KNOTS('',3,(#32163,#32164,#32165,#32166,#32167,
#32168,#32169,#32170,#32171,#32172,#32173,#32174,#32175,#32176,#32177,#32178,
#32179,#32180,#32181,#32182,#32183,#32184,#32185,#32186,#32187,#32188,#32189,
#32190,#32191,#32192,#32193,#32194,#32195,#32196,#32197,#32198,#32199,#32200,
#32201,#32202),.UNSPECIFIED.,.F.,.F.,(4,3,3,3,3,3,3,3,3,3,3,3,3,4),(0.,
0.0873072382834166,0.176851949375498,0.2,0.3,0.4,0.489488062363135,0.580299164992892,
0.6,0.7,0.8,0.9,0.994991847753164,1.),.UNSPECIFIED.);
#2311=B_SPLINE_CURVE_WITH_KNOTS('',3,(#32206,#32207,#32208,#32209,#32210,
#32211,#32212),.UNSPECIFIED.,.F.,.F.,(4,1,1,1,4),(4.6145470383373E-8,0.25,
0.5,0.75,1.),.UNSPECIFIED.);
#2312=B_SPLINE_CURVE_WITH_KNOTS('',3,(#32214,#32215,#32216,#32217,#32218,
#32219,#32220,#32221,#32222,#32223,#32224,#32225,#32226,#32227,#32228,#32229,
#32230,#32231,#32232,#32233,#32234,#32235,#32236,#32237,#32238,#32239,#32240,
#32241,#32242,#32243,#32244,#32245,#32246,#32247,#32248,#32249,#32250,#32251,
#32252,#32253,#32254,#32255,#32256,#32257,#32258,#32259,#32260,#32261,#32262,
#32263,#32264,#32265,#32266,#32267,#32268,#32269,#32270,#32271,#32272,#32273,
#32274,#32275,#32276,#32277,#32278,#32279,#32280,#32281,#32282,#32283,#32284,
#32285,#32286,#32287,#32288,#32289,#32290,#32291,#32292,#32293,#32294,#32295,
#32296,#32297,#32298,#32299,#32300,#32301,#32302,#32303,#32304,#32305,#32306,
#32307,#32308,#32309,#32310,#32311,#32312,#32313,#32314,#32315,#32316,#32317,
#32318,#32319,#32320,#32321,#32322,#32323,#32324,#32325,#32326,#32327,#32328,
#32329,#32330,#32331,#32332,#32333,#32334,#32335,#32336,#32337,#32338,#32339,
#32340,#32341,#32342,#32343,#32344,#32345,#32346,#32347,#32348,#32349,#32350,
#32351,#32352),.UNSPECIFIED.,.F.,.F.,(4,3,3,3,3,3,3,3,3,3,3,3,3,3,3,3,3,
3,3,3,3,3,3,3,3,3,3,3,3,3,3,3,3,3,3,3,3,3,3,3,3,3,3,3,3,3,4),(0.,0.0227804383416707,
0.03703703703704,0.07407407407407,0.105393757646733,0.1111111111111,0.1481481481481,
0.171652082563555,0.1851851851852,0.206342119921921,0.2222222222222,0.255267041242846,
0.2592592592593,0.283739101009767,0.2962962962963,0.3333333333333,0.3703703703704,
0.4074074074074,0.441759331394964,0.4444444444444,0.476437287297752,0.4814814814815,
0.5185185185185,0.5555555555556,0.579466611196372,0.5925925925926,0.615050887578397,
0.6296296296296,0.651825697816008,0.6666666666667,0.689429242643129,0.7037037037037,
0.733601140280399,0.7407407407407,0.775250041261276,0.7777777777778,0.811949750863182,
0.8148148148148,0.8518518518519,0.881392679271282,0.8888888888889,0.924034877764861,
0.9259259259259,0.96104211205333,0.962962962963,0.992579641396002,1.),
 .UNSPECIFIED.);
#2313=B_SPLINE_CURVE_WITH_KNOTS('',3,(#32354,#32355,#32356,#32357,#32358,
#32359,#32360,#32361,#32362,#32363,#32364,#32365,#32366),.UNSPECIFIED.,
 .F.,.F.,(4,3,3,3,4),(2.51811213932785E-8,0.25,0.5,0.75,1.),
 .UNSPECIFIED.);
#2314=B_SPLINE_CURVE_WITH_KNOTS('',3,(#32444,#32445,#32446,#32447,#32448,
#32449,#32450,#32451,#32452),.UNSPECIFIED.,.F.,.F.,(4,1,1,1,1,1,4),(0.,
0.1666666666667,0.3333333333333,0.5,0.6666666666667,0.8333333333333,1.),
 .UNSPECIFIED.);
#2315=B_SPLINE_CURVE_WITH_KNOTS('',3,(#32454,#32455,#32456,#32457,#32458,
#32459,#32460,#32461,#32462,#32463,#32464,#32465,#32466,#32467,#32468,#32469,
#32470,#32471,#32472,#32473,#32474,#32475),.UNSPECIFIED.,.F.,.F.,(4,3,3,
3,3,3,3,4),(1.10839718840703E-8,0.1428571428571,0.2857142857143,0.4285714285714,
0.5714285714286,0.7142857142857,0.8571428571429,1.),.UNSPECIFIED.);
#2316=B_SPLINE_CURVE_WITH_KNOTS('',3,(#32476,#32477,#32478,#32479,#32480,
#32481,#32482,#32483,#32484),.UNSPECIFIED.,.F.,.F.,(4,1,1,1,1,1,4),(0.,
0.1666666666667,0.3333333333333,0.5,0.6666666666667,0.8333333333333,1.),
 .UNSPECIFIED.);
#2317=B_SPLINE_CURVE_WITH_KNOTS('',3,(#32486,#32487,#32488,#32489,#32490,
#32491,#32492),.UNSPECIFIED.,.F.,.F.,(4,1,1,1,4),(5.24779788127142E-8,0.25,
0.5,0.75,1.),.UNSPECIFIED.);
#2318=B_SPLINE_CURVE_WITH_KNOTS('',3,(#32494,#32495,#32496,#32497,#32498,
#32499,#32500,#32501,#32502,#32503,#32504,#32505,#32506,#32507,#32508,#32509,
#32510,#32511,#32512,#32513,#32514,#32515,#32516,#32517,#32518,#32519,#32520,
#32521,#32522,#32523,#32524,#32525,#32526,#32527,#32528,#32529,#32530,#32531,
#32532,#32533,#32534,#32535,#32536,#32537,#32538,#32539,#32540,#32541,#32542,
#32543,#32544,#32545,#32546,#32547,#32548,#32549,#32550,#32551,#32552,#32553,
#32554,#32555,#32556,#32557,#32558,#32559,#32560,#32561,#32562,#32563,#32564,
#32565,#32566,#32567,#32568,#32569,#32570,#32571,#32572,#32573,#32574,#32575,
#32576,#32577,#32578,#32579,#32580,#32581,#32582,#32583,#32584,#32585,#32586,
#32587,#32588,#32589,#32590,#32591,#32592,#32593,#32594,#32595,#32596,#32597,
#32598,#32599,#32600,#32601,#32602,#32603,#32604,#32605,#32606,#32607,#32608,
#32609,#32610,#32611,#32612,#32613,#32614,#32615,#32616,#32617,#32618,#32619,
#32620,#32621,#32622,#32623,#32624,#32625,#32626,#32627,#32628,#32629,#32630,
#32631,#32632),.UNSPECIFIED.,.F.,.F.,(4,3,3,3,3,3,3,3,3,3,3,3,3,3,3,3,3,
3,3,3,3,3,3,3,3,3,3,3,3,3,3,3,3,3,3,3,3,3,3,3,3,3,3,3,3,3,4),(0.,0.0227845093839862,
0.03703703703704,0.07407407407407,0.105393728442604,0.1111111111111,0.1481481481481,
0.17169446631537,0.1851851851852,0.206344932871926,0.2222222222222,0.2557035750719,
0.2592592592593,0.283717132387724,0.2962962962963,0.3333333333333,0.3703703703704,
0.4074074074074,0.441952044037632,0.4444444444444,0.476531264648132,0.4814814814815,
0.5185185185185,0.5555555555556,0.579551235001554,0.5925925925926,0.614954621736422,
0.6296296296296,0.651869758798282,0.6666666666667,0.689384247655644,0.7037037037037,
0.733707164566707,0.7407407407407,0.775015711726731,0.7777777777778,0.811946415212526,
0.8148148148148,0.8518518518519,0.881398338187637,0.8888888888889,0.923946377325199,
0.9259259259259,0.96100223100447,0.962962962963,0.992566994343094,1.),
 .UNSPECIFIED.);
#2319=B_SPLINE_CURVE_WITH_KNOTS('',3,(#32634,#32635,#32636,#32637,#32638,
#32639,#32640,#32641,#32642,#32643,#32644,#32645,#32646),.UNSPECIFIED.,
 .F.,.F.,(4,3,3,3,4),(2.9457427153716E-8,0.25,0.5,0.75,1.),
 .UNSPECIFIED.);
#2320=B_SPLINE_CURVE_WITH_KNOTS('',3,(#32649,#32650,#32651,#32652,#32653,
#32654,#32655,#32656,#32657,#32658,#32659,#32660,#32661,#32662,#32663,#32664),
 .UNSPECIFIED.,.F.,.F.,(4,3,3,3,3,4),(7.06541338515659E-8,0.2,0.4,0.6,0.8,
1.),.UNSPECIFIED.);
#2321=B_SPLINE_CURVE_WITH_KNOTS('',3,(#32706,#32707,#32708,#32709,#32710,
#32711,#32712,#32713,#32714,#32715,#32716,#32717,#32718,#32719,#32720,#32721,
#32722,#32723,#32724,#32725,#32726,#32727,#32728,#32729,#32730,#32731,#32732,
#32733,#32734,#32735,#32736,#32737,#32738,#32739,#32740,#32741,#32742,#32743,
#32744,#32745),.UNSPECIFIED.,.F.,.F.,(4,3,3,3,3,3,3,3,3,3,3,3,3,4),(2.47725076196298E-8,
0.10534087193495,0.2,0.289177733415754,0.377970090718556,0.4,0.475948493762322,
0.552624124210195,0.6,0.681040095770149,0.75981969748944,0.8,0.9,1.),
 .UNSPECIFIED.);
#2322=B_SPLINE_CURVE_WITH_KNOTS('',3,(#32750,#32751,#32752,#32753,#32754,
#32755,#32756,#32757,#32758,#32759,#32760,#32761,#32762,#32763,#32764,#32765,
#32766,#32767,#32768,#32769,#32770,#32771,#32772,#32773,#32774,#32775,#32776,
#32777,#32778,#32779,#32780,#32781,#32782,#32783,#32784,#32785,#32786,#32787,
#32788,#32789,#32790,#32791,#32792),.UNSPECIFIED.,.F.,.F.,(4,3,3,3,3,3,
3,3,3,3,3,3,3,3,4),(0.,0.134788958835649,0.2,0.283389163058699,0.36731742804291,
0.4,0.480376948958258,0.561646740947815,0.6,0.680148416600893,0.758660279668076,
0.8,0.89004290129727,0.979061936724548,1.),.UNSPECIFIED.);
#2323=B_SPLINE_CURVE_WITH_KNOTS('',3,(#32976,#32977,#32978,#32979,#32980,
#32981,#32982,#32983,#32984,#32985,#32986,#32987,#32988,#32989,#32990,#32991,
#32992,#32993,#32994,#32995,#32996,#32997,#32998,#32999,#33000,#33001,#33002,
#33003),.UNSPECIFIED.,.F.,.F.,(4,3,3,3,3,3,3,3,3,4),(1.61555868942031E-8,
0.18960286946556,0.25,0.375,0.5,0.625,0.740175560169049,0.75,0.881701904926917,
1.),.UNSPECIFIED.);
#2324=B_SPLINE_CURVE_WITH_KNOTS('',3,(#33008,#33009,#33010,#33011,#33012,
#33013,#33014,#33015,#33016,#33017,#33018,#33019,#33020,#33021,#33022,#33023,
#33024,#33025,#33026,#33027,#33028,#33029,#33030,#33031,#33032),
 .UNSPECIFIED.,.F.,.F.,(4,3,3,3,3,3,3,3,4),(3.13800440150335E-8,0.148044836757143,
0.25,0.381998755728953,0.5,0.625,0.75,0.880006403819899,1.),
 .UNSPECIFIED.);
#2325=B_SPLINE_CURVE_WITH_KNOTS('',3,(#33199,#33200,#33201,#33202,#33203,
#33204,#33205,#33206,#33207,#33208,#33209,#33210,#33211,#33212,#33213,#33214,
#33215,#33216,#33217,#33218,#33219,#33220,#33221,#33222,#33223,#33224,#33225,
#33226,#33227,#33228,#33229,#33230,#33231,#33232,#33233,#33234,#33235,#33236,
#33237,#33238,#33239,#33240,#33241,#33242,#33243,#33244,#33245,#33246,#33247,
#33248,#33249,#33250,#33251,#33252,#33253,#33254,#33255,#33256,#33257,#33258,
#33259,#33260,#33261,#33262,#33263,#33264,#33265,#33266,#33267,#33268,#33269,
#33270,#33271,#33272,#33273,#33274,#33275,#33276,#33277,#33278,#33279,#33280,
#33281,#33282,#33283,#33284,#33285,#33286,#33287,#33288,#33289,#33290,#33291,
#33292,#33293,#33294,#33295,#33296,#33297,#33298,#33299,#33300,#33301,#33302,
#33303,#33304,#33305,#33306,#33307,#33308,#33309,#33310,#33311,#33312,#33313,
#33314,#33315,#33316,#33317,#33318,#33319,#33320,#33321,#33322,#33323,#33324,
#33325,#33326,#33327,#33328,#33329,#33330,#33331,#33332,#33333,#33334,#33335,
#33336,#33337,#33338,#33339,#33340,#33341,#33342,#33343,#33344,#33345,#33346,
#33347,#33348,#33349,#33350,#33351,#33352,#33353,#33354,#33355,#33356,#33357,
#33358,#33359,#33360,#33361,#33362,#33363,#33364,#33365,#33366,#33367,#33368,
#33369,#33370,#33371,#33372,#33373,#33374,#33375,#33376,#33377,#33378,#33379,
#33380,#33381,#33382,#33383,#33384,#33385,#33386,#33387,#33388,#33389,#33390,
#33391),.UNSPECIFIED.,.F.,.F.,(4,3,3,3,3,3,3,3,3,3,3,3,3,3,3,3,3,3,3,3,
3,3,3,3,3,3,3,3,3,3,3,3,3,3,3,3,3,3,3,3,3,3,3,3,3,3,3,3,3,3,3,3,3,3,3,3,
3,3,3,3,3,3,3,3,4),(0.,0.0158753989555512,0.0320140903722559,0.03703703703704,
0.0505952807113718,0.0645704283886565,0.07407407407407,0.092592592592585,
0.1111111111111,0.130016736639153,0.1481481481481,0.16230401228581,0.17679020103838,
0.1851851851852,0.198952837567042,0.212747578072399,0.2222222222222,0.24403267386365,
0.2592592592593,0.276080579509804,0.292869611775802,0.2962962962963,0.318799233780505,
0.3333333333333,0.358324870880841,0.3703703703704,0.4074074074074,0.433897901523346,
0.4444444444444,0.468170095258189,0.4814814814815,0.511388926566693,0.5185185185185,
0.542320497906127,0.5555555555556,0.57190664168362,0.588363012021197,0.5925925925926,
0.607301801204851,0.622385682318724,0.6296296296296,0.64442539279618,0.659647939515595,
0.6666666666667,0.681611773858689,0.696639654563951,0.7037037037037,0.723990226377065,
0.7407407407407,0.76341671663032,0.7777777777778,0.799246099943322,0.8148148148148,
0.841827649657547,0.8518518518519,0.869437743955809,0.886783138376001,0.8888888888889,
0.9074074074074,0.9259259259259,0.942545285990403,0.958686130318573,0.962962962963,
0.984332770802104,1.),.UNSPECIFIED.);
#2326=B_SPLINE_CURVE_WITH_KNOTS('',3,(#33395,#33396,#33397,#33398,#33399,
#33400,#33401,#33402,#33403,#33404,#33405,#33406,#33407,#33408,#33409,#33410,
#33411,#33412,#33413,#33414,#33415,#33416,#33417,#33418,#33419,#33420,#33421,
#33422,#33423,#33424,#33425,#33426,#33427,#33428,#33429,#33430,#33431,#33432,
#33433,#33434,#33435,#33436,#33437,#33438,#33439,#33440,#33441,#33442,#33443,
#33444,#33445,#33446,#33447,#33448,#33449,#33450,#33451,#33452,#33453,#33454,
#33455,#33456,#33457,#33458,#33459,#33460,#33461,#33462,#33463,#33464,#33465,
#33466,#33467,#33468,#33469,#33470,#33471,#33472,#33473,#33474,#33475,#33476,
#33477,#33478,#33479,#33480,#33481,#33482,#33483,#33484,#33485,#33486,#33487,
#33488,#33489,#33490,#33491,#33492,#33493,#33494,#33495,#33496,#33497,#33498,
#33499,#33500,#33501,#33502,#33503,#33504,#33505,#33506,#33507,#33508,#33509,
#33510,#33511,#33512,#33513,#33514,#33515,#33516,#33517,#33518,#33519,#33520,
#33521,#33522,#33523,#33524,#33525,#33526,#33527,#33528,#33529,#33530,#33531,
#33532,#33533,#33534,#33535,#33536,#33537,#33538,#33539,#33540,#33541,#33542,
#33543,#33544,#33545,#33546,#33547,#33548,#33549,#33550,#33551,#33552,#33553,
#33554,#33555,#33556,#33557,#33558,#33559,#33560,#33561,#33562,#33563,#33564,
#33565,#33566,#33567,#33568,#33569,#33570,#33571,#33572,#33573,#33574,#33575,
#33576,#33577,#33578,#33579,#33580,#33581,#33582,#33583,#33584,#33585,#33586,
#33587),.UNSPECIFIED.,.F.,.F.,(4,3,3,3,3,3,3,3,3,3,3,3,3,3,3,3,3,3,3,3,
3,3,3,3,3,3,3,3,3,3,3,3,3,3,3,3,3,3,3,3,3,3,3,3,3,3,3,3,3,3,3,3,3,3,3,3,
3,3,3,3,3,3,3,3,4),(0.,0.0165822562128935,0.0334988362068336,0.03703703703704,
0.0507053457331975,0.0647436237201557,0.07407407407407,0.092592592592585,
0.1111111111111,0.130277373557652,0.1481481481481,0.162380982922882,0.176941705207943,
0.1851851851852,0.199007952753526,0.212869450033032,0.2222222222222,0.243969810128695,
0.2592592592593,0.27600395361121,0.29272868746584,0.2962962962963,0.319534274545662,
0.3333333333333,0.359328590068892,0.3703703703704,0.4074074074074,0.43316432447304,
0.4444444444444,0.467750347323342,0.4814814814815,0.514386802020862,0.5185185185185,
0.54295337501735,0.5555555555556,0.571951925973206,0.588445780819957,0.5925925925926,
0.607248493950731,0.622273991910819,0.6296296296296,0.644556288294263,0.659893419231155,
0.6666666666667,0.681650482058062,0.696707258462661,0.7037037037037,0.724031178536157,
0.7407407407407,0.763131518114845,0.7777777777778,0.799393381195803,0.8148148148148,
0.842210623004667,0.8518518518519,0.8703703703704,0.88776312568209,0.8888888888889,
0.9074074074074,0.9259259259259,0.942566718460714,0.958758891551145,0.962962962963,
0.985139306031294,1.),.UNSPECIFIED.);
#2327=B_SPLINE_CURVE_WITH_KNOTS('',3,(#33591,#33592,#33593,#33594,#33595,
#33596,#33597,#33598,#33599,#33600,#33601,#33602,#33603,#33604),
 .UNSPECIFIED.,.F.,.F.,(4,2,2,2,2,2,4),(-1.42633728259246,-1.37599677975708,
-1.2777147925774,-1.17943280539771,-1.08115081821802,-0.982868831038335,
-0.932528328202956),.UNSPECIFIED.);
#2328=B_SPLINE_CURVE_WITH_KNOTS('',3,(#33606,#33607,#33608,#33609,#33610,
#33611,#33612,#33613,#33614,#33615),.UNSPECIFIED.,.F.,.F.,(4,2,2,2,4),(0.662602885754242,
0.706027743980102,0.805474923937918,0.904922103895734,0.948346962121595),
 .UNSPECIFIED.);
#2329=B_SPLINE_CURVE_WITH_KNOTS('',3,(#33617,#33618,#33619,#33620,#33621,
#33622,#33623,#33624,#33625,#33626,#33627,#33628,#33629,#33630),
 .UNSPECIFIED.,.F.,.F.,(4,2,2,2,2,2,4),(-0.640048745660657,-0.589708242825278,
-0.491426255645591,-0.393144268465903,-0.294862281286216,-0.196580294106529,
-0.146239791271149),.UNSPECIFIED.);
#2330=B_SPLINE_CURVE_WITH_KNOTS('',3,(#33631,#33632,#33633,#33634,#33635,
#33636,#33637,#33638,#33639,#33640,#33641),.UNSPECIFIED.,.F.,.F.,(4,2,3,
2,4),(1.46807780969216,1.51150266791802,1.61094984787584,1.71039702783365,
1.75382188605951),.UNSPECIFIED.);
#2331=B_SPLINE_CURVE_WITH_KNOTS('',3,(#33831,#33832,#33833,#33834,#33835,
#33836,#33837,#33838,#33839,#33840,#33841,#33842,#33843,#33844,#33845,#33846,
#33847,#33848,#33849,#33850,#33851,#33852,#33853,#33854,#33855,#33856,#33857,
#33858),.UNSPECIFIED.,.F.,.F.,(4,3,3,3,3,3,3,3,3,4),(3.56871364693513E-8,
0.189519225027544,0.25,0.375012101554345,0.5,0.625,0.741012963505921,0.75,
0.88392559174732,1.),.UNSPECIFIED.);
#2332=B_SPLINE_CURVE_WITH_KNOTS('',3,(#33860,#33861,#33862,#33863,#33864,
#33865,#33866,#33867,#33868,#33869,#33870,#33871,#33872,#33873,#33874,#33875,
#33876,#33877,#33878,#33879,#33880,#33881,#33882,#33883,#33884,#33885,#33886,
#33887),.UNSPECIFIED.,.F.,.F.,(4,3,3,3,3,3,3,3,3,4),(1.38126679696758E-8,
0.187650448938451,0.25,0.375,0.5,0.618621411128423,0.733216918900281,0.75,
0.881423683727945,1.),.UNSPECIFIED.);
#2333=B_SPLINE_CURVE_WITH_KNOTS('',3,(#33964,#33965,#33966,#33967,#33968,
#33969,#33970,#33971,#33972,#33973,#33974,#33975,#33976,#33977,#33978,#33979,
#33980,#33981,#33982,#33983,#33984,#33985,#33986,#33987,#33988,#33989,#33990,
#33991,#33992,#33993,#33994,#33995,#33996,#33997,#33998,#33999,#34000,#34001,
#34002,#34003,#34004,#34005,#34006,#34007,#34008,#34009,#34010,#34011,#34012,
#34013,#34014,#34015,#34016,#34017,#34018,#34019,#34020,#34021,#34022,#34023,
#34024,#34025,#34026,#34027,#34028,#34029,#34030,#34031,#34032,#34033,#34034,
#34035,#34036,#34037,#34038,#34039),.UNSPECIFIED.,.F.,.F.,(4,3,3,3,3,3,
3,3,3,3,3,3,3,3,3,3,3,3,3,3,3,3,3,3,3,4),(1.69545582308687E-6,0.0609595895495215,
0.06666666666667,0.10840451091604,0.11607460416853,0.1333333333333,0.2,
0.2666666666667,0.311268715280741,0.3333333333333,0.4,0.4666666666667,0.501758645465729,
0.5333333333333,0.6,0.6666666666667,0.683482450052278,0.7333333333333,0.796163252121639,
0.8,0.850694627387244,0.8666666666667,0.926125080370586,0.9333333333333,
0.990551624959652,0.999999945911362),.UNSPECIFIED.);
#2334=B_SPLINE_CURVE_WITH_KNOTS('',3,(#34206,#34207,#34208,#34209,#34210,
#34211,#34212,#34213,#34214,#34215,#34216,#34217,#34218,#34219,#34220,#34221,
#34222,#34223,#34224,#34225,#34226,#34227,#34228,#34229,#34230,#34231,#34232,
#34233,#34234,#34235,#34236,#34237,#34238,#34239,#34240,#34241,#34242,#34243,
#34244,#34245,#34246,#34247,#34248,#34249,#34250,#34251,#34252,#34253,#34254,
#34255,#34256,#34257,#34258,#34259,#34260,#34261,#34262,#34263,#34264,#34265,
#34266,#34267,#34268,#34269,#34270,#34271,#34272,#34273,#34274,#34275,#34276,
#34277,#34278,#34279,#34280,#34281),.UNSPECIFIED.,.F.,.F.,(4,3,3,3,3,3,
3,3,3,3,3,3,3,3,3,3,3,3,3,3,3,3,3,3,3,4),(0.,0.0592153998652141,0.07692307692308,
0.137971745989572,0.1538461538462,0.156168787892723,0.216720875042898,0.2307692307692,
0.298403926666996,0.3076923076923,0.331220102375332,0.3846153846154,0.4615384615385,
0.521400106929585,0.5384615384615,0.6153846153846,0.6923076923077,0.723395663579233,
0.7692307692308,0.816611805544925,0.8461538461538,0.88433378116142,0.918684917435874,
0.9230769230769,0.969983868366533,1.),.UNSPECIFIED.);
#2335=B_SPLINE_CURVE_WITH_KNOTS('',3,(#34398,#34399,#34400,#34401,#34402,
#34403,#34404,#34405,#34406,#34407,#34408,#34409,#34410,#34411,#34412,#34413,
#34414,#34415,#34416,#34417,#34418,#34419,#34420,#34421,#34422,#34423,#34424,
#34425,#34426,#34427,#34428,#34429,#34430,#34431),.UNSPECIFIED.,.F.,.F.,
(4,3,3,3,3,3,3,3,3,3,3,4),(3.05224366949974E-7,0.1666666666667,0.320864307652846,
0.3333333333333,0.5,0.643823830912737,0.6666666666667,0.810437048615872,
0.833327065149254,0.8333333333333,0.963427087902464,1.),.UNSPECIFIED.);
#2732=LINE('',#29280,#3197);
#2733=LINE('',#29314,#3198);
#2734=LINE('',#29351,#3199);
#2735=LINE('',#29389,#3200);
#2736=LINE('',#29395,#3201);
#2737=LINE('',#29402,#3202);
#2738=LINE('',#29413,#3203);
#2739=LINE('',#29421,#3204);
#2740=LINE('',#29760,#3205);
#2741=LINE('',#29797,#3206);
#2742=LINE('',#31283,#3207);
#2743=LINE('',#32204,#3208);
#2744=LINE('',#32367,#3209);
#2745=LINE('',#32401,#3210);
#2746=LINE('',#32405,#3211);
#2747=LINE('',#32406,#3212);
#2748=LINE('',#32441,#3213);
#2749=LINE('',#32648,#3214);
#2750=LINE('',#32749,#3215);
#2751=LINE('',#32900,#3216);
#2752=LINE('',#32904,#3217);
#2753=LINE('',#32905,#3218);
#2754=LINE('',#33007,#3219);
#2755=LINE('',#33588,#3220);
#2756=LINE('',#33652,#3221);
#2757=LINE('',#33656,#3222);
#2758=LINE('',#33663,#3223);
#3197=VECTOR('',#11486,0.6826696020578);
#3198=VECTOR('',#11487,4.991813260128);
#3199=VECTOR('',#11488,0.6826695987007);
#3200=VECTOR('',#11495,0.7035430188284);
#3201=VECTOR('',#11502,0.7035430205274);
#3202=VECTOR('',#11509,0.7035430198318);
#3203=VECTOR('',#11522,0.703543023457);
#3204=VECTOR('',#11531,0.6826696018365);
#3205=VECTOR('',#11564,4.991813260138);
#3206=VECTOR('',#11565,0.6826695985817);
#3207=VECTOR('',#11622,4.875081924963);
#3208=VECTOR('',#11707,10.);
#3209=VECTOR('',#11708,10.);
#3210=VECTOR('',#11709,10.);
#3211=VECTOR('',#11714,10.);
#3212=VECTOR('',#11715,4.493663028249);
#3213=VECTOR('',#11718,10.);
#3214=VECTOR('',#11721,10.);
#3215=VECTOR('',#11726,4.875081924964);
#3216=VECTOR('',#11731,10.);
#3217=VECTOR('',#11736,10.);
#3218=VECTOR('',#11737,4.49366302825);
#3219=VECTOR('',#11744,4.515053245399);
#3220=VECTOR('',#11751,4.5150532454);
#3221=VECTOR('',#11766,1.925);
#3222=VECTOR('',#11771,1.25);
#3223=VECTOR('',#11780,2.5);
#3862=VERTEX_POINT('',#29278);
#3863=VERTEX_POINT('',#29279);
#3864=VERTEX_POINT('',#29281);
#3865=VERTEX_POINT('',#29313);
#3866=VERTEX_POINT('',#29315);
#3867=VERTEX_POINT('',#29350);
#3868=VERTEX_POINT('',#29352);
#3869=VERTEX_POINT('',#29361);
#3870=VERTEX_POINT('',#29363);
#3871=VERTEX_POINT('',#29370);
#3872=VERTEX_POINT('',#29377);
#3873=VERTEX_POINT('',#29387);
#3874=VERTEX_POINT('',#29388);
#3875=VERTEX_POINT('',#29393);
#3876=VERTEX_POINT('',#29394);
#3877=VERTEX_POINT('',#29396);
#3878=VERTEX_POINT('',#29400);
#3879=VERTEX_POINT('',#29401);
#3880=VERTEX_POINT('',#29403);
#3881=VERTEX_POINT('',#29407);
#3882=VERTEX_POINT('',#29411);
#3883=VERTEX_POINT('',#29412);
#3884=VERTEX_POINT('',#29414);
#3885=VERTEX_POINT('',#29418);
#3886=VERTEX_POINT('',#29420);
#3887=VERTEX_POINT('',#29467);
#3888=VERTEX_POINT('',#29505);
#3889=VERTEX_POINT('',#29517);
#3890=VERTEX_POINT('',#29519);
#3891=VERTEX_POINT('',#29558);
#3892=VERTEX_POINT('',#29590);
#3893=VERTEX_POINT('',#29624);
#3894=VERTEX_POINT('',#29626);
#3895=VERTEX_POINT('',#29665);
#3896=VERTEX_POINT('',#29700);
#3897=VERTEX_POINT('',#29702);
#3898=VERTEX_POINT('',#29739);
#3899=VERTEX_POINT('',#29759);
#3900=VERTEX_POINT('',#29761);
#3901=VERTEX_POINT('',#29796);
#3902=VERTEX_POINT('',#29798);
#3903=VERTEX_POINT('',#29800);
#3904=VERTEX_POINT('',#29802);
#3905=VERTEX_POINT('',#29933);
#3906=VERTEX_POINT('',#29942);
#3907=VERTEX_POINT('',#29943);
#3908=VERTEX_POINT('',#30005);
#3909=VERTEX_POINT('',#30031);
#3910=VERTEX_POINT('',#30093);
#3911=VERTEX_POINT('',#30122);
#3912=VERTEX_POINT('',#30153);
#3913=VERTEX_POINT('',#30215);
#3914=VERTEX_POINT('',#30217);
#3915=VERTEX_POINT('',#30246);
#3916=VERTEX_POINT('',#30334);
#3917=VERTEX_POINT('',#30336);
#3918=VERTEX_POINT('',#30368);
#3919=VERTEX_POINT('',#30407);
#3920=VERTEX_POINT('',#30408);
#3921=VERTEX_POINT('',#30440);
#3922=VERTEX_POINT('',#30447);
#3923=VERTEX_POINT('',#30449);
#3924=VERTEX_POINT('',#30451);
#3925=VERTEX_POINT('',#30565);
#3926=VERTEX_POINT('',#30707);
#3927=VERTEX_POINT('',#30709);
#3928=VERTEX_POINT('',#30768);
#3929=VERTEX_POINT('',#30832);
#3930=VERTEX_POINT('',#30909);
#3931=VERTEX_POINT('',#31062);
#3932=VERTEX_POINT('',#31101);
#3933=VERTEX_POINT('',#31136);
#3934=VERTEX_POINT('',#31179);
#3935=VERTEX_POINT('',#31220);
#3936=VERTEX_POINT('',#31239);
#3937=VERTEX_POINT('',#31324);
#3938=VERTEX_POINT('',#31326);
#3939=VERTEX_POINT('',#31400);
#3940=VERTEX_POINT('',#31451);
#3941=VERTEX_POINT('',#31456);
#3942=VERTEX_POINT('',#31458);
#3943=VERTEX_POINT('',#31527);
#3944=VERTEX_POINT('',#31808);
#3945=VERTEX_POINT('',#31956);
#3946=VERTEX_POINT('',#31961);
#3947=VERTEX_POINT('',#32088);
#3948=VERTEX_POINT('',#32090);
#3949=VERTEX_POINT('',#32160);
#3950=VERTEX_POINT('',#32162);
#3951=VERTEX_POINT('',#32203);
#3952=VERTEX_POINT('',#32205);
#3953=VERTEX_POINT('',#32213);
#3954=VERTEX_POINT('',#32353);
#3955=VERTEX_POINT('',#32400);
#3956=VERTEX_POINT('',#32404);
#3957=VERTEX_POINT('',#32439);
#3958=VERTEX_POINT('',#32443);
#3959=VERTEX_POINT('',#32453);
#3960=VERTEX_POINT('',#32485);
#3961=VERTEX_POINT('',#32493);
#3962=VERTEX_POINT('',#32633);
#3963=VERTEX_POINT('',#32647);
#3964=VERTEX_POINT('',#32705);
#3965=VERTEX_POINT('',#32748);
#3966=VERTEX_POINT('',#32899);
#3967=VERTEX_POINT('',#32903);
#3968=VERTEX_POINT('',#32975);
#3969=VERTEX_POINT('',#33006);
#3970=VERTEX_POINT('',#33198);
#3971=VERTEX_POINT('',#33394);
#3972=VERTEX_POINT('',#33589);
#3973=VERTEX_POINT('',#33590);
#3974=VERTEX_POINT('',#33605);
#3975=VERTEX_POINT('',#33616);
#3976=VERTEX_POINT('',#33643);
#3977=VERTEX_POINT('',#33649);
#3978=VERTEX_POINT('',#33650);
#3979=VERTEX_POINT('',#33655);
#3980=VERTEX_POINT('',#33659);
#3981=VERTEX_POINT('',#33662);
#4973=EDGE_CURVE('',#3862,#3863,#2732,.T.);
#4974=EDGE_CURVE('',#3863,#3864,#2260,.T.);
#4975=EDGE_CURVE('',#3865,#3864,#2733,.T.);
#4976=EDGE_CURVE('',#3865,#3866,#2261,.T.);
#4977=EDGE_CURVE('',#3866,#3867,#2734,.T.);
#4978=EDGE_CURVE('',#3867,#3868,#2262,.T.);
#4979=EDGE_CURVE('',#3868,#3869,#84,.T.);
#4980=EDGE_CURVE('',#3870,#3869,#2263,.T.);
#4981=EDGE_CURVE('',#3871,#3870,#2264,.T.);
#4982=EDGE_CURVE('',#3871,#3872,#85,.T.);
#4983=EDGE_CURVE('',#3872,#3862,#2265,.T.);
#4984=EDGE_CURVE('',#3873,#3874,#2735,.T.);
#4985=EDGE_CURVE('',#3863,#3874,#1888,.T.);
#4986=EDGE_CURVE('',#3862,#3873,#1889,.T.);
#4987=EDGE_CURVE('',#3875,#3876,#2736,.T.);
#4988=EDGE_CURVE('',#3877,#3876,#1890,.T.);
#4989=EDGE_CURVE('',#3877,#3875,#1891,.T.);
#4990=EDGE_CURVE('',#3878,#3879,#2737,.T.);
#4991=EDGE_CURVE('',#3879,#3880,#1892,.T.);
#4992=EDGE_CURVE('',#3878,#3880,#1893,.T.);
#4993=EDGE_CURVE('',#3881,#3873,#1894,.T.);
#4994=EDGE_CURVE('',#3881,#3874,#1895,.T.);
#4995=EDGE_CURVE('',#3882,#3883,#2738,.T.);
#4996=EDGE_CURVE('',#3882,#3884,#1896,.T.);
#4997=EDGE_CURVE('',#3883,#3884,#1897,.T.);
#4998=EDGE_CURVE('',#3885,#3875,#1898,.T.);
#4999=EDGE_CURVE('',#3885,#3886,#2739,.T.);
#5000=EDGE_CURVE('',#3876,#3886,#1899,.T.);
#5001=EDGE_CURVE('',#3876,#3887,#2266,.T.);
#5002=EDGE_CURVE('',#3886,#3888,#2267,.T.);
#5003=EDGE_CURVE('',#3887,#3888,#1900,.T.);
#5004=EDGE_CURVE('',#3887,#3889,#1901,.T.);
#5005=EDGE_CURVE('',#3890,#3889,#1902,.T.);
#5006=EDGE_CURVE('',#3877,#3890,#1903,.T.);
#5007=EDGE_CURVE('',#3891,#3877,#2268,.T.);
#5008=EDGE_CURVE('',#3892,#3890,#2269,.T.);
#5009=EDGE_CURVE('',#3891,#3892,#1904,.T.);
#5010=EDGE_CURVE('',#3875,#3893,#1905,.T.);
#5011=EDGE_CURVE('',#3891,#3894,#1906,.T.);
#5012=EDGE_CURVE('',#3894,#3893,#1907,.T.);
#5013=EDGE_CURVE('',#3885,#3895,#1908,.T.);
#5014=EDGE_CURVE('',#3895,#3893,#1909,.T.);
#5015=EDGE_CURVE('',#3895,#3896,#86,.T.);
#5016=EDGE_CURVE('',#3897,#3896,#1910,.T.);
#5017=EDGE_CURVE('',#3885,#3897,#2270,.T.);
#5018=EDGE_CURVE('',#3888,#3898,#2271,.T.);
#5019=EDGE_CURVE('',#3897,#3899,#2740,.T.);
#5020=EDGE_CURVE('',#3899,#3900,#2272,.T.);
#5021=EDGE_CURVE('',#3901,#3900,#2741,.T.);
#5022=EDGE_CURVE('',#3902,#3901,#87,.T.);
#5023=EDGE_CURVE('',#3903,#3902,#88,.T.);
#5024=EDGE_CURVE('',#3904,#3903,#2273,.T.);
#5025=EDGE_CURVE('',#3898,#3904,#2274,.T.);
#5026=EDGE_CURVE('',#3887,#3898,#2275,.T.);
#5027=EDGE_CURVE('',#3898,#3905,#1911,.T.);
#5028=EDGE_CURVE('',#3889,#3905,#2276,.T.);
#5029=EDGE_CURVE('',#3906,#3907,#2277,.T.);
#5030=EDGE_CURVE('',#3907,#3908,#2278,.T.);
#5031=EDGE_CURVE('',#3908,#3909,#2279,.T.);
#5032=EDGE_CURVE('',#3909,#3910,#2280,.T.);
#5033=EDGE_CURVE('',#3911,#3910,#1912,.T.);
#5034=EDGE_CURVE('',#3911,#3906,#2281,.T.);
#5035=EDGE_CURVE('',#3912,#3892,#2282,.T.);
#5036=EDGE_CURVE('',#3913,#3890,#1913,.T.);
#5037=EDGE_CURVE('',#3913,#3914,#2283,.T.);
#5038=EDGE_CURVE('',#3914,#3915,#2284,.T.);
#5039=EDGE_CURVE('',#3915,#3912,#2285,.T.);
#5040=EDGE_CURVE('',#3889,#3916,#1914,.T.);
#5041=EDGE_CURVE('',#3905,#3917,#2286,.T.);
#5042=EDGE_CURVE('',#3917,#3918,#2287,.T.);
#5043=EDGE_CURVE('',#3918,#3916,#2288,.T.);
#5044=EDGE_CURVE('',#3919,#3920,#2289,.T.);
#5045=EDGE_CURVE('',#3920,#3921,#2290,.T.);
#5046=EDGE_CURVE('',#3922,#3921,#1915,.T.);
#5047=EDGE_CURVE('',#3923,#3922,#1916,.T.);
#5048=EDGE_CURVE('',#3923,#3924,#2291,.T.);
#5049=EDGE_CURVE('',#3924,#3919,#2292,.T.);
#5050=EDGE_CURVE('',#3925,#3907,#2293,.T.);
#5051=EDGE_CURVE('',#3925,#3906,#1917,.T.);
#5052=EDGE_CURVE('',#3925,#3926,#1918,.T.);
#5053=EDGE_CURVE('',#3926,#3927,#2294,.T.);
#5054=EDGE_CURVE('',#3907,#3927,#1919,.T.);
#5055=EDGE_CURVE('',#3927,#3928,#2295,.T.);
#5056=EDGE_CURVE('',#3908,#3928,#1920,.T.);
#5057=EDGE_CURVE('',#3908,#3929,#2296,.T.);
#5058=EDGE_CURVE('',#3928,#3930,#2297,.T.);
#5059=EDGE_CURVE('',#3929,#3930,#1921,.T.);
#5060=EDGE_CURVE('',#3929,#3909,#1922,.T.);
#5061=EDGE_CURVE('',#3929,#3881,#2298,.T.);
#5062=EDGE_CURVE('',#3881,#3910,#1923,.T.);
#5063=EDGE_CURVE('',#3874,#3931,#1924,.T.);
#5064=EDGE_CURVE('',#3930,#3931,#1925,.T.);
#5065=EDGE_CURVE('',#3863,#3932,#1926,.T.);
#5066=EDGE_CURVE('',#3932,#3931,#1927,.T.);
#5067=EDGE_CURVE('',#3932,#3933,#89,.T.);
#5068=EDGE_CURVE('',#3864,#3933,#1928,.T.);
#5069=EDGE_CURVE('',#3864,#3934,#2299,.T.);
#5070=EDGE_CURVE('',#3933,#3935,#2300,.T.);
#5071=EDGE_CURVE('',#3934,#3935,#1929,.T.);
#5072=EDGE_CURVE('',#3936,#3865,#2301,.T.);
#5073=EDGE_CURVE('',#3936,#3934,#2742,.T.);
#5074=EDGE_CURVE('',#3936,#3937,#1930,.T.);
#5075=EDGE_CURVE('',#3937,#3938,#2302,.T.);
#5076=EDGE_CURVE('',#3865,#3938,#1931,.T.);
#5077=EDGE_CURVE('',#3866,#3939,#1932,.T.);
#5078=EDGE_CURVE('',#3938,#3939,#90,.T.);
#5079=EDGE_CURVE('',#3882,#3940,#1933,.T.);
#5080=EDGE_CURVE('',#3882,#3866,#1934,.T.);
#5081=EDGE_CURVE('',#3940,#3939,#1935,.T.);
#5082=EDGE_CURVE('',#3940,#3941,#1936,.T.);
#5083=EDGE_CURVE('',#3942,#3941,#1937,.T.);
#5084=EDGE_CURVE('',#3884,#3942,#2303,.T.);
#5085=EDGE_CURVE('',#3942,#3914,#1938,.T.);
#5086=EDGE_CURVE('',#3884,#3913,#1939,.T.);
#5087=EDGE_CURVE('',#3883,#3943,#2304,.T.);
#5088=EDGE_CURVE('',#3921,#3913,#1940,.T.);
#5089=EDGE_CURVE('',#3943,#3921,#1941,.T.);
#5090=EDGE_CURVE('',#3867,#3883,#1942,.T.);
#5091=EDGE_CURVE('',#3868,#3943,#1943,.T.);
#5092=EDGE_CURVE('',#3943,#3869,#2305,.T.);
#5093=EDGE_CURVE('',#3869,#3920,#1944,.T.);
#5094=EDGE_CURVE('',#3870,#3919,#1945,.T.);
#5095=EDGE_CURVE('',#3871,#3924,#1946,.T.);
#5096=EDGE_CURVE('',#3871,#3944,#2306,.T.);
#5097=EDGE_CURVE('',#3944,#3923,#1947,.T.);
#5098=EDGE_CURVE('',#3872,#3944,#1948,.T.);
#5099=EDGE_CURVE('',#3944,#3873,#2307,.T.);
#5100=EDGE_CURVE('',#3910,#3923,#1949,.T.);
#5101=EDGE_CURVE('',#3945,#3945,#1950,.T.);
#5102=EDGE_CURVE('',#3945,#3922,#1951,.T.);
#5103=EDGE_CURVE('',#3916,#3911,#1952,.T.);
#5104=EDGE_CURVE('',#3946,#3878,#2308,.T.);
#5105=EDGE_CURVE('',#3880,#3911,#1953,.T.);
#5106=EDGE_CURVE('',#3946,#3916,#1954,.T.);
#5107=EDGE_CURVE('',#3946,#3902,#1955,.T.);
#5108=EDGE_CURVE('',#3878,#3901,#1956,.T.);
#5109=EDGE_CURVE('',#3879,#3900,#1957,.T.);
#5110=EDGE_CURVE('',#3879,#3947,#1958,.T.);
#5111=EDGE_CURVE('',#3900,#3948,#1959,.T.);
#5112=EDGE_CURVE('',#3947,#3948,#1960,.T.);
#5113=EDGE_CURVE('',#3947,#3926,#1961,.T.);
#5114=EDGE_CURVE('',#3880,#3925,#2309,.T.);
#5115=EDGE_CURVE('',#3949,#3948,#91,.T.);
#5116=EDGE_CURVE('',#3950,#3949,#2310,.T.);
#5117=EDGE_CURVE('',#3951,#3950,#2743,.T.);
#5118=EDGE_CURVE('',#3952,#3951,#2311,.T.);
#5119=EDGE_CURVE('',#3953,#3952,#2312,.T.);
#5120=EDGE_CURVE('',#3954,#3953,#2313,.T.);
#5121=EDGE_CURVE('',#3935,#3954,#2744,.T.);
#5122=EDGE_CURVE('',#3934,#3955,#2745,.T.);
#5123=EDGE_CURVE('',#3955,#3954,#1962,.T.);
#5124=EDGE_CURVE('',#3956,#3936,#2746,.T.);
#5125=EDGE_CURVE('',#3956,#3955,#2747,.T.);
#5126=EDGE_CURVE('',#3956,#3957,#1963,.T.);
#5127=EDGE_CURVE('',#3957,#3937,#2748,.T.);
#5128=EDGE_CURVE('',#3958,#3894,#2314,.T.);
#5129=EDGE_CURVE('',#3959,#3958,#2315,.T.);
#5130=EDGE_CURVE('',#3941,#3959,#2316,.T.);
#5131=EDGE_CURVE('',#3960,#3957,#2317,.T.);
#5132=EDGE_CURVE('',#3961,#3960,#2318,.T.);
#5133=EDGE_CURVE('',#3962,#3961,#2319,.T.);
#5134=EDGE_CURVE('',#3963,#3962,#2749,.T.);
#5135=EDGE_CURVE('',#3896,#3963,#2320,.T.);
#5136=EDGE_CURVE('',#3897,#3964,#2321,.T.);
#5137=EDGE_CURVE('',#3964,#3963,#1964,.T.);
#5138=EDGE_CURVE('',#3964,#3965,#2750,.T.);
#5139=EDGE_CURVE('',#3965,#3899,#2322,.T.);
#5140=EDGE_CURVE('',#3965,#3950,#1965,.T.);
#5141=EDGE_CURVE('',#3899,#3949,#1966,.T.);
#5142=EDGE_CURVE('',#3966,#3965,#2751,.T.);
#5143=EDGE_CURVE('',#3966,#3951,#1967,.T.);
#5144=EDGE_CURVE('',#3964,#3967,#2752,.T.);
#5145=EDGE_CURVE('',#3967,#3966,#2753,.T.);
#5146=EDGE_CURVE('',#3967,#3962,#1968,.T.);
#5147=EDGE_CURVE('',#3967,#3968,#2323,.T.);
#5148=EDGE_CURVE('',#3968,#3961,#1969,.T.);
#5149=EDGE_CURVE('',#3968,#3969,#2754,.T.);
#5150=EDGE_CURVE('',#3969,#3966,#2324,.T.);
#5151=EDGE_CURVE('',#3969,#3952,#1970,.T.);
#5152=EDGE_CURVE('',#3970,#3969,#2325,.T.);
#5153=EDGE_CURVE('',#3970,#3953,#1971,.T.);
#5154=EDGE_CURVE('',#3968,#3971,#2326,.T.);
#5155=EDGE_CURVE('',#3971,#3970,#2755,.T.);
#5156=EDGE_CURVE('',#3972,#3973,#2327,.T.);
#5157=EDGE_CURVE('',#3973,#3974,#2328,.T.);
#5158=EDGE_CURVE('',#3974,#3975,#2329,.T.);
#5159=EDGE_CURVE('',#3975,#3972,#2330,.T.);
#5160=EDGE_CURVE('',#3972,#3976,#1972,.T.);
#5161=EDGE_CURVE('',#3976,#3973,#1973,.T.);
#5162=EDGE_CURVE('',#3975,#3974,#1974,.T.);
#5163=EDGE_CURVE('',#3977,#3978,#1975,.T.);
#5164=EDGE_CURVE('',#3978,#3976,#2756,.T.);
#5165=EDGE_CURVE('',#3978,#3977,#1976,.T.);
#5166=EDGE_CURVE('',#3977,#3979,#2757,.T.);
#5167=EDGE_CURVE('',#3979,#3979,#1977,.T.);
#5168=EDGE_CURVE('',#3980,#3980,#1978,.T.);
#5169=EDGE_CURVE('',#3980,#3981,#2758,.T.);
#5170=EDGE_CURVE('',#3981,#3981,#1979,.T.);
#5171=EDGE_CURVE('',#3971,#3960,#1980,.T.);
#5172=EDGE_CURVE('',#3971,#3956,#2331,.T.);
#5173=EDGE_CURVE('',#3955,#3970,#2332,.T.);
#5174=EDGE_CURVE('',#3942,#3915,#2333,.T.);
#5175=EDGE_CURVE('',#3915,#3959,#1981,.T.);
#5176=EDGE_CURVE('',#3912,#3958,#1982,.T.);
#5177=EDGE_CURVE('',#3912,#3891,#2334,.T.);
#5178=EDGE_CURVE('',#3903,#3946,#2335,.T.);
#5179=EDGE_CURVE('',#3903,#3918,#1983,.T.);
#5180=EDGE_CURVE('',#3904,#3917,#1984,.T.);
#7054=ORIENTED_EDGE('',*,*,#4973,.T.);
#7055=ORIENTED_EDGE('',*,*,#4974,.T.);
#7056=ORIENTED_EDGE('',*,*,#4975,.F.);
#7057=ORIENTED_EDGE('',*,*,#4976,.T.);
#7058=ORIENTED_EDGE('',*,*,#4977,.T.);
#7059=ORIENTED_EDGE('',*,*,#4978,.T.);
#7060=ORIENTED_EDGE('',*,*,#4979,.T.);
#7061=ORIENTED_EDGE('',*,*,#4980,.F.);
#7062=ORIENTED_EDGE('',*,*,#4981,.F.);
#7063=ORIENTED_EDGE('',*,*,#4982,.T.);
#7064=ORIENTED_EDGE('',*,*,#4983,.T.);
#7065=ORIENTED_EDGE('',*,*,#4984,.T.);
#7066=ORIENTED_EDGE('',*,*,#4985,.F.);
#7067=ORIENTED_EDGE('',*,*,#4973,.F.);
#7068=ORIENTED_EDGE('',*,*,#4986,.T.);
#7069=ORIENTED_EDGE('',*,*,#4987,.T.);
#7070=ORIENTED_EDGE('',*,*,#4988,.F.);
#7071=ORIENTED_EDGE('',*,*,#4989,.T.);
#7072=ORIENTED_EDGE('',*,*,#4990,.T.);
#7073=ORIENTED_EDGE('',*,*,#4991,.T.);
#7074=ORIENTED_EDGE('',*,*,#4992,.F.);
#7075=ORIENTED_EDGE('',*,*,#4984,.F.);
#7076=ORIENTED_EDGE('',*,*,#4993,.F.);
#7077=ORIENTED_EDGE('',*,*,#4994,.T.);
#7078=ORIENTED_EDGE('',*,*,#4995,.F.);
#7079=ORIENTED_EDGE('',*,*,#4996,.T.);
#7080=ORIENTED_EDGE('',*,*,#4997,.F.);
#7081=ORIENTED_EDGE('',*,*,#4987,.F.);
#7082=ORIENTED_EDGE('',*,*,#4998,.F.);
#7083=ORIENTED_EDGE('',*,*,#4999,.T.);
#7084=ORIENTED_EDGE('',*,*,#5000,.F.);
#7085=ORIENTED_EDGE('',*,*,#5001,.F.);
#7086=ORIENTED_EDGE('',*,*,#5000,.T.);
#7087=ORIENTED_EDGE('',*,*,#5002,.T.);
#7088=ORIENTED_EDGE('',*,*,#5003,.F.);
#7089=ORIENTED_EDGE('',*,*,#5001,.T.);
#7090=ORIENTED_EDGE('',*,*,#5004,.T.);
#7091=ORIENTED_EDGE('',*,*,#5005,.F.);
#7092=ORIENTED_EDGE('',*,*,#5006,.F.);
#7093=ORIENTED_EDGE('',*,*,#4988,.T.);
#7094=ORIENTED_EDGE('',*,*,#5007,.T.);
#7095=ORIENTED_EDGE('',*,*,#5006,.T.);
#7096=ORIENTED_EDGE('',*,*,#5008,.F.);
#7097=ORIENTED_EDGE('',*,*,#5009,.F.);
#7098=ORIENTED_EDGE('',*,*,#5010,.F.);
#7099=ORIENTED_EDGE('',*,*,#4989,.F.);
#7100=ORIENTED_EDGE('',*,*,#5007,.F.);
#7101=ORIENTED_EDGE('',*,*,#5011,.T.);
#7102=ORIENTED_EDGE('',*,*,#5012,.T.);
#7103=ORIENTED_EDGE('',*,*,#5013,.F.);
#7104=ORIENTED_EDGE('',*,*,#4998,.T.);
#7105=ORIENTED_EDGE('',*,*,#5010,.T.);
#7106=ORIENTED_EDGE('',*,*,#5014,.F.);
#7107=ORIENTED_EDGE('',*,*,#5013,.T.);
#7108=ORIENTED_EDGE('',*,*,#5015,.T.);
#7109=ORIENTED_EDGE('',*,*,#5016,.F.);
#7110=ORIENTED_EDGE('',*,*,#5017,.F.);
#7111=ORIENTED_EDGE('',*,*,#5018,.F.);
#7112=ORIENTED_EDGE('',*,*,#5002,.F.);
#7113=ORIENTED_EDGE('',*,*,#4999,.F.);
#7114=ORIENTED_EDGE('',*,*,#5017,.T.);
#7115=ORIENTED_EDGE('',*,*,#5019,.T.);
#7116=ORIENTED_EDGE('',*,*,#5020,.T.);
#7117=ORIENTED_EDGE('',*,*,#5021,.F.);
#7118=ORIENTED_EDGE('',*,*,#5022,.F.);
#7119=ORIENTED_EDGE('',*,*,#5023,.F.);
#7120=ORIENTED_EDGE('',*,*,#5024,.F.);
#7121=ORIENTED_EDGE('',*,*,#5025,.F.);
#7122=ORIENTED_EDGE('',*,*,#5018,.T.);
#7123=ORIENTED_EDGE('',*,*,#5026,.F.);
#7124=ORIENTED_EDGE('',*,*,#5003,.T.);
#7125=ORIENTED_EDGE('',*,*,#5026,.T.);
#7126=ORIENTED_EDGE('',*,*,#5027,.T.);
#7127=ORIENTED_EDGE('',*,*,#5028,.F.);
#7128=ORIENTED_EDGE('',*,*,#5004,.F.);
#7129=ORIENTED_EDGE('',*,*,#5029,.T.);
#7130=ORIENTED_EDGE('',*,*,#5030,.T.);
#7131=ORIENTED_EDGE('',*,*,#5031,.T.);
#7132=ORIENTED_EDGE('',*,*,#5032,.T.);
#7133=ORIENTED_EDGE('',*,*,#5033,.F.);
#7134=ORIENTED_EDGE('',*,*,#5034,.T.);
#7135=ORIENTED_EDGE('',*,*,#5035,.T.);
#7136=ORIENTED_EDGE('',*,*,#5008,.T.);
#7137=ORIENTED_EDGE('',*,*,#5036,.F.);
#7138=ORIENTED_EDGE('',*,*,#5037,.T.);
#7139=ORIENTED_EDGE('',*,*,#5038,.T.);
#7140=ORIENTED_EDGE('',*,*,#5039,.T.);
#7141=ORIENTED_EDGE('',*,*,#5040,.F.);
#7142=ORIENTED_EDGE('',*,*,#5028,.T.);
#7143=ORIENTED_EDGE('',*,*,#5041,.T.);
#7144=ORIENTED_EDGE('',*,*,#5042,.T.);
#7145=ORIENTED_EDGE('',*,*,#5043,.T.);
#7146=ORIENTED_EDGE('',*,*,#5044,.T.);
#7147=ORIENTED_EDGE('',*,*,#5045,.T.);
#7148=ORIENTED_EDGE('',*,*,#5046,.F.);
#7149=ORIENTED_EDGE('',*,*,#5047,.F.);
#7150=ORIENTED_EDGE('',*,*,#5048,.T.);
#7151=ORIENTED_EDGE('',*,*,#5049,.T.);
#7152=ORIENTED_EDGE('',*,*,#5050,.T.);
#7153=ORIENTED_EDGE('',*,*,#5029,.F.);
#7154=ORIENTED_EDGE('',*,*,#5051,.F.);
#7155=ORIENTED_EDGE('',*,*,#5050,.F.);
#7156=ORIENTED_EDGE('',*,*,#5052,.T.);
#7157=ORIENTED_EDGE('',*,*,#5053,.T.);
#7158=ORIENTED_EDGE('',*,*,#5054,.F.);
#7159=ORIENTED_EDGE('',*,*,#5030,.F.);
#7160=ORIENTED_EDGE('',*,*,#5054,.T.);
#7161=ORIENTED_EDGE('',*,*,#5055,.T.);
#7162=ORIENTED_EDGE('',*,*,#5056,.F.);
#7163=ORIENTED_EDGE('',*,*,#5057,.F.);
#7164=ORIENTED_EDGE('',*,*,#5056,.T.);
#7165=ORIENTED_EDGE('',*,*,#5058,.T.);
#7166=ORIENTED_EDGE('',*,*,#5059,.F.);
#7167=ORIENTED_EDGE('',*,*,#5031,.F.);
#7168=ORIENTED_EDGE('',*,*,#5057,.T.);
#7169=ORIENTED_EDGE('',*,*,#5060,.T.);
#7170=ORIENTED_EDGE('',*,*,#5061,.T.);
#7171=ORIENTED_EDGE('',*,*,#5062,.T.);
#7172=ORIENTED_EDGE('',*,*,#5032,.F.);
#7173=ORIENTED_EDGE('',*,*,#5060,.F.);
#7174=ORIENTED_EDGE('',*,*,#5063,.F.);
#7175=ORIENTED_EDGE('',*,*,#4994,.F.);
#7176=ORIENTED_EDGE('',*,*,#5061,.F.);
#7177=ORIENTED_EDGE('',*,*,#5059,.T.);
#7178=ORIENTED_EDGE('',*,*,#5064,.T.);
#7179=ORIENTED_EDGE('',*,*,#5065,.F.);
#7180=ORIENTED_EDGE('',*,*,#4985,.T.);
#7181=ORIENTED_EDGE('',*,*,#5063,.T.);
#7182=ORIENTED_EDGE('',*,*,#5066,.F.);
#7183=ORIENTED_EDGE('',*,*,#5065,.T.);
#7184=ORIENTED_EDGE('',*,*,#5067,.T.);
#7185=ORIENTED_EDGE('',*,*,#5068,.F.);
#7186=ORIENTED_EDGE('',*,*,#4974,.F.);
#7187=ORIENTED_EDGE('',*,*,#5069,.F.);
#7188=ORIENTED_EDGE('',*,*,#5068,.T.);
#7189=ORIENTED_EDGE('',*,*,#5070,.T.);
#7190=ORIENTED_EDGE('',*,*,#5071,.F.);
#7191=ORIENTED_EDGE('',*,*,#5072,.T.);
#7192=ORIENTED_EDGE('',*,*,#4975,.T.);
#7193=ORIENTED_EDGE('',*,*,#5069,.T.);
#7194=ORIENTED_EDGE('',*,*,#5073,.F.);
#7195=ORIENTED_EDGE('',*,*,#5072,.F.);
#7196=ORIENTED_EDGE('',*,*,#5074,.T.);
#7197=ORIENTED_EDGE('',*,*,#5075,.T.);
#7198=ORIENTED_EDGE('',*,*,#5076,.F.);
#7199=ORIENTED_EDGE('',*,*,#5077,.F.);
#7200=ORIENTED_EDGE('',*,*,#4976,.F.);
#7201=ORIENTED_EDGE('',*,*,#5076,.T.);
#7202=ORIENTED_EDGE('',*,*,#5078,.T.);
#7203=ORIENTED_EDGE('',*,*,#5079,.F.);
#7204=ORIENTED_EDGE('',*,*,#5080,.T.);
#7205=ORIENTED_EDGE('',*,*,#5077,.T.);
#7206=ORIENTED_EDGE('',*,*,#5081,.F.);
#7207=ORIENTED_EDGE('',*,*,#5079,.T.);
#7208=ORIENTED_EDGE('',*,*,#5082,.T.);
#7209=ORIENTED_EDGE('',*,*,#5083,.F.);
#7210=ORIENTED_EDGE('',*,*,#5084,.F.);
#7211=ORIENTED_EDGE('',*,*,#4996,.F.);
#7212=ORIENTED_EDGE('',*,*,#5084,.T.);
#7213=ORIENTED_EDGE('',*,*,#5085,.T.);
#7214=ORIENTED_EDGE('',*,*,#5037,.F.);
#7215=ORIENTED_EDGE('',*,*,#5086,.F.);
#7216=ORIENTED_EDGE('',*,*,#5087,.F.);
#7217=ORIENTED_EDGE('',*,*,#4997,.T.);
#7218=ORIENTED_EDGE('',*,*,#5086,.T.);
#7219=ORIENTED_EDGE('',*,*,#5088,.F.);
#7220=ORIENTED_EDGE('',*,*,#5089,.F.);
#7221=ORIENTED_EDGE('',*,*,#4978,.F.);
#7222=ORIENTED_EDGE('',*,*,#5090,.T.);
#7223=ORIENTED_EDGE('',*,*,#5087,.T.);
#7224=ORIENTED_EDGE('',*,*,#5091,.F.);
#7225=ORIENTED_EDGE('',*,*,#5091,.T.);
#7226=ORIENTED_EDGE('',*,*,#5092,.T.);
#7227=ORIENTED_EDGE('',*,*,#4979,.F.);
#7228=ORIENTED_EDGE('',*,*,#5092,.F.);
#7229=ORIENTED_EDGE('',*,*,#5089,.T.);
#7230=ORIENTED_EDGE('',*,*,#5045,.F.);
#7231=ORIENTED_EDGE('',*,*,#5093,.F.);
#7232=ORIENTED_EDGE('',*,*,#4980,.T.);
#7233=ORIENTED_EDGE('',*,*,#5093,.T.);
#7234=ORIENTED_EDGE('',*,*,#5044,.F.);
#7235=ORIENTED_EDGE('',*,*,#5094,.F.);
#7236=ORIENTED_EDGE('',*,*,#4981,.T.);
#7237=ORIENTED_EDGE('',*,*,#5094,.T.);
#7238=ORIENTED_EDGE('',*,*,#5049,.F.);
#7239=ORIENTED_EDGE('',*,*,#5095,.F.);
#7240=ORIENTED_EDGE('',*,*,#5096,.F.);
#7241=ORIENTED_EDGE('',*,*,#5095,.T.);
#7242=ORIENTED_EDGE('',*,*,#5048,.F.);
#7243=ORIENTED_EDGE('',*,*,#5097,.F.);
#7244=ORIENTED_EDGE('',*,*,#4982,.F.);
#7245=ORIENTED_EDGE('',*,*,#5096,.T.);
#7246=ORIENTED_EDGE('',*,*,#5098,.F.);
#7247=ORIENTED_EDGE('',*,*,#4983,.F.);
#7248=ORIENTED_EDGE('',*,*,#5098,.T.);
#7249=ORIENTED_EDGE('',*,*,#5099,.T.);
#7250=ORIENTED_EDGE('',*,*,#4986,.F.);
#7251=ORIENTED_EDGE('',*,*,#5099,.F.);
#7252=ORIENTED_EDGE('',*,*,#5097,.T.);
#7253=ORIENTED_EDGE('',*,*,#5100,.F.);
#7254=ORIENTED_EDGE('',*,*,#5062,.F.);
#7255=ORIENTED_EDGE('',*,*,#4993,.T.);
#7256=ORIENTED_EDGE('',*,*,#5101,.F.);
#7257=ORIENTED_EDGE('',*,*,#5102,.T.);
#7258=ORIENTED_EDGE('',*,*,#5046,.T.);
#7259=ORIENTED_EDGE('',*,*,#5088,.T.);
#7260=ORIENTED_EDGE('',*,*,#5036,.T.);
#7261=ORIENTED_EDGE('',*,*,#5005,.T.);
#7262=ORIENTED_EDGE('',*,*,#5040,.T.);
#7263=ORIENTED_EDGE('',*,*,#5103,.T.);
#7264=ORIENTED_EDGE('',*,*,#5033,.T.);
#7265=ORIENTED_EDGE('',*,*,#5100,.T.);
#7266=ORIENTED_EDGE('',*,*,#5047,.T.);
#7267=ORIENTED_EDGE('',*,*,#5102,.F.);
#7268=ORIENTED_EDGE('',*,*,#5104,.T.);
#7269=ORIENTED_EDGE('',*,*,#4992,.T.);
#7270=ORIENTED_EDGE('',*,*,#5105,.T.);
#7271=ORIENTED_EDGE('',*,*,#5103,.F.);
#7272=ORIENTED_EDGE('',*,*,#5106,.F.);
#7273=ORIENTED_EDGE('',*,*,#5104,.F.);
#7274=ORIENTED_EDGE('',*,*,#5107,.T.);
#7275=ORIENTED_EDGE('',*,*,#5022,.T.);
#7276=ORIENTED_EDGE('',*,*,#5108,.F.);
#7277=ORIENTED_EDGE('',*,*,#5021,.T.);
#7278=ORIENTED_EDGE('',*,*,#5109,.F.);
#7279=ORIENTED_EDGE('',*,*,#4990,.F.);
#7280=ORIENTED_EDGE('',*,*,#5108,.T.);
#7281=ORIENTED_EDGE('',*,*,#5110,.F.);
#7282=ORIENTED_EDGE('',*,*,#5109,.T.);
#7283=ORIENTED_EDGE('',*,*,#5111,.T.);
#7284=ORIENTED_EDGE('',*,*,#5112,.F.);
#7285=ORIENTED_EDGE('',*,*,#5110,.T.);
#7286=ORIENTED_EDGE('',*,*,#5113,.T.);
#7287=ORIENTED_EDGE('',*,*,#5052,.F.);
#7288=ORIENTED_EDGE('',*,*,#5114,.F.);
#7289=ORIENTED_EDGE('',*,*,#4991,.F.);
#7290=ORIENTED_EDGE('',*,*,#5114,.T.);
#7291=ORIENTED_EDGE('',*,*,#5051,.T.);
#7292=ORIENTED_EDGE('',*,*,#5034,.F.);
#7293=ORIENTED_EDGE('',*,*,#5105,.F.);
#7294=ORIENTED_EDGE('',*,*,#5112,.T.);
#7295=ORIENTED_EDGE('',*,*,#5115,.F.);
#7296=ORIENTED_EDGE('',*,*,#5116,.F.);
#7297=ORIENTED_EDGE('',*,*,#5117,.F.);
#7298=ORIENTED_EDGE('',*,*,#5118,.F.);
#7299=ORIENTED_EDGE('',*,*,#5119,.F.);
#7300=ORIENTED_EDGE('',*,*,#5120,.F.);
#7301=ORIENTED_EDGE('',*,*,#5121,.F.);
#7302=ORIENTED_EDGE('',*,*,#5070,.F.);
#7303=ORIENTED_EDGE('',*,*,#5067,.F.);
#7304=ORIENTED_EDGE('',*,*,#5066,.T.);
#7305=ORIENTED_EDGE('',*,*,#5064,.F.);
#7306=ORIENTED_EDGE('',*,*,#5058,.F.);
#7307=ORIENTED_EDGE('',*,*,#5055,.F.);
#7308=ORIENTED_EDGE('',*,*,#5053,.F.);
#7309=ORIENTED_EDGE('',*,*,#5113,.F.);
#7310=ORIENTED_EDGE('',*,*,#5122,.F.);
#7311=ORIENTED_EDGE('',*,*,#5071,.T.);
#7312=ORIENTED_EDGE('',*,*,#5121,.T.);
#7313=ORIENTED_EDGE('',*,*,#5123,.F.);
#7314=ORIENTED_EDGE('',*,*,#5124,.T.);
#7315=ORIENTED_EDGE('',*,*,#5073,.T.);
#7316=ORIENTED_EDGE('',*,*,#5122,.T.);
#7317=ORIENTED_EDGE('',*,*,#5125,.F.);
#7318=ORIENTED_EDGE('',*,*,#5124,.F.);
#7319=ORIENTED_EDGE('',*,*,#5126,.T.);
#7320=ORIENTED_EDGE('',*,*,#5127,.T.);
#7321=ORIENTED_EDGE('',*,*,#5074,.F.);
#7322=ORIENTED_EDGE('',*,*,#5014,.T.);
#7323=ORIENTED_EDGE('',*,*,#5012,.F.);
#7324=ORIENTED_EDGE('',*,*,#5128,.F.);
#7325=ORIENTED_EDGE('',*,*,#5129,.F.);
#7326=ORIENTED_EDGE('',*,*,#5130,.F.);
#7327=ORIENTED_EDGE('',*,*,#5082,.F.);
#7328=ORIENTED_EDGE('',*,*,#5081,.T.);
#7329=ORIENTED_EDGE('',*,*,#5078,.F.);
#7330=ORIENTED_EDGE('',*,*,#5075,.F.);
#7331=ORIENTED_EDGE('',*,*,#5127,.F.);
#7332=ORIENTED_EDGE('',*,*,#5131,.F.);
#7333=ORIENTED_EDGE('',*,*,#5132,.F.);
#7334=ORIENTED_EDGE('',*,*,#5133,.F.);
#7335=ORIENTED_EDGE('',*,*,#5134,.F.);
#7336=ORIENTED_EDGE('',*,*,#5135,.F.);
#7337=ORIENTED_EDGE('',*,*,#5015,.F.);
#7338=ORIENTED_EDGE('',*,*,#5136,.F.);
#7339=ORIENTED_EDGE('',*,*,#5016,.T.);
#7340=ORIENTED_EDGE('',*,*,#5135,.T.);
#7341=ORIENTED_EDGE('',*,*,#5137,.F.);
#7342=ORIENTED_EDGE('',*,*,#5136,.T.);
#7343=ORIENTED_EDGE('',*,*,#5138,.T.);
#7344=ORIENTED_EDGE('',*,*,#5139,.T.);
#7345=ORIENTED_EDGE('',*,*,#5019,.F.);
#7346=ORIENTED_EDGE('',*,*,#5139,.F.);
#7347=ORIENTED_EDGE('',*,*,#5140,.T.);
#7348=ORIENTED_EDGE('',*,*,#5116,.T.);
#7349=ORIENTED_EDGE('',*,*,#5141,.F.);
#7350=ORIENTED_EDGE('',*,*,#5111,.F.);
#7351=ORIENTED_EDGE('',*,*,#5020,.F.);
#7352=ORIENTED_EDGE('',*,*,#5141,.T.);
#7353=ORIENTED_EDGE('',*,*,#5115,.T.);
#7354=ORIENTED_EDGE('',*,*,#5142,.F.);
#7355=ORIENTED_EDGE('',*,*,#5143,.T.);
#7356=ORIENTED_EDGE('',*,*,#5117,.T.);
#7357=ORIENTED_EDGE('',*,*,#5140,.F.);
#7358=ORIENTED_EDGE('',*,*,#5144,.T.);
#7359=ORIENTED_EDGE('',*,*,#5145,.T.);
#7360=ORIENTED_EDGE('',*,*,#5142,.T.);
#7361=ORIENTED_EDGE('',*,*,#5138,.F.);
#7362=ORIENTED_EDGE('',*,*,#5144,.F.);
#7363=ORIENTED_EDGE('',*,*,#5137,.T.);
#7364=ORIENTED_EDGE('',*,*,#5134,.T.);
#7365=ORIENTED_EDGE('',*,*,#5146,.F.);
#7366=ORIENTED_EDGE('',*,*,#5147,.F.);
#7367=ORIENTED_EDGE('',*,*,#5146,.T.);
#7368=ORIENTED_EDGE('',*,*,#5133,.T.);
#7369=ORIENTED_EDGE('',*,*,#5148,.F.);
#7370=ORIENTED_EDGE('',*,*,#5147,.T.);
#7371=ORIENTED_EDGE('',*,*,#5149,.T.);
#7372=ORIENTED_EDGE('',*,*,#5150,.T.);
#7373=ORIENTED_EDGE('',*,*,#5145,.F.);
#7374=ORIENTED_EDGE('',*,*,#5150,.F.);
#7375=ORIENTED_EDGE('',*,*,#5151,.T.);
#7376=ORIENTED_EDGE('',*,*,#5118,.T.);
#7377=ORIENTED_EDGE('',*,*,#5143,.F.);
#7378=ORIENTED_EDGE('',*,*,#5152,.F.);
#7379=ORIENTED_EDGE('',*,*,#5153,.T.);
#7380=ORIENTED_EDGE('',*,*,#5119,.T.);
#7381=ORIENTED_EDGE('',*,*,#5151,.F.);
#7382=ORIENTED_EDGE('',*,*,#5154,.T.);
#7383=ORIENTED_EDGE('',*,*,#5155,.T.);
#7384=ORIENTED_EDGE('',*,*,#5152,.T.);
#7385=ORIENTED_EDGE('',*,*,#5149,.F.);
#7386=ORIENTED_EDGE('',*,*,#5156,.T.);
#7387=ORIENTED_EDGE('',*,*,#5157,.T.);
#7388=ORIENTED_EDGE('',*,*,#5158,.T.);
#7389=ORIENTED_EDGE('',*,*,#5159,.T.);
#7390=ORIENTED_EDGE('',*,*,#5160,.T.);
#7391=ORIENTED_EDGE('',*,*,#5161,.T.);
#7392=ORIENTED_EDGE('',*,*,#5156,.F.);
#7393=ORIENTED_EDGE('',*,*,#5158,.F.);
#7394=ORIENTED_EDGE('',*,*,#5162,.F.);
#7395=ORIENTED_EDGE('',*,*,#5163,.T.);
#7396=ORIENTED_EDGE('',*,*,#5164,.T.);
#7397=ORIENTED_EDGE('',*,*,#5160,.F.);
#7398=ORIENTED_EDGE('',*,*,#5159,.F.);
#7399=ORIENTED_EDGE('',*,*,#5162,.T.);
#7400=ORIENTED_EDGE('',*,*,#5157,.F.);
#7401=ORIENTED_EDGE('',*,*,#5161,.F.);
#7402=ORIENTED_EDGE('',*,*,#5164,.F.);
#7403=ORIENTED_EDGE('',*,*,#5165,.T.);
#7404=ORIENTED_EDGE('',*,*,#5163,.F.);
#7405=ORIENTED_EDGE('',*,*,#5166,.T.);
#7406=ORIENTED_EDGE('',*,*,#5167,.T.);
#7407=ORIENTED_EDGE('',*,*,#5166,.F.);
#7408=ORIENTED_EDGE('',*,*,#5165,.F.);
#7409=ORIENTED_EDGE('',*,*,#5168,.T.);
#7410=ORIENTED_EDGE('',*,*,#5167,.F.);
#7411=ORIENTED_EDGE('',*,*,#5168,.F.);
#7412=ORIENTED_EDGE('',*,*,#5169,.T.);
#7413=ORIENTED_EDGE('',*,*,#5170,.T.);
#7414=ORIENTED_EDGE('',*,*,#5169,.F.);
#7415=ORIENTED_EDGE('',*,*,#5101,.T.);
#7416=ORIENTED_EDGE('',*,*,#5170,.F.);
#7417=ORIENTED_EDGE('',*,*,#5154,.F.);
#7418=ORIENTED_EDGE('',*,*,#5148,.T.);
#7419=ORIENTED_EDGE('',*,*,#5132,.T.);
#7420=ORIENTED_EDGE('',*,*,#5171,.F.);
#7421=ORIENTED_EDGE('',*,*,#5172,.F.);
#7422=ORIENTED_EDGE('',*,*,#5171,.T.);
#7423=ORIENTED_EDGE('',*,*,#5131,.T.);
#7424=ORIENTED_EDGE('',*,*,#5126,.F.);
#7425=ORIENTED_EDGE('',*,*,#5172,.T.);
#7426=ORIENTED_EDGE('',*,*,#5125,.T.);
#7427=ORIENTED_EDGE('',*,*,#5173,.T.);
#7428=ORIENTED_EDGE('',*,*,#5155,.F.);
#7429=ORIENTED_EDGE('',*,*,#5173,.F.);
#7430=ORIENTED_EDGE('',*,*,#5123,.T.);
#7431=ORIENTED_EDGE('',*,*,#5120,.T.);
#7432=ORIENTED_EDGE('',*,*,#5153,.F.);
#7433=ORIENTED_EDGE('',*,*,#5174,.F.);
#7434=ORIENTED_EDGE('',*,*,#5083,.T.);
#7435=ORIENTED_EDGE('',*,*,#5130,.T.);
#7436=ORIENTED_EDGE('',*,*,#5175,.F.);
#7437=ORIENTED_EDGE('',*,*,#5174,.T.);
#7438=ORIENTED_EDGE('',*,*,#5038,.F.);
#7439=ORIENTED_EDGE('',*,*,#5085,.F.);
#7440=ORIENTED_EDGE('',*,*,#5039,.F.);
#7441=ORIENTED_EDGE('',*,*,#5175,.T.);
#7442=ORIENTED_EDGE('',*,*,#5129,.T.);
#7443=ORIENTED_EDGE('',*,*,#5176,.F.);
#7444=ORIENTED_EDGE('',*,*,#5177,.F.);
#7445=ORIENTED_EDGE('',*,*,#5176,.T.);
#7446=ORIENTED_EDGE('',*,*,#5128,.T.);
#7447=ORIENTED_EDGE('',*,*,#5011,.F.);
#7448=ORIENTED_EDGE('',*,*,#5035,.F.);
#7449=ORIENTED_EDGE('',*,*,#5177,.T.);
#7450=ORIENTED_EDGE('',*,*,#5009,.T.);
#7451=ORIENTED_EDGE('',*,*,#5107,.F.);
#7452=ORIENTED_EDGE('',*,*,#5178,.F.);
#7453=ORIENTED_EDGE('',*,*,#5023,.T.);
#7454=ORIENTED_EDGE('',*,*,#5178,.T.);
#7455=ORIENTED_EDGE('',*,*,#5106,.T.);
#7456=ORIENTED_EDGE('',*,*,#5043,.F.);
#7457=ORIENTED_EDGE('',*,*,#5179,.F.);
#7458=ORIENTED_EDGE('',*,*,#5024,.T.);
#7459=ORIENTED_EDGE('',*,*,#5179,.T.);
#7460=ORIENTED_EDGE('',*,*,#5042,.F.);
#7461=ORIENTED_EDGE('',*,*,#5180,.F.);
#7462=ORIENTED_EDGE('',*,*,#5025,.T.);
#7463=ORIENTED_EDGE('',*,*,#5180,.T.);
#7464=ORIENTED_EDGE('',*,*,#5041,.F.);
#7465=ORIENTED_EDGE('',*,*,#5027,.F.);
#7466=ORIENTED_EDGE('',*,*,#4977,.F.);
#7467=ORIENTED_EDGE('',*,*,#5080,.F.);
#7468=ORIENTED_EDGE('',*,*,#4995,.T.);
#7469=ORIENTED_EDGE('',*,*,#5090,.F.);
#8506=CYLINDRICAL_SURFACE('',#9780,1.);
#8507=CYLINDRICAL_SURFACE('',#9795,1.);
#8508=CYLINDRICAL_SURFACE('',#9816,3.8);
#8509=CYLINDRICAL_SURFACE('',#9818,3.8);
#8510=CYLINDRICAL_SURFACE('',#9820,3.8);
#8511=CYLINDRICAL_SURFACE('',#9822,3.8);
#8512=CYLINDRICAL_SURFACE('',#9840,1.);
#8513=CYLINDRICAL_SURFACE('',#9874,1.);
#8514=CYLINDRICAL_SURFACE('',#9888,1.);
#8515=CYLINDRICAL_SURFACE('',#9895,1.);
#8516=CYLINDRICAL_SURFACE('',#9898,11.8073463034);
#8517=CYLINDRICAL_SURFACE('',#9899,2.6);
#8518=CYLINDRICAL_SURFACE('',#9902,2.6);
#8519=CYLINDRICAL_SURFACE('',#9907,1.25);
#8520=CYLINDRICAL_SURFACE('',#9911,2.5);
#8521=CYLINDRICAL_SURFACE('',#9915,1.);
#8522=CYLINDRICAL_SURFACE('',#9920,1.);
#8844=ADVANCED_FACE('',(#781),#458,.T.);
#8845=ADVANCED_FACE('',(#782),#8506,.T.);
#8846=ADVANCED_FACE('',(#783),#459,.T.);
#8847=ADVANCED_FACE('',(#784),#460,.T.);
#8848=ADVANCED_FACE('',(#785),#461,.T.);
#8849=ADVANCED_FACE('',(#786),#462,.T.);
#8850=ADVANCED_FACE('',(#787),#8507,.T.);
#8851=ADVANCED_FACE('',(#788),#128,.T.);
#8852=ADVANCED_FACE('',(#789),#210,.F.);
#8853=ADVANCED_FACE('',(#790),#129,.F.);
#8854=ADVANCED_FACE('',(#791),#211,.T.);
#8855=ADVANCED_FACE('',(#792),#130,.T.);
#8856=ADVANCED_FACE('',(#793),#131,.T.);
#8857=ADVANCED_FACE('',(#794),#463,.T.);
#8858=ADVANCED_FACE('',(#795),#132,.T.);
#8859=ADVANCED_FACE('',(#796),#133,.F.);
#8860=ADVANCED_FACE('',(#797),#8508,.T.);
#8861=ADVANCED_FACE('',(#798),#8509,.T.);
#8862=ADVANCED_FACE('',(#799),#8510,.T.);
#8863=ADVANCED_FACE('',(#800),#8511,.T.);
#8864=ADVANCED_FACE('',(#801),#134,.F.);
#8865=ADVANCED_FACE('',(#802),#135,.T.);
#8866=ADVANCED_FACE('',(#803),#136,.T.);
#8867=ADVANCED_FACE('',(#804),#137,.T.);
#8868=ADVANCED_FACE('',(#805),#138,.F.);
#8869=ADVANCED_FACE('',(#806),#139,.F.);
#8870=ADVANCED_FACE('',(#807),#212,.T.);
#8871=ADVANCED_FACE('',(#808),#140,.T.);
#8872=ADVANCED_FACE('',(#809),#141,.T.);
#8873=ADVANCED_FACE('',(#810),#142,.T.);
#8874=ADVANCED_FACE('',(#811),#8512,.T.);
#8875=ADVANCED_FACE('',(#812),#143,.T.);
#8876=ADVANCED_FACE('',(#813),#144,.T.);
#8877=ADVANCED_FACE('',(#814),#145,.T.);
#8878=ADVANCED_FACE('',(#815),#213,.T.);
#8879=ADVANCED_FACE('',(#816),#146,.F.);
#8880=ADVANCED_FACE('',(#817),#214,.F.);
#8881=ADVANCED_FACE('',(#818),#147,.T.);
#8882=ADVANCED_FACE('',(#819),#148,.T.);
#8883=ADVANCED_FACE('',(#820),#149,.F.);
#8884=ADVANCED_FACE('',(#821),#150,.F.);
#8885=ADVANCED_FACE('',(#822),#151,.F.);
#8886=ADVANCED_FACE('',(#823),#152,.F.);
#8887=ADVANCED_FACE('',(#824),#153,.T.);
#8888=ADVANCED_FACE('',(#825),#154,.T.);
#8889=ADVANCED_FACE('',(#826),#215,.F.);
#8890=ADVANCED_FACE('',(#827),#216,.T.);
#8891=ADVANCED_FACE('',(#828),#217,.F.);
#8892=ADVANCED_FACE('',(#829),#155,.T.);
#8893=ADVANCED_FACE('',(#830),#8513,.T.);
#8894=ADVANCED_FACE('',(#831),#156,.T.);
#8895=ADVANCED_FACE('',(#832),#218,.T.);
#8896=ADVANCED_FACE('',(#833),#157,.F.);
#8897=ADVANCED_FACE('',(#834),#202,.T.);
#8898=ADVANCED_FACE('',(#835),#158,.T.);
#8899=ADVANCED_FACE('',(#836),#464,.T.);
#8900=ADVANCED_FACE('',(#837),#159,.T.);
#8901=ADVANCED_FACE('',(#838),#203,.T.);
#8902=ADVANCED_FACE('',(#839),#160,.T.);
#8903=ADVANCED_FACE('',(#840),#8514,.T.);
#8904=ADVANCED_FACE('',(#841),#161,.T.);
#8905=ADVANCED_FACE('',(#842),#162,.T.);
#8906=ADVANCED_FACE('',(#843),#163,.T.);
#8907=ADVANCED_FACE('',(#844),#465,.T.);
#8908=ADVANCED_FACE('',(#845),#164,.T.);
#8909=ADVANCED_FACE('',(#846),#165,.T.);
#8910=ADVANCED_FACE('',(#847),#8515,.T.);
#8911=ADVANCED_FACE('',(#848),#166,.T.);
#8912=ADVANCED_FACE('',(#849),#167,.T.);
#8913=ADVANCED_FACE('',(#850,#300),#8516,.T.);
#8914=ADVANCED_FACE('',(#851),#8517,.F.);
#8915=ADVANCED_FACE('',(#852),#8518,.F.);
#8916=ADVANCED_FACE('',(#853),#204,.F.);
#8917=ADVANCED_FACE('',(#854),#8519,.F.);
#8918=ADVANCED_FACE('',(#855,#301),#466,.T.);
#8919=ADVANCED_FACE('',(#856),#8520,.F.);
#8920=ADVANCED_FACE('',(#857,#302),#467,.T.);
#8921=ADVANCED_FACE('',(#858),#168,.T.);
#8922=ADVANCED_FACE('',(#859),#169,.T.);
#8923=ADVANCED_FACE('',(#860),#8521,.T.);
#8924=ADVANCED_FACE('',(#861),#170,.T.);
#8925=ADVANCED_FACE('',(#862),#171,.T.);
#8926=ADVANCED_FACE('',(#863),#172,.F.);
#8927=ADVANCED_FACE('',(#864),#173,.T.);
#8928=ADVANCED_FACE('',(#865),#174,.T.);
#8929=ADVANCED_FACE('',(#866),#175,.F.);
#8930=ADVANCED_FACE('',(#867),#176,.T.);
#8931=ADVANCED_FACE('',(#868),#177,.F.);
#8932=ADVANCED_FACE('',(#869),#178,.F.);
#8933=ADVANCED_FACE('',(#870),#179,.F.);
#8934=ADVANCED_FACE('',(#871),#8522,.T.);
#9123=CLOSED_SHELL('',(#8844,#8845,#8846,#8847,#8848,#8849,#8850,#8851,
#8852,#8853,#8854,#8855,#8856,#8857,#8858,#8859,#8860,#8861,#8862,#8863,
#8864,#8865,#8866,#8867,#8868,#8869,#8870,#8871,#8872,#8873,#8874,#8875,
#8876,#8877,#8878,#8879,#8880,#8881,#8882,#8883,#8884,#8885,#8886,#8887,
#8888,#8889,#8890,#8891,#8892,#8893,#8894,#8895,#8896,#8897,#8898,#8899,
#8900,#8901,#8902,#8903,#8904,#8905,#8906,#8907,#8908,#8909,#8910,#8911,
#8912,#8913,#8914,#8915,#8916,#8917,#8918,#8919,#8920,#8921,#8922,#8923,
#8924,#8925,#8926,#8927,#8928,#8929,#8930,#8931,#8932,#8933,#8934));
#9776=AXIS2_PLACEMENT_3D('',#29276,#11482,#11483);
#9777=AXIS2_PLACEMENT_3D('',#29277,#11484,#11485);
#9778=AXIS2_PLACEMENT_3D('',#29362,#11489,#11490);
#9779=AXIS2_PLACEMENT_3D('',#29378,#11491,#11492);
#9780=AXIS2_PLACEMENT_3D('',#29386,#11493,#11494);
#9781=AXIS2_PLACEMENT_3D('',#29390,#11496,#11497);
#9782=AXIS2_PLACEMENT_3D('',#29391,#11498,#11499);
#9783=AXIS2_PLACEMENT_3D('',#29392,#11500,#11501);
#9784=AXIS2_PLACEMENT_3D('',#29397,#11503,#11504);
#9785=AXIS2_PLACEMENT_3D('',#29398,#11505,#11506);
#9786=AXIS2_PLACEMENT_3D('',#29399,#11507,#11508);
#9787=AXIS2_PLACEMENT_3D('',#29404,#11510,#11511);
#9788=AXIS2_PLACEMENT_3D('',#29405,#11512,#11513);
#9789=AXIS2_PLACEMENT_3D('',#29406,#11514,#11515);
#9790=AXIS2_PLACEMENT_3D('',#29408,#11516,#11517);
#9791=AXIS2_PLACEMENT_3D('',#29409,#11518,#11519);
#9792=AXIS2_PLACEMENT_3D('',#29410,#11520,#11521);
#9793=AXIS2_PLACEMENT_3D('',#29415,#11523,#11524);
#9794=AXIS2_PLACEMENT_3D('',#29416,#11525,#11526);
#9795=AXIS2_PLACEMENT_3D('',#29417,#11527,#11528);
#9796=AXIS2_PLACEMENT_3D('',#29419,#11529,#11530);
#9797=AXIS2_PLACEMENT_3D('',#29422,#11532,#11533);
#9798=AXIS2_PLACEMENT_3D('',#29515,#11534,#11535);
#9799=AXIS2_PLACEMENT_3D('',#29516,#11536,#11537);
#9800=AXIS2_PLACEMENT_3D('',#29518,#11538,#11539);
#9801=AXIS2_PLACEMENT_3D('',#29520,#11540,#11541);
#9802=AXIS2_PLACEMENT_3D('',#29521,#11542,#11543);
#9803=AXIS2_PLACEMENT_3D('',#29622,#11544,#11545);
#9804=AXIS2_PLACEMENT_3D('',#29623,#11546,#11547);
#9805=AXIS2_PLACEMENT_3D('',#29625,#11548,#11549);
#9806=AXIS2_PLACEMENT_3D('',#29627,#11550,#11551);
#9807=AXIS2_PLACEMENT_3D('',#29628,#11552,#11553);
#9808=AXIS2_PLACEMENT_3D('',#29666,#11554,#11555);
#9809=AXIS2_PLACEMENT_3D('',#29667,#11556,#11557);
#9810=AXIS2_PLACEMENT_3D('',#29701,#11558,#11559);
#9811=AXIS2_PLACEMENT_3D('',#29703,#11560,#11561);
#9812=AXIS2_PLACEMENT_3D('',#29738,#11562,#11563);
#9813=AXIS2_PLACEMENT_3D('',#29799,#11566,#11567);
#9814=AXIS2_PLACEMENT_3D('',#29801,#11568,#11569);
#9815=AXIS2_PLACEMENT_3D('',#29934,#11570,#11571);
#9816=AXIS2_PLACEMENT_3D('',#29941,#11572,#11573);
#9817=AXIS2_PLACEMENT_3D('',#30123,#11574,#11575);
#9818=AXIS2_PLACEMENT_3D('',#30152,#11576,#11577);
#9819=AXIS2_PLACEMENT_3D('',#30216,#11578,#11579);
#9820=AXIS2_PLACEMENT_3D('',#30333,#11580,#11581);
#9821=AXIS2_PLACEMENT_3D('',#30335,#11582,#11583);
#9822=AXIS2_PLACEMENT_3D('',#30406,#11584,#11585);
#9823=AXIS2_PLACEMENT_3D('',#30448,#11586,#11587);
#9824=AXIS2_PLACEMENT_3D('',#30450,#11588,#11589);
#9825=AXIS2_PLACEMENT_3D('',#30666,#11590,#11591);
#9826=AXIS2_PLACEMENT_3D('',#30708,#11592,#11593);
#9827=AXIS2_PLACEMENT_3D('',#30719,#11594,#11595);
#9828=AXIS2_PLACEMENT_3D('',#30791,#11596,#11597);
#9829=AXIS2_PLACEMENT_3D('',#30919,#11598,#11599);
#9830=AXIS2_PLACEMENT_3D('',#30992,#11600,#11601);
#9831=AXIS2_PLACEMENT_3D('',#31060,#11602,#11603);
#9832=AXIS2_PLACEMENT_3D('',#31061,#11604,#11605);
#9833=AXIS2_PLACEMENT_3D('',#31063,#11606,#11607);
#9834=AXIS2_PLACEMENT_3D('',#31064,#11608,#11609);
#9835=AXIS2_PLACEMENT_3D('',#31102,#11610,#11611);
#9836=AXIS2_PLACEMENT_3D('',#31103,#11612,#11613);
#9837=AXIS2_PLACEMENT_3D('',#31137,#11614,#11615);
#9838=AXIS2_PLACEMENT_3D('',#31138,#11616,#11617);
#9839=AXIS2_PLACEMENT_3D('',#31237,#11618,#11619);
#9840=AXIS2_PLACEMENT_3D('',#31238,#11620,#11621);
#9841=AXIS2_PLACEMENT_3D('',#31325,#11623,#11624);
#9842=AXIS2_PLACEMENT_3D('',#31367,#11625,#11626);
#9843=AXIS2_PLACEMENT_3D('',#31401,#11627,#11628);
#9844=AXIS2_PLACEMENT_3D('',#31402,#11629,#11630);
#9845=AXIS2_PLACEMENT_3D('',#31452,#11631,#11632);
#9846=AXIS2_PLACEMENT_3D('',#31453,#11633,#11634);
#9847=AXIS2_PLACEMENT_3D('',#31454,#11635,#11636);
#9848=AXIS2_PLACEMENT_3D('',#31455,#11637,#11638);
#9849=AXIS2_PLACEMENT_3D('',#31457,#11639,#11640);
#9850=AXIS2_PLACEMENT_3D('',#31459,#11641,#11642);
#9851=AXIS2_PLACEMENT_3D('',#31524,#11643,#11644);
#9852=AXIS2_PLACEMENT_3D('',#31525,#11645,#11646);
#9853=AXIS2_PLACEMENT_3D('',#31526,#11647,#11648);
#9854=AXIS2_PLACEMENT_3D('',#31568,#11649,#11650);
#9855=AXIS2_PLACEMENT_3D('',#31569,#11651,#11652);
#9856=AXIS2_PLACEMENT_3D('',#31610,#11653,#11654);
#9857=AXIS2_PLACEMENT_3D('',#31611,#11655,#11656);
#9858=AXIS2_PLACEMENT_3D('',#31713,#11657,#11658);
#9859=AXIS2_PLACEMENT_3D('',#31746,#11659,#11660);
#9860=AXIS2_PLACEMENT_3D('',#31779,#11661,#11662);
#9861=AXIS2_PLACEMENT_3D('',#31843,#11663,#11664);
#9862=AXIS2_PLACEMENT_3D('',#31888,#11665,#11666);
#9863=AXIS2_PLACEMENT_3D('',#31953,#11667,#11668);
#9864=AXIS2_PLACEMENT_3D('',#31954,#11669,#11670);
#9865=AXIS2_PLACEMENT_3D('',#31955,#11671,#11672);
#9866=AXIS2_PLACEMENT_3D('',#31957,#11673,#11674);
#9867=AXIS2_PLACEMENT_3D('',#31958,#11675,#11676);
#9868=AXIS2_PLACEMENT_3D('',#31959,#11677,#11678);
#9869=AXIS2_PLACEMENT_3D('',#31960,#11679,#11680);
#9870=AXIS2_PLACEMENT_3D('',#31990,#11681,#11682);
#9871=AXIS2_PLACEMENT_3D('',#31991,#11683,#11684);
#9872=AXIS2_PLACEMENT_3D('',#32036,#11685,#11686);
#9873=AXIS2_PLACEMENT_3D('',#32037,#11687,#11688);
#9874=AXIS2_PLACEMENT_3D('',#32038,#11689,#11690);
#9875=AXIS2_PLACEMENT_3D('',#32039,#11691,#11692);
#9876=AXIS2_PLACEMENT_3D('',#32089,#11693,#11694);
#9877=AXIS2_PLACEMENT_3D('',#32091,#11695,#11696);
#9878=AXIS2_PLACEMENT_3D('',#32092,#11697,#11698);
#9879=AXIS2_PLACEMENT_3D('',#32093,#11699,#11700);
#9880=AXIS2_PLACEMENT_3D('',#32094,#11701,#11702);
#9881=AXIS2_PLACEMENT_3D('',#32159,#11703,#11704);
#9882=AXIS2_PLACEMENT_3D('',#32161,#11705,#11706);
#9883=AXIS2_PLACEMENT_3D('',#32402,#11710,#11711);
#9884=AXIS2_PLACEMENT_3D('',#32403,#11712,#11713);
#9885=AXIS2_PLACEMENT_3D('',#32440,#11716,#11717);
#9886=AXIS2_PLACEMENT_3D('',#32442,#11719,#11720);
#9887=AXIS2_PLACEMENT_3D('',#32746,#11722,#11723);
#9888=AXIS2_PLACEMENT_3D('',#32747,#11724,#11725);
#9889=AXIS2_PLACEMENT_3D('',#32833,#11727,#11728);
#9890=AXIS2_PLACEMENT_3D('',#32834,#11729,#11730);
#9891=AXIS2_PLACEMENT_3D('',#32901,#11732,#11733);
#9892=AXIS2_PLACEMENT_3D('',#32902,#11734,#11735);
#9893=AXIS2_PLACEMENT_3D('',#32938,#11738,#11739);
#9894=AXIS2_PLACEMENT_3D('',#33004,#11740,#11741);
#9895=AXIS2_PLACEMENT_3D('',#33005,#11742,#11743);
#9896=AXIS2_PLACEMENT_3D('',#33069,#11745,#11746);
#9897=AXIS2_PLACEMENT_3D('',#33392,#11747,#11748);
#9898=AXIS2_PLACEMENT_3D('',#33393,#11749,#11750);
#9899=AXIS2_PLACEMENT_3D('',#33642,#11752,#11753);
#9900=AXIS2_PLACEMENT_3D('',#33644,#11754,#11755);
#9901=AXIS2_PLACEMENT_3D('',#33645,#11756,#11757);
#9902=AXIS2_PLACEMENT_3D('',#33646,#11758,#11759);
#9903=AXIS2_PLACEMENT_3D('',#33647,#11760,#11761);
#9904=AXIS2_PLACEMENT_3D('',#33648,#11762,#11763);
#9905=AXIS2_PLACEMENT_3D('',#33651,#11764,#11765);
#9906=AXIS2_PLACEMENT_3D('',#33653,#11767,#11768);
#9907=AXIS2_PLACEMENT_3D('',#33654,#11769,#11770);
#9908=AXIS2_PLACEMENT_3D('',#33657,#11772,#11773);
#9909=AXIS2_PLACEMENT_3D('',#33658,#11774,#11775);
#9910=AXIS2_PLACEMENT_3D('',#33660,#11776,#11777);
#9911=AXIS2_PLACEMENT_3D('',#33661,#11778,#11779);
#9912=AXIS2_PLACEMENT_3D('',#33664,#11781,#11782);
#9913=AXIS2_PLACEMENT_3D('',#33665,#11783,#11784);
#9914=AXIS2_PLACEMENT_3D('',#33794,#11785,#11786);
#9915=AXIS2_PLACEMENT_3D('',#33859,#11787,#11788);
#9916=AXIS2_PLACEMENT_3D('',#34040,#11789,#11790);
#9917=AXIS2_PLACEMENT_3D('',#34165,#11791,#11792);
#9918=AXIS2_PLACEMENT_3D('',#34460,#11793,#11794);
#9919=AXIS2_PLACEMENT_3D('',#34493,#11795,#11796);
#9920=AXIS2_PLACEMENT_3D('',#34526,#11797,#11798);
#11482=DIRECTION('axis',(0.,0.,1.));
#11483=DIRECTION('refdir',(1.,0.,0.));
#11484=DIRECTION('center_axis',(-0.866025403784429,0.,0.500000000000017));
#11485=DIRECTION('ref_axis',(0.500000000000017,0.,0.866025403784429));
#11486=DIRECTION('',(3.731805933989E-9,-1.,-1.76837731384E-9));
#11487=DIRECTION('',(4.187512236206E-13,-1.,7.252305024337E-13));
#11488=DIRECTION('',(-1.797493038896E-8,-1.,1.001821272828E-8));
#11489=DIRECTION('center_axis',(-0.866025403784529,2.50962908580945E-13,
0.499999999999843));
#11490=DIRECTION('ref_axis',(-0.0976799095104206,-0.980731635623266,-0.169186566150357));
#11491=DIRECTION('center_axis',(-0.866025403786267,-1.30314015865624E-12,
0.499999999996833));
#11492=DIRECTION('ref_axis',(0.127371879782138,-0.967008591980107,0.220614567237561));
#11493=DIRECTION('center_axis',(0.,-1.,0.));
#11494=DIRECTION('ref_axis',(-0.866025403784429,0.,0.500000000000017));
#11495=DIRECTION('',(-1.265825400597E-11,-1.,4.163515733621E-12));
#11496=DIRECTION('center_axis',(0.0220021483116849,-0.999116223542966,0.0358144848198564));
#11497=DIRECTION('ref_axis',(-0.999757922609801,-0.0219865712180024,0.000828773196178992));
#11498=DIRECTION('center_axis',(0.,-1.,0.));
#11499=DIRECTION('ref_axis',(-0.866025403784429,0.,0.500000000000017));
#11500=DIRECTION('center_axis',(-1.,0.,0.));
#11501=DIRECTION('ref_axis',(0.,0.,1.));
#11502=DIRECTION('',(1.257132338397E-11,-1.,-1.262436544441E-14));
#11503=DIRECTION('center_axis',(-1.,0.,0.));
#11504=DIRECTION('ref_axis',(0.,0.743887963014959,-0.668304345699963));
#11505=DIRECTION('center_axis',(-1.,0.,0.));
#11506=DIRECTION('ref_axis',(0.,0.998312190093586,-0.0580755637987892));
#11507=DIRECTION('center_axis',(-1.,0.,0.));
#11508=DIRECTION('ref_axis',(0.,0.,1.));
#11509=DIRECTION('',(2.02237243844E-8,-1.,-2.714238573232E-14));
#11510=DIRECTION('center_axis',(-1.,0.,0.));
#11511=DIRECTION('ref_axis',(0.,-0.997449181646666,-0.0713801795486376));
#11512=DIRECTION('center_axis',(-1.,0.,0.));
#11513=DIRECTION('ref_axis',(0.,-0.570342240088595,-0.821407164060993));
#11514=DIRECTION('center_axis',(-1.,0.,0.));
#11515=DIRECTION('ref_axis',(0.,0.,1.));
#11516=DIRECTION('center_axis',(-1.,0.,0.));
#11517=DIRECTION('ref_axis',(0.,-0.743887963015197,0.668304345699697));
#11518=DIRECTION('center_axis',(-1.,0.,0.));
#11519=DIRECTION('ref_axis',(0.,-0.998312190093589,0.0580755637987493));
#11520=DIRECTION('center_axis',(-1.,0.,0.));
#11521=DIRECTION('ref_axis',(0.,0.,1.));
#11522=DIRECTION('',(-2.111258706869E-8,-1.,-6.059695388083E-14));
#11523=DIRECTION('center_axis',(-1.,0.,0.));
#11524=DIRECTION('ref_axis',(0.,0.997449181646666,0.0713801795486376));
#11525=DIRECTION('center_axis',(-1.,0.,0.));
#11526=DIRECTION('ref_axis',(0.,0.57034223781309,0.821407165640985));
#11527=DIRECTION('center_axis',(0.,-1.,0.));
#11528=DIRECTION('ref_axis',(-1.,0.,0.));
#11529=DIRECTION('center_axis',(0.022000557232617,0.999116243244608,-0.035814912623604));
#11530=DIRECTION('ref_axis',(-0.999757957615157,0.0219849728771459,-0.000828946778124254));
#11531=DIRECTION('',(-3.509175205565E-9,-1.,-1.661152348979E-9));
#11532=DIRECTION('center_axis',(9.69425622428E-9,-1.,-1.679094432204E-8));
#11533=DIRECTION('ref_axis',(-1.,-9.69425622428E-9,-2.68179925674151E-24));
#11534=DIRECTION('center_axis',(-0.222676118655611,-0.895355451606744,0.385686351143719));
#11535=DIRECTION('ref_axis',(-0.959639358826226,0.131600370203915,-0.248543041652312));
#11536=DIRECTION('center_axis',(-1.,0.,0.));
#11537=DIRECTION('ref_axis',(0.,0.762967197668601,-0.646437201344201));
#11538=DIRECTION('center_axis',(0.,-0.883720930232564,-0.468014227848781));
#11539=DIRECTION('ref_axis',(0.95964016823036,-0.131620002936973,0.248529520068901));
#11540=DIRECTION('center_axis',(-1.,0.,0.));
#11541=DIRECTION('ref_axis',(0.,0.743887962015906,-0.668304346812006));
#11542=DIRECTION('center_axis',(0.,-0.668304347088608,-0.743887961767409));
#11543=DIRECTION('ref_axis',(1.,-1.2479157085834E-11,1.1211197595737E-11));
#11544=DIRECTION('center_axis',(-0.280818391263604,-0.447274630670207,-0.849168084590413));
#11545=DIRECTION('ref_axis',(0.826864856300596,-0.561948510408893,0.0225473072498959));
#11546=DIRECTION('center_axis',(-1.,0.,0.));
#11547=DIRECTION('ref_axis',(0.,0.751071345860703,0.660221048912402));
#11548=DIRECTION('center_axis',(0.,-0.0713801795485182,-0.997449181646675));
#11549=DIRECTION('ref_axis',(-1.,0.,0.));
#11550=DIRECTION('center_axis',(0.,-0.040042283539229,-0.999197986151375));
#11551=DIRECTION('ref_axis',(-0.826848298356623,0.561973937025615,-0.0225207817068473));
#11552=DIRECTION('center_axis',(-1.,0.,0.));
#11553=DIRECTION('ref_axis',(0.,0.99919819108701,-0.0400371693360804));
#11554=DIRECTION('center_axis',(0.49824937053172,-0.0836077691306534,-0.862993224600135));
#11555=DIRECTION('ref_axis',(-0.866025403784453,-4.30093460845859E-13,-0.499999999999976));
#11556=DIRECTION('center_axis',(0.0439783181580926,0.996474919904308,-0.0714397755713733));
#11557=DIRECTION('ref_axis',(-0.99903248020092,0.043873250862281,-0.00303996091638142));
#11558=DIRECTION('center_axis',(-0.868182440414283,0.000195291349290394,
-0.496245112840005));
#11559=DIRECTION('ref_axis',(0.496237261125393,0.00598072766512104,-0.868166350169922));
#11560=DIRECTION('center_axis',(0.493374800291908,-0.162251348583303,-0.854550060745314));
#11561=DIRECTION('ref_axis',(-0.866025364189605,-1.31083826571125E-8,-0.500000068580258));
#11562=DIRECTION('center_axis',(-0.866025403784429,0.,-0.500000000000017));
#11563=DIRECTION('ref_axis',(-0.500000000000017,0.,0.866025403784429));
#11564=DIRECTION('',(-5.201696206723E-13,-1.,9.013782446814E-13));
#11565=DIRECTION('',(1.873702888582E-8,-1.,1.048002362625E-8));
#11566=DIRECTION('center_axis',(-0.866023526388187,3.03179301675285E-7,
-0.500003251731503));
#11567=DIRECTION('ref_axis',(0.0780807385647998,0.987731781529046,-0.135238034674545));
#11568=DIRECTION('center_axis',(0.866025403784448,1.54730561598205E-14,
0.499999999999983));
#11569=DIRECTION('ref_axis',(0.105564362892848,-0.977458265681004,-0.18284283999903));
#11570=DIRECTION('center_axis',(0.190441801473105,-0.924622993985522,-0.329854876036308));
#11571=DIRECTION('ref_axis',(0.86602540378445,3.8663516832569E-14,0.499999999999981));
#11572=DIRECTION('center_axis',(-1.,0.,0.));
#11573=DIRECTION('ref_axis',(0.,0.,1.));
#11574=DIRECTION('center_axis',(-1.,0.,0.));
#11575=DIRECTION('ref_axis',(0.,-0.743887962015906,-0.668304346812006));
#11576=DIRECTION('center_axis',(-1.,0.,0.));
#11577=DIRECTION('ref_axis',(0.,0.,1.));
#11578=DIRECTION('center_axis',(-1.,0.,0.));
#11579=DIRECTION('ref_axis',(0.,0.743887962015906,0.668304346812006));
#11580=DIRECTION('center_axis',(-1.,0.,0.));
#11581=DIRECTION('ref_axis',(0.,-1.97666424549385E-6,-0.999999999998046));
#11582=DIRECTION('center_axis',(-1.,0.,0.));
#11583=DIRECTION('ref_axis',(0.,0.467970411627219,-0.883744133695636));
#11584=DIRECTION('center_axis',(-1.,0.,0.));
#11585=DIRECTION('ref_axis',(0.,0.,1.));
#11586=DIRECTION('center_axis',(-1.,0.,0.));
#11587=DIRECTION('ref_axis',(0.,-0.467970411624927,0.88374413369685));
#11588=DIRECTION('center_axis',(-1.,0.,0.));
#11589=DIRECTION('ref_axis',(0.,-0.467970411624927,0.88374413369685));
#11590=DIRECTION('center_axis',(0.280781834080107,-0.447280798160512,0.849176924584922));
#11591=DIRECTION('ref_axis',(0.826871614630506,0.561937308806419,0.0225786157622499));
#11592=DIRECTION('center_axis',(0.,-0.040042283539229,0.999197986151375));
#11593=DIRECTION('ref_axis',(-0.826851728368265,-0.561968898410276,-0.0225205797872409));
#11594=DIRECTION('center_axis',(-0.351932310973904,-0.0131675051143801,
0.935932831618611));
#11595=DIRECTION('ref_axis',(6.04805910778599E-8,-0.999901048641168,-0.0140674420663423));
#11596=DIRECTION('center_axis',(0.351932331559598,0.0131675058692799,0.935932823867294));
#11597=DIRECTION('ref_axis',(-5.5740687180029E-6,-0.999901018808378,0.014069561290144));
#11598=DIRECTION('center_axis',(0.,0.040042283539229,0.999197986151375));
#11599=DIRECTION('ref_axis',(-0.826848298356623,-0.561973937025615,0.0225207817068473));
#11600=DIRECTION('center_axis',(-0.280818391263604,0.447274630670207,0.849168084590413));
#11601=DIRECTION('ref_axis',(0.826864856300596,0.561948510408893,-0.0225473072498959));
#11602=DIRECTION('center_axis',(0.,0.668304347090714,0.743887961765516));
#11603=DIRECTION('ref_axis',(1.,1.15056772865253E-11,-1.0336629360903E-11));
#11604=DIRECTION('center_axis',(-1.,0.,0.));
#11605=DIRECTION('ref_axis',(0.,-0.751071345860703,-0.660221048912402));
#11606=DIRECTION('center_axis',(0.,0.0713801795485182,0.997449181646675));
#11607=DIRECTION('ref_axis',(-1.,-2.96023766778491E-14,2.11842668399344E-15));
#11608=DIRECTION('center_axis',(-1.,0.,0.));
#11609=DIRECTION('ref_axis',(0.,-0.99919819108701,0.0400371693360804));
#11610=DIRECTION('center_axis',(0.498249370522803,0.0836077693430705,0.862993224584705));
#11611=DIRECTION('ref_axis',(-0.866025403784456,4.10046996357472E-13,0.49999999999997));
#11612=DIRECTION('center_axis',(0.0439824930033502,-0.99647481566198,0.0714386594263497));
#11613=DIRECTION('ref_axis',(-0.999032296552403,-0.043877321995646,0.00304155547751212));
#11614=DIRECTION('center_axis',(-0.868182440268428,-0.000195293486889366,
0.496245113094338));
#11615=DIRECTION('ref_axis',(0.496235363589393,-0.00662239063405862,0.868162777286375));
#11616=DIRECTION('center_axis',(0.493374794684409,0.162251348872403,0.854550063927915));
#11617=DIRECTION('ref_axis',(-0.866025367369646,1.20499664413301E-8,0.500000063072265));
#11618=DIRECTION('center_axis',(0.999372239295449,0.0354277761876217,0.));
#11619=DIRECTION('ref_axis',(0.,0.,1.));
#11620=DIRECTION('center_axis',(0.,-1.,0.));
#11621=DIRECTION('ref_axis',(0.,0.,1.));
#11622=DIRECTION('',(1.38025161653E-12,-1.,0.));
#11623=DIRECTION('center_axis',(-0.999372239543964,0.0354277691772887,4.01641479363486E-8));
#11624=DIRECTION('ref_axis',(4.01406338457382E-8,-1.37498900862607E-9,0.999999999999999));
#11625=DIRECTION('center_axis',(-0.493374730482818,0.162251352179406,-0.854550100366831));
#11626=DIRECTION('ref_axis',(-0.866025403784436,2.20656826144257E-15,0.500000000000005));
#11627=DIRECTION('center_axis',(-0.498249373922926,0.0836076882921444,-0.862993230473945));
#11628=DIRECTION('ref_axis',(-0.866025403784452,3.85108611666864E-15,0.499999999999977));
#11629=DIRECTION('center_axis',(-0.868182476504346,0.000194770775834953,
0.496245049904909));
#11630=DIRECTION('ref_axis',(0.496242860058454,0.00333736388693019,0.868177335481232));
#11631=DIRECTION('center_axis',(0.,0.0713801892709608,-0.99744918095091));
#11632=DIRECTION('ref_axis',(-1.,1.59057546106842E-14,1.1382592680318E-15));
#11633=DIRECTION('center_axis',(0.0220023491734484,0.9991162207134,0.0358144403589185));
#11634=DIRECTION('ref_axis',(-0.865987807571244,0.00114527309927654,0.500063801416858));
#11635=DIRECTION('center_axis',(0.043979209247116,0.996474897810047,0.0714395351920356));
#11636=DIRECTION('ref_axis',(-0.868223079665157,0.00274755012920933,0.496166438712896));
#11637=DIRECTION('center_axis',(-1.,0.,0.));
#11638=DIRECTION('ref_axis',(0.,0.751071345860703,0.660221048912402));
#11639=DIRECTION('center_axis',(-1.,0.,0.));
#11640=DIRECTION('ref_axis',(0.,0.997449180243098,0.0713801991617598));
#11641=DIRECTION('center_axis',(0.,0.040042283539229,-0.999197986151375));
#11642=DIRECTION('ref_axis',(-0.826851728368265,0.561968898410276,0.0225205797872409));
#11643=DIRECTION('center_axis',(0.280781834080107,0.447280798160512,-0.849176924584922));
#11644=DIRECTION('ref_axis',(0.826871614630508,-0.561937308806416,-0.0225786157622471));
#11645=DIRECTION('center_axis',(7.29309508193181E-7,0.668304022744483,-0.743888253155681));
#11646=DIRECTION('ref_axis',(0.999999999999734,-4.87417910926425E-7,5.42509114576228E-7));
#11647=DIRECTION('center_axis',(-1.,0.,0.));
#11648=DIRECTION('ref_axis',(0.,-0.99999889596136,0.00148595964285994));
#11649=DIRECTION('center_axis',(-1.,0.,0.));
#11650=DIRECTION('ref_axis',(0.,0.468006113503988,0.883725227501678));
#11651=DIRECTION('center_axis',(0.,0.883720930238071,-0.468014227838384));
#11652=DIRECTION('ref_axis',(0.959631287113083,-0.131634185239414,-0.248556299598387));
#11653=DIRECTION('center_axis',(9.559147147985E-9,-1.,1.655692853734E-8));
#11654=DIRECTION('ref_axis',(-0.866025403784429,1.79498192924013E-21,0.500000000000017));
#11655=DIRECTION('center_axis',(-0.222723179217891,-0.895308629331963,-0.385767862428684));
#11656=DIRECTION('ref_axis',(-0.86602540376781,-1.65629454595974E-11,0.500000000028802));
#11657=DIRECTION('center_axis',(-0.190441695445105,0.924622974493123,-0.329854991891108));
#11658=DIRECTION('ref_axis',(0.866025432288796,-1.38474408523102E-7,-0.499999950628983));
#11659=DIRECTION('center_axis',(1.8985766484E-10,1.,3.288431217093E-10));
#11660=DIRECTION('ref_axis',(0.866025403784429,2.57201471715716E-23,-0.500000000000017));
#11661=DIRECTION('center_axis',(0.19044180147329,0.92462299398535,0.329854876036682));
#11662=DIRECTION('ref_axis',(0.866025403784455,-1.38777878078137E-14,-0.499999999999972));
#11663=DIRECTION('center_axis',(0.,0.883720930232564,0.468014227848781));
#11664=DIRECTION('ref_axis',(0.959640168230617,0.131620002936562,-0.248529520068125));
#11665=DIRECTION('center_axis',(0.222676472654806,-0.895355099446026,0.385686964288411));
#11666=DIRECTION('ref_axis',(-0.866025536407818,-1.31934723174299E-7,0.49999977028948));
#11667=DIRECTION('center_axis',(-1.,0.,0.));
#11668=DIRECTION('ref_axis',(0.,-0.762644877891583,0.646817431912385));
#11669=DIRECTION('center_axis',(-1.,0.,0.));
#11670=DIRECTION('ref_axis',(0.,-0.743887962015906,0.668304346812006));
#11671=DIRECTION('center_axis',(-1.,0.,0.));
#11672=DIRECTION('ref_axis',(0.,0.0098807139151359,-0.99995118455479));
#11673=DIRECTION('center_axis',(-1.,0.,0.));
#11674=DIRECTION('ref_axis',(0.,0.,-1.));
#11675=DIRECTION('center_axis',(0.,0.99995118455479,0.00988071391513576));
#11676=DIRECTION('ref_axis',(0.,-0.00988071391513575,0.99995118455479));
#11677=DIRECTION('center_axis',(-1.,0.,0.));
#11678=DIRECTION('ref_axis',(0.,-0.468018161851774,-0.883718846792851));
#11679=DIRECTION('center_axis',(-1.,0.,0.));
#11680=DIRECTION('ref_axis',(0.,0.99999889596136,-0.00148595964285994));
#11681=DIRECTION('center_axis',(7.29307587577525E-7,-0.668304022745323,
0.743888253154926));
#11682=DIRECTION('ref_axis',(0.999999999999734,4.87415776280581E-7,-5.42508450466735E-7));
#11683=DIRECTION('center_axis',(0.,-0.883720930238698,0.468014227837199));
#11684=DIRECTION('ref_axis',(0.959631287109364,0.131634185245019,0.248556299609778));
#11685=DIRECTION('center_axis',(0.222725367331005,-0.895306451997919,-0.385771652351708));
#11686=DIRECTION('ref_axis',(-0.959634003928859,-0.131634145854039,-0.248545831083011));
#11687=DIRECTION('center_axis',(0.,-1.,0.));
#11688=DIRECTION('ref_axis',(-1.,0.,0.));
#11689=DIRECTION('center_axis',(0.,-1.,0.));
#11690=DIRECTION('ref_axis',(-1.,0.,0.));
#11691=DIRECTION('center_axis',(0.0220020309913136,-0.999116224741113,-0.0358145234691645));
#11692=DIRECTION('ref_axis',(-0.865987846623121,-0.00114495897030132,-0.500063734507918));
#11693=DIRECTION('center_axis',(0.,-0.0713801877643918,0.997449181058724));
#11694=DIRECTION('ref_axis',(-1.,-2.91605501258917E-14,-2.08680861423913E-15));
#11695=DIRECTION('center_axis',(-0.498249373968018,-0.083607687218453,0.862993230551932));
#11696=DIRECTION('ref_axis',(-0.866025403784423,9.78384040450952E-16,-0.500000000000027));
#11697=DIRECTION('center_axis',(0.0439792054831152,-0.996474897881974,-0.071439536505943));
#11698=DIRECTION('ref_axis',(-0.868223086749888,-0.00274754739562432,-0.496166426330727));
#11699=DIRECTION('center_axis',(-1.,0.,0.));
#11700=DIRECTION('ref_axis',(0.,-0.751071345860703,-0.660221048912402));
#11701=DIRECTION('center_axis',(-1.,0.,0.));
#11702=DIRECTION('ref_axis',(0.,-0.997449180276294,-0.0713801986978796));
#11703=DIRECTION('center_axis',(-1.,0.,0.));
#11704=DIRECTION('ref_axis',(0.,0.,1.));
#11705=DIRECTION('center_axis',(-0.868182476775313,-0.000194768429474923,
-0.496245049431772));
#11706=DIRECTION('ref_axis',(0.496245087391322,-0.000373257433497943,-0.86818239668797));
#11707=DIRECTION('',(-0.999371785786445,-0.0354405142272462,6.10354031209678E-5));
#11708=DIRECTION('',(0.999371785786445,0.0354405142272462,6.10354031209678E-5));
#11709=DIRECTION('',(0.999372166129595,0.0354298400425457,0.));
#11710=DIRECTION('center_axis',(0.999372092799054,0.0354319084221984,-2.05236350338391E-8));
#11711=DIRECTION('ref_axis',(2.05104383127819E-8,7.35929113883462E-10,1.));
#11712=DIRECTION('center_axis',(0.,0.,1.));
#11713=DIRECTION('ref_axis',(1.,0.,0.));
#11714=DIRECTION('',(-0.999372166129596,0.0354298400425258,0.));
#11715=DIRECTION('',(7.743978635044E-13,-1.,0.));
#11716=DIRECTION('center_axis',(-0.999372092671549,0.0354319120185417,0.));
#11717=DIRECTION('ref_axis',(0.,0.,1.));
#11718=DIRECTION('',(-0.999371785786448,0.0354405142271533,-6.1035403120968E-5));
#11719=DIRECTION('center_axis',(-1.,0.,0.));
#11720=DIRECTION('ref_axis',(0.,0.,1.));
#11721=DIRECTION('',(0.999371785786448,-0.0354405142271533,-6.1035403120968E-5));
#11722=DIRECTION('center_axis',(0.999372239295449,-0.0354277761876217,0.));
#11723=DIRECTION('ref_axis',(0.,0.,-1.));
#11724=DIRECTION('center_axis',(0.,-1.,0.));
#11725=DIRECTION('ref_axis',(-0.866025403784429,0.,-0.500000000000017));
#11726=DIRECTION('',(-1.111343038653E-12,-1.,0.));
#11727=DIRECTION('center_axis',(-0.999372239506482,-0.0354277702346294,
-3.41063282467894E-8));
#11728=DIRECTION('ref_axis',(3.40863636314234E-8,1.16752162350377E-9,-0.999999999999999));
#11729=DIRECTION('center_axis',(-0.493374730482899,-0.1622513521788,0.854550100366899));
#11730=DIRECTION('ref_axis',(-0.866025403784418,3.73312492030221E-15,-0.500000000000036));
#11731=DIRECTION('',(-0.9993721661296,-0.0354298400424142,0.));
#11732=DIRECTION('center_axis',(-0.999372092671548,-0.0354319120185517,
0.));
#11733=DIRECTION('ref_axis',(0.,0.,-1.));
#11734=DIRECTION('center_axis',(0.,0.,-1.));
#11735=DIRECTION('ref_axis',(-1.,0.,0.));
#11736=DIRECTION('',(0.9993721661296,-0.0354298400424206,0.));
#11737=DIRECTION('',(-8.842919962527E-13,-1.,0.));
#11738=DIRECTION('center_axis',(0.999372092820432,-0.0354319078192211,2.39647906652608E-8));
#11739=DIRECTION('ref_axis',(2.39493900704611E-8,-8.59072814438014E-10,
-1.));
#11740=DIRECTION('center_axis',(0.737263762925204,0.0895414080136305,0.669645040397004));
#11741=DIRECTION('ref_axis',(0.672345785926011,2.4021409861242E-12,-0.740237221536133));
#11742=DIRECTION('center_axis',(0.,-1.,0.));
#11743=DIRECTION('ref_axis',(0.,0.,-1.));
#11744=DIRECTION('',(-4.095605011303E-13,-1.,-3.717912330146E-13));
#11745=DIRECTION('center_axis',(-0.737263807819715,0.0895413984213018,-0.669644992251814));
#11746=DIRECTION('ref_axis',(0.672345737398719,5.92140809302375E-9,-0.740237265612704));
#11747=DIRECTION('center_axis',(0.737263762924105,-0.0895414080137006,-0.669645040398205));
#11748=DIRECTION('ref_axis',(0.672345785927211,-2.55426235717958E-12,0.740237221535044));
#11749=DIRECTION('center_axis',(0.,1.,0.));
#11750=DIRECTION('ref_axis',(1.,0.,0.));
#11751=DIRECTION('',(4.642472539228E-13,-1.,-4.217568272926E-13));
#11752=DIRECTION('center_axis',(-1.,0.,0.));
#11753=DIRECTION('ref_axis',(0.,1.,0.));
#11754=DIRECTION('center_axis',(-1.,0.,0.));
#11755=DIRECTION('ref_axis',(0.,1.,0.));
#11756=DIRECTION('center_axis',(-1.,0.,0.));
#11757=DIRECTION('ref_axis',(0.,1.,0.));
#11758=DIRECTION('center_axis',(-1.,0.,0.));
#11759=DIRECTION('ref_axis',(0.,-1.,1.22464679914735E-16));
#11760=DIRECTION('center_axis',(1.,0.,0.));
#11761=DIRECTION('ref_axis',(0.,-0.554308231206715,0.832311471035023));
#11762=DIRECTION('center_axis',(1.,0.,0.));
#11763=DIRECTION('ref_axis',(0.,-1.,0.));
#11764=DIRECTION('center_axis',(-1.,0.,0.));
#11765=DIRECTION('ref_axis',(0.,1.,0.));
#11766=DIRECTION('',(0.707106781186547,0.707106781186547,8.65956056235493E-17));
#11767=DIRECTION('center_axis',(-1.,0.,0.));
#11768=DIRECTION('ref_axis',(0.,1.,0.));
#11769=DIRECTION('center_axis',(-1.,0.,0.));
#11770=DIRECTION('ref_axis',(0.,1.,0.));
#11771=DIRECTION('',(-1.,0.,0.));
#11772=DIRECTION('center_axis',(-1.,0.,0.));
#11773=DIRECTION('ref_axis',(0.,-1.,0.));
#11774=DIRECTION('center_axis',(-1.,0.,0.));
#11775=DIRECTION('ref_axis',(0.,0.,1.));
#11776=DIRECTION('center_axis',(-1.,0.,0.));
#11777=DIRECTION('ref_axis',(0.,0.,1.));
#11778=DIRECTION('center_axis',(-1.,0.,0.));
#11779=DIRECTION('ref_axis',(0.,0.,1.));
#11780=DIRECTION('',(-1.,0.,0.));
#11781=DIRECTION('center_axis',(-1.,0.,0.));
#11782=DIRECTION('ref_axis',(0.,0.,1.));
#11783=DIRECTION('center_axis',(-1.,0.,0.));
#11784=DIRECTION('ref_axis',(0.,0.,1.));
#11785=DIRECTION('center_axis',(-0.737263813887754,-0.0895413971243944,
0.669644985744458));
#11786=DIRECTION('ref_axis',(0.672345730839688,-6.72198713358419E-9,0.740237271570168));
#11787=DIRECTION('center_axis',(0.,-1.,0.));
#11788=DIRECTION('ref_axis',(0.672345785906318,0.,0.74023722155402));
#11789=DIRECTION('center_axis',(-0.351932310972217,0.0131675051143506,-0.935932831619245));
#11790=DIRECTION('ref_axis',(6.04805859916508E-8,0.999901048641168,0.0140674420663031));
#11791=DIRECTION('center_axis',(0.351932331559182,-0.0131675058692493,-0.935932823867451));
#11792=DIRECTION('ref_axis',(-5.57406870898581E-6,0.999901018808379,-0.0140695612901056));
#11793=DIRECTION('center_axis',(-0.190441695445105,-0.924622974493123,0.329854991891108));
#11794=DIRECTION('ref_axis',(0.866025432288782,1.38474419875132E-7,0.499999950629006));
#11795=DIRECTION('center_axis',(1.899754571623E-10,-1.,-3.290471439962E-10));
#11796=DIRECTION('ref_axis',(0.866025403784429,6.82424005356271E-24,0.500000000000017));
#11797=DIRECTION('center_axis',(0.,-1.,0.));
#11798=DIRECTION('ref_axis',(-0.866025403784429,0.,0.500000000000017));
#29276=CARTESIAN_POINT('',(0.,0.,0.));
#29277=CARTESIAN_POINT('Origin',(0.,0.,3.8));
#29278=CARTESIAN_POINT('',(0.133974596216,1.34752837055,4.03205080757));
#29279=CARTESIAN_POINT('',(0.133975838235341,0.664859028439009,4.03205295596885));
#29280=CARTESIAN_POINT('',(0.133974596216,1.34752837055,4.03205080757));
#29281=CARTESIAN_POINT('',(2.71354627738384,1.30409337481055,8.50000002111664));
#29282=CARTESIAN_POINT('Ctrl Pts',(0.133975839160916,0.664858977042815,
4.03205296041379));
#29283=CARTESIAN_POINT('Ctrl Pts',(0.247132282736217,0.683846965301094,
4.22804566988996));
#29284=CARTESIAN_POINT('Ctrl Pts',(0.36075899558286,0.704110746029599,4.42485290926822));
#29285=CARTESIAN_POINT('Ctrl Pts',(0.47425093097406,0.725533099101974,4.621426707294));
#29286=CARTESIAN_POINT('Ctrl Pts',(0.561430823810993,0.741988880199786,
4.77242671083931));
#29287=CARTESIAN_POINT('Ctrl Pts',(0.648531228319088,0.759127295663591,
4.92328903774398));
#29288=CARTESIAN_POINT('Ctrl Pts',(0.735278965462407,0.77687530163016,5.07354052591786));
#29289=CARTESIAN_POINT('Ctrl Pts',(0.821592229549516,0.794534417319612,
5.22303948468387));
#29290=CARTESIAN_POINT('Ctrl Pts',(0.907554962852823,0.812822098130855,
5.37193130515576));
#29291=CARTESIAN_POINT('Ctrl Pts',(0.993977273034051,0.831907903641516,
5.52161913744188));
#29292=CARTESIAN_POINT('Ctrl Pts',(1.04856084276224,0.843962330255724,5.61616065356101));
#29293=CARTESIAN_POINT('Ctrl Pts',(1.1033276922141,0.85633615357053,5.71101961970344));
#29294=CARTESIAN_POINT('Ctrl Pts',(1.15848133271126,0.869082750270139,5.80654852750131));
#29295=CARTESIAN_POINT('Ctrl Pts',(1.2180206215764,0.882842917252854,5.90967360111531));
#29296=CARTESIAN_POINT('Ctrl Pts',(1.27801067445639,0.897037334625361,6.01357942077414));
#29297=CARTESIAN_POINT('Ctrl Pts',(1.3387068707796,0.91174429412865,6.11870831663208));
#29298=CARTESIAN_POINT('Ctrl Pts',(1.43336285608852,0.934679862203939,6.28265729242754));
#29299=CARTESIAN_POINT('Ctrl Pts',(1.52973609727286,0.958853710900147,6.44958064268732));
#29300=CARTESIAN_POINT('Ctrl Pts',(1.62843729109613,0.984543986523405,6.62053612509274));
#29301=CARTESIAN_POINT('Ctrl Pts',(1.71302174746797,1.00655991068261,6.76704070100435));
#29302=CARTESIAN_POINT('Ctrl Pts',(1.79931583017353,1.02969013216229,6.91650643650829));
#29303=CARTESIAN_POINT('Ctrl Pts',(1.8877011757851,1.05413975161752,7.06959434585853));
#29304=CARTESIAN_POINT('Ctrl Pts',(1.92057356758229,1.06323308563645,7.12653099865718));
#29305=CARTESIAN_POINT('Ctrl Pts',(1.95373520706313,1.07250921588961,7.18396864316921));
#29306=CARTESIAN_POINT('Ctrl Pts',(1.98720558499433,1.08197974195953,7.24194103829456));
#29307=CARTESIAN_POINT('Ctrl Pts',(2.1539401013221,1.12915768500172,7.53073369194964));
#29308=CARTESIAN_POINT('Ctrl Pts',(2.32834097569438,1.18110458813524,7.83280486711957));
#29309=CARTESIAN_POINT('Ctrl Pts',(2.50952487075871,1.2383290506724,8.14662457897929));
#29310=CARTESIAN_POINT('Ctrl Pts',(2.5766171014717,1.25951921683814,8.26283173140252));
#29311=CARTESIAN_POINT('Ctrl Pts',(2.64463931462142,1.28143262361183,8.38064966061838));
#29312=CARTESIAN_POINT('Ctrl Pts',(2.71354626506708,1.304093369936,8.49999999978495));
#29313=CARTESIAN_POINT('',(2.713546265065,6.295906630064,8.499999999781));
#29314=CARTESIAN_POINT('',(2.713546265065,6.295906630064,8.499999999781));
#29315=CARTESIAN_POINT('',(0.133974546587078,6.93514124142996,4.03205068645143));
#29316=CARTESIAN_POINT('Ctrl Pts',(2.71354626506511,6.295906630064,8.49999999978094));
#29317=CARTESIAN_POINT('Ctrl Pts',(2.61139186763909,6.32950114282925,8.32306339322283));
#29318=CARTESIAN_POINT('Ctrl Pts',(2.50870084894661,6.36224673356896,8.14519733060976));
#29319=CARTESIAN_POINT('Ctrl Pts',(2.40615912187201,6.3939534451709,7.96758984811973));
#29320=CARTESIAN_POINT('Ctrl Pts',(2.3086542390515,6.42410272476244,7.79870643585148));
#29321=CARTESIAN_POINT('Ctrl Pts',(2.21128440432946,6.4533130808905,7.63005693828328));
#29322=CARTESIAN_POINT('Ctrl Pts',(2.11464207311449,6.48146460959975,7.46266751045704));
#29323=CARTESIAN_POINT('Ctrl Pts',(2.09163285950551,6.48816710248612,7.42281438344407));
#29324=CARTESIAN_POINT('Ctrl Pts',(2.06866466968897,6.49480642163638,7.38303231116932));
#29325=CARTESIAN_POINT('Ctrl Pts',(2.04571368948606,6.50138989845776,7.34328004662047));
#29326=CARTESIAN_POINT('Ctrl Pts',(1.96873400784639,6.52347148039071,7.20994732434137));
#29327=CARTESIAN_POINT('Ctrl Pts',(1.89194820262661,6.54492874953572,7.07695040454043));
#29328=CARTESIAN_POINT('Ctrl Pts',(1.81445492386495,6.56600503948902,6.94272810863974));
#29329=CARTESIAN_POINT('Ctrl Pts',(1.73791067961232,6.5868232151025,6.81014958872486));
#29330=CARTESIAN_POINT('Ctrl Pts',(1.66067615707177,6.60726972394034,6.67637547553564));
#29331=CARTESIAN_POINT('Ctrl Pts',(1.58187949656786,6.62752885128245,6.53989565838102));
#29332=CARTESIAN_POINT('Ctrl Pts',(1.55928046578883,6.63333920719643,6.50075298953098));
#29333=CARTESIAN_POINT('Ctrl Pts',(1.53655292167311,6.63913382699167,6.46138772885641));
#29334=CARTESIAN_POINT('Ctrl Pts',(1.51367625064916,6.64491626389417,6.42176417233491));
#29335=CARTESIAN_POINT('Ctrl Pts',(1.46609117940512,6.65694413594258,6.33934441125846));
#29336=CARTESIAN_POINT('Ctrl Pts',(1.417861702161,6.66892999551049,6.25580850454491));
#29337=CARTESIAN_POINT('Ctrl Pts',(1.36900976236698,6.68084982723003,6.17119446184299));
#29338=CARTESIAN_POINT('Ctrl Pts',(1.21594957699074,6.7181963821537,5.9060864412404));
#29339=CARTESIAN_POINT('Ctrl Pts',(1.05677805398043,6.75489136322574,5.63039328136468));
#29340=CARTESIAN_POINT('Ctrl Pts',(0.892178373440007,6.79022340698429,5.34529827216908));
#29341=CARTESIAN_POINT('Ctrl Pts',(0.880260159593054,6.79278170388852,5.32465532028037));
#29342=CARTESIAN_POINT('Ctrl Pts',(0.86831349204015,6.79533287580036,5.30396308511113));
#29343=CARTESIAN_POINT('Ctrl Pts',(0.856338632539872,6.79787666269458,5.28322202004314));
#29344=CARTESIAN_POINT('Ctrl Pts',(0.777345203864997,6.81465702229612,5.14640138811414));
#29345=CARTESIAN_POINT('Ctrl Pts',(0.697124668072234,6.83111225314263,5.00745534397502));
#29346=CARTESIAN_POINT('Ctrl Pts',(0.615648984965793,6.84719804282709,4.86633532126311));
#29347=CARTESIAN_POINT('Ctrl Pts',(0.459751271772893,6.87797701553522,4.59631256124802));
#29348=CARTESIAN_POINT('Ctrl Pts',(0.299258018817764,6.90740619144373,4.31833009316456));
#29349=CARTESIAN_POINT('Ctrl Pts',(0.133974596321897,6.935141228052,4.03205080775324));
#29350=CARTESIAN_POINT('',(0.133974596215585,6.25247165111742,4.03205080756906));
#29351=CARTESIAN_POINT('',(0.1339746084865,6.935141228052,4.03205080073));
#29352=CARTESIAN_POINT('',(0.0734244918642833,5.61500841690498,3.92717512466558));
#29353=CARTESIAN_POINT('Ctrl Pts',(0.1339745962156,6.252471629351,4.032050807569));
#29354=CARTESIAN_POINT('Ctrl Pts',(0.1339743516313,6.210070040294,4.032050175084));
#29355=CARTESIAN_POINT('Ctrl Pts',(0.1327751855236,6.126676439139,4.029973442397));
#29356=CARTESIAN_POINT('Ctrl Pts',(0.1277364860869,6.010122770097,4.021246134362));
#29357=CARTESIAN_POINT('Ctrl Pts',(0.1185452327114,5.889181793142,4.005326089051));
#29358=CARTESIAN_POINT('Ctrl Pts',(0.103261617757799,5.76029299121146,3.97885542594176));
#29359=CARTESIAN_POINT('Ctrl Pts',(0.0855624395784293,5.66383148718846,
3.94819620974927));
#29360=CARTESIAN_POINT('Ctrl Pts',(0.0734243412793448,5.61500841659961,
3.92717521231643));
#29361=CARTESIAN_POINT('',(-1.29316404762894E-8,5.24481852459253,3.79999997760173));
#29362=CARTESIAN_POINT('Origin',(-0.198918003246391,2.40959514383602,3.4554639118384));
#29363=CARTESIAN_POINT('',(0.14433756729743,3.79999999952898,4.04999999999999));
#29364=CARTESIAN_POINT('Ctrl Pts',(0.1443375672974,3.800000000001,4.05));
#29365=CARTESIAN_POINT('Ctrl Pts',(0.1443378984973,3.958261403905,4.050000359522));
#29366=CARTESIAN_POINT('Ctrl Pts',(0.1338012341637,4.276090778539,4.031750623427));
#29367=CARTESIAN_POINT('Ctrl Pts',(0.09119037446517,4.728509036729,3.957946375843));
#29368=CARTESIAN_POINT('Ctrl Pts',(0.03592510445712,5.070395215176,3.862224014774));
#29369=CARTESIAN_POINT('Ctrl Pts',(1.940766991559E-12,5.24481832766,3.800000000003));
#29370=CARTESIAN_POINT('',(3.386874111916E-13,2.355181672324,3.800000000001));
#29371=CARTESIAN_POINT('Ctrl Pts',(3.386874111916E-13,2.355181672324,3.800000000001));
#29372=CARTESIAN_POINT('Ctrl Pts',(0.03068797257625,2.504173780267,3.853152901811));
#29373=CARTESIAN_POINT('Ctrl Pts',(0.08231078075842,2.809566709961,3.942566526949));
#29374=CARTESIAN_POINT('Ctrl Pts',(0.1295382484853,3.25413134046,4.024366912382));
#29375=CARTESIAN_POINT('Ctrl Pts',(0.1443374905,3.61171344699,4.049999621415));
#29376=CARTESIAN_POINT('Ctrl Pts',(0.1443375672974,3.800000000001,4.05));
#29377=CARTESIAN_POINT('',(0.0734360006991422,1.98494851950308,3.92719616078412));
#29378=CARTESIAN_POINT('Origin',(-0.0267630005725188,2.98738908516278,3.75364512324667));
#29379=CARTESIAN_POINT('Ctrl Pts',(0.0734361377817803,1.98494851831011,
3.92719607885935));
#29380=CARTESIAN_POINT('Ctrl Pts',(0.0844284068963691,1.94072397567073,
3.94623216194698));
#29381=CARTESIAN_POINT('Ctrl Pts',(0.102287144414616,1.84748240172733,3.97716748379283));
#29382=CARTESIAN_POINT('Ctrl Pts',(0.119996932845,1.700515755579,4.007840642711));
#29383=CARTESIAN_POINT('Ctrl Pts',(0.1311959657202,1.536687730076,4.027237692571));
#29384=CARTESIAN_POINT('Ctrl Pts',(0.1339757766234,1.412832779138,4.03205384679));
#29385=CARTESIAN_POINT('Ctrl Pts',(0.133974596216,1.34752837055,4.03205080757));
#29386=CARTESIAN_POINT('Origin',(1.,6.995321512442,3.532050807569));
#29387=CARTESIAN_POINT('',(1.66253962058448E-16,1.34752836921872,3.53205080731726));
#29388=CARTESIAN_POINT('',(-8.905626236455E-12,0.6439853496971,3.532050807569));
#29389=CARTESIAN_POINT('',(0.,1.347528368525,3.532050807566));
#29390=CARTESIAN_POINT('Origin',(1.00129300833713,0.666005680359366,3.53122076182685));
#29391=CARTESIAN_POINT('Origin',(1.,1.347528370609,3.532050807569));
#29392=CARTESIAN_POINT('Origin',(0.,0.,-3.8));
#29393=CARTESIAN_POINT('',(-8.844466825586E-12,6.956014650303,-3.532050807569));
#29394=CARTESIAN_POINT('',(-2.12915400332963E-17,6.25247164440103,-3.5320508052874));
#29395=CARTESIAN_POINT('',(-8.844466825586E-12,6.956014650303,-3.532050807569));
#29396=CARTESIAN_POINT('',(3.29873385069466E-15,6.99871823693242,-2.87370869095006));
#29397=CARTESIAN_POINT('Origin',(0.,3.8,0.));
#29398=CARTESIAN_POINT('Origin',(0.,-42.4,0.));
#29399=CARTESIAN_POINT('Origin',(0.,0.,-3.8));
#29400=CARTESIAN_POINT('',(0.,1.34752836990142,-3.53205080743734));
#29401=CARTESIAN_POINT('',(3.55903513595825E-9,0.643985367713358,-3.53205101022315));
#29402=CARTESIAN_POINT('',(0.,1.347528369529,-3.532050807569));
#29403=CARTESIAN_POINT('',(2.73760181190852E-12,0.601281259440645,-2.87370767806568));
#29404=CARTESIAN_POINT('Origin',(0.,50.,0.));
#29405=CARTESIAN_POINT('Origin',(0.,3.8,0.));
#29406=CARTESIAN_POINT('Origin',(0.,0.,-3.8));
#29407=CARTESIAN_POINT('',(3.27721772858058E-15,0.601281763069545,2.87370869095238));
#29408=CARTESIAN_POINT('Origin',(0.,3.8,0.));
#29409=CARTESIAN_POINT('Origin',(0.,50.,0.));
#29410=CARTESIAN_POINT('Origin',(0.,0.,-3.8));
#29411=CARTESIAN_POINT('',(1.90152351602403E-8,6.95601462898345,3.5320510473839));
#29412=CARTESIAN_POINT('',(3.5763139446717E-16,6.25247164282405,3.53205080558666));
#29413=CARTESIAN_POINT('',(1.485361333931E-8,6.956014650303,3.532050807569));
#29414=CARTESIAN_POINT('',(2.73760181190852E-12,6.99871874056045,2.87370767806342));
#29415=CARTESIAN_POINT('Origin',(0.,-42.4,0.));
#29416=CARTESIAN_POINT('Origin',(0.,3.8,0.));
#29417=CARTESIAN_POINT('Origin',(1.,18.3911851122,-3.532050807569));
#29418=CARTESIAN_POINT('',(0.133975834635972,6.93514097197305,-4.0320529499034));
#29419=CARTESIAN_POINT('Origin',(1.00129390752562,6.93399590143332,-3.53122058726189));
#29420=CARTESIAN_POINT('',(0.133974596215514,6.25247165142154,-4.032050807569));
#29421=CARTESIAN_POINT('',(0.1339745986111,6.935141231182,-4.032050806435));
#29422=CARTESIAN_POINT('Origin',(1.,6.25247167405,-3.532050807569));
#29423=CARTESIAN_POINT('Ctrl Pts',(0.0005956539577002,6.267381300312,-3.496598976845));
#29424=CARTESIAN_POINT('Ctrl Pts',(0.0005454737658584,6.26241504239,-3.498634307646));
#29425=CARTESIAN_POINT('Ctrl Pts',(0.0001990202063126,6.230880706393,-3.511470929608));
#29426=CARTESIAN_POINT('Ctrl Pts',(-0.0007621112943634,6.173196747509,-3.533936979622));
#29427=CARTESIAN_POINT('Ctrl Pts',(-0.002892090579078,6.094032006508,-3.562357810308));
#29428=CARTESIAN_POINT('Ctrl Pts',(-0.00592218410683,6.014627167998,-3.588339308072));
#29429=CARTESIAN_POINT('Ctrl Pts',(-0.01012911618744,5.932736633387,-3.612262577613));
#29430=CARTESIAN_POINT('Ctrl Pts',(-0.01606034386805,5.845994028826,-3.633968305936));
#29431=CARTESIAN_POINT('Ctrl Pts',(-0.02193414995839,5.783303687288,-3.646093985463));
#29432=CARTESIAN_POINT('Ctrl Pts',(-0.02585027170663,5.750191401094,-3.650825051518));
#29433=CARTESIAN_POINT('Ctrl Pts',(-0.02638515003392,5.745804308856,-3.651418389814));
#29434=CARTESIAN_POINT('Ctrl Pts',(-0.006377801946632,6.26876976599,-3.693389523142));
#29435=CARTESIAN_POINT('Ctrl Pts',(-0.006032302342462,6.263345873378,-3.695442025085));
#29436=CARTESIAN_POINT('Ctrl Pts',(-0.003867291976553,6.228875461554,-3.708370566011));
#29437=CARTESIAN_POINT('Ctrl Pts',(-0.0002451597187239,6.165452133895,-3.730795665578));
#29438=CARTESIAN_POINT('Ctrl Pts',(0.003860634442441,6.077325338663,-3.758560483081));
#29439=CARTESIAN_POINT('Ctrl Pts',(0.00697153741604,5.987496073211,-3.783097616472));
#29440=CARTESIAN_POINT('Ctrl Pts',(0.008854436988706,5.892748574972,-3.804363708712));
#29441=CARTESIAN_POINT('Ctrl Pts',(0.008764742844783,5.788862659501,-3.821183298427));
#29442=CARTESIAN_POINT('Ctrl Pts',(0.005993463682357,5.709109095087,-3.826759357469));
#29443=CARTESIAN_POINT('Ctrl Pts',(0.002559975292538,5.66404914375,-3.825622482226));
#29444=CARTESIAN_POINT('Ctrl Pts',(0.002062518958956,5.658019058761,-3.825389338686));
#29445=CARTESIAN_POINT('Ctrl Pts',(0.04343955716361,6.270349119306,-3.88389624378));
#29446=CARTESIAN_POINT('Ctrl Pts',(0.04416842517361,6.26440357571,-3.885852742728));
#29447=CARTESIAN_POINT('Ctrl Pts',(0.0487635922003,6.226593348799,-3.898152002359));
#29448=CARTESIAN_POINT('Ctrl Pts',(0.05678337425826,6.156724067586,-3.919186369339));
#29449=CARTESIAN_POINT('Ctrl Pts',(0.0667793086814,6.058741282577,-3.944363515824));
#29450=CARTESIAN_POINT('Ctrl Pts',(0.0755852569517,5.95766968524,-3.965426912709));
#29451=CARTESIAN_POINT('Ctrl Pts',(0.08297966657217,5.849310626945,-3.981825631411));
#29452=CARTESIAN_POINT('Ctrl Pts',(0.08796210861139,5.727591585706,-3.991250184282));
#29453=CARTESIAN_POINT('Ctrl Pts',(0.08757643356987,5.630384339256,-3.988276144813));
#29454=CARTESIAN_POINT('Ctrl Pts',(0.08417413305102,5.573211510378,-3.980120686141));
#29455=CARTESIAN_POINT('Ctrl Pts',(0.08365291538563,5.56551734014,-3.978906690537));
#29456=CARTESIAN_POINT('Ctrl Pts',(0.1458535053006,6.271986391254,-4.052079985885));
#29457=CARTESIAN_POINT('Ctrl Pts',(0.1469211537512,6.265499099249,-4.053835390391));
#29458=CARTESIAN_POINT('Ctrl Pts',(0.1536605702835,6.224226503898,-4.064837148956));
#29459=CARTESIAN_POINT('Ctrl Pts',(0.1655221409961,6.147747382447,-4.083248089847));
#29460=CARTESIAN_POINT('Ctrl Pts',(0.1805666794667,6.039844468178,-4.104123768826));
#29461=CARTESIAN_POINT('Ctrl Pts',(0.1941422442452,5.927659149072,-4.119976518101));
#29462=CARTESIAN_POINT('Ctrl Pts',(0.2060058169343,5.806079919546,-4.129707461221));
#29463=CARTESIAN_POINT('Ctrl Pts',(0.2148639642194,5.66733934524,-4.129850682383));
#29464=CARTESIAN_POINT('Ctrl Pts',(0.2159461215713,5.553757419004,-4.117045916765));
#29465=CARTESIAN_POINT('Ctrl Pts',(0.2121209376649,5.485326308278,-4.101312141519));
#29466=CARTESIAN_POINT('Ctrl Pts',(0.2115167758576,5.476087063052,-4.099045503577));
#29467=CARTESIAN_POINT('',(-0.0201793190613418,5.74664977779542,-3.67573539656421));
#29468=CARTESIAN_POINT('Ctrl Pts',(-8.5045295969094E-17,6.252471629776,
-3.532050807569));
#29469=CARTESIAN_POINT('Ctrl Pts',(-1.72754179486701E-9,6.22515092260001,
-3.542947549531));
#29470=CARTESIAN_POINT('Ctrl Pts',(-0.000132427690026248,6.19801380159061,
-3.55333740578014));
#29471=CARTESIAN_POINT('Ctrl Pts',(-0.000397224786372729,6.17126247112049,
-3.56316476120976));
#29472=CARTESIAN_POINT('Ctrl Pts',(-0.000637049866794604,6.14703395777986,
-3.57206533579596));
#29473=CARTESIAN_POINT('Ctrl Pts',(-0.000983692273868425,6.12312170573986,
-3.5805035516757));
#29474=CARTESIAN_POINT('Ctrl Pts',(-0.00145122229008661,6.09910625879538,
-3.58861822102923));
#29475=CARTESIAN_POINT('Ctrl Pts',(-0.00149990430028179,6.09660562740823,
-3.58946316873846));
#29476=CARTESIAN_POINT('Ctrl Pts',(-0.00154991211757044,6.09410386888282,
-3.5903045648392));
#29477=CARTESIAN_POINT('Ctrl Pts',(-0.00160127252760695,6.09160050491002,
-3.59114253456933));
#29478=CARTESIAN_POINT('Ctrl Pts',(-0.0021458856451855,6.06505545091433,
-3.60002815886317));
#29479=CARTESIAN_POINT('Ctrl Pts',(-0.00284151775027957,6.03833096917016,
-3.60853468104776));
#29480=CARTESIAN_POINT('Ctrl Pts',(-0.0037223342651763,6.01134660899402,
-3.61661970088636));
#29481=CARTESIAN_POINT('Ctrl Pts',(-0.00436205786534019,5.99174827977556,
-3.62249172747882));
#29482=CARTESIAN_POINT('Ctrl Pts',(-0.00509925812006014,5.9720138726226,
-3.62813767104629));
#29483=CARTESIAN_POINT('Ctrl Pts',(-0.00596753483628204,5.95189359828813,
-3.63358175376179));
#29484=CARTESIAN_POINT('Ctrl Pts',(-0.00629476266444873,5.94431086164487,
-3.63563346761069));
#29485=CARTESIAN_POINT('Ctrl Pts',(-0.00664075452653387,5.93667343669818,
-3.63765606058147));
#29486=CARTESIAN_POINT('Ctrl Pts',(-0.00700790819414537,5.92896854922353,
-3.63964899627758));
#29487=CARTESIAN_POINT('Ctrl Pts',(-0.00782485968872279,5.91182444882841,
-3.64408346592657));
#29488=CARTESIAN_POINT('Ctrl Pts',(-0.00874585896548231,5.89434844461603,
-3.6483701221662));
#29489=CARTESIAN_POINT('Ctrl Pts',(-0.00981144211653737,5.87644460480726,
-3.65245416715839));
#29490=CARTESIAN_POINT('Ctrl Pts',(-0.0104954637008456,5.86495173082641,
-3.65507580670212));
#29491=CARTESIAN_POINT('Ctrl Pts',(-0.011239294790122,5.85328292767612,
-3.65761330920383));
#29492=CARTESIAN_POINT('Ctrl Pts',(-0.0120569570969732,5.8414189888438,
-3.66004292839892));
#29493=CARTESIAN_POINT('Ctrl Pts',(-0.0120570279255355,5.84141796115092,
-3.66004313886041));
#29494=CARTESIAN_POINT('Ctrl Pts',(-0.01205709875466,5.84141693345665,-3.66004334932103));
#29495=CARTESIAN_POINT('Ctrl Pts',(-0.0120571695843467,5.84141590576098,
-3.66004355978076));
#29496=CARTESIAN_POINT('Ctrl Pts',(-0.0130092523383889,5.82760176412085,
-3.6628725300981));
#29497=CARTESIAN_POINT('Ctrl Pts',(-0.0140620820519736,5.81353299437985,
-3.66554488478095));
#29498=CARTESIAN_POINT('Ctrl Pts',(-0.015250518781809,5.79919911074599,
-3.66800316381262));
#29499=CARTESIAN_POINT('Ctrl Pts',(-0.0163231857994438,5.78626154005109,
-3.67022197342293));
#29500=CARTESIAN_POINT('Ctrl Pts',(-0.0175062495206092,5.77310770600626,
-3.6722665937512));
#29501=CARTESIAN_POINT('Ctrl Pts',(-0.0188341058644166,5.75975835931925,
-3.6740632774332));
#29502=CARTESIAN_POINT('Ctrl Pts',(-0.0192667280551368,5.75540907587805,
-3.67464864589882));
#29503=CARTESIAN_POINT('Ctrl Pts',(-0.0197147999565475,5.75103929996326,
-3.67520741276272));
#29504=CARTESIAN_POINT('Ctrl Pts',(-0.020179768057466,5.74665057746385,
-3.67573612888107));
#29505=CARTESIAN_POINT('',(0.0734352791607451,5.61504677957465,-3.92719395374012));
#29506=CARTESIAN_POINT('Ctrl Pts',(0.1339745962155,6.252471629345,-4.032050807569));
#29507=CARTESIAN_POINT('Ctrl Pts',(0.1339746659036,6.217593804566,-4.032050986724));
#29508=CARTESIAN_POINT('Ctrl Pts',(0.1331756273777,6.148571274798,-4.030666927977));
#29509=CARTESIAN_POINT('Ctrl Pts',(0.1296207577408,6.048706349432,-4.024509737841));
#29510=CARTESIAN_POINT('Ctrl Pts',(0.1233657849458,5.948101684635,-4.013675833537));
#29511=CARTESIAN_POINT('Ctrl Pts',(0.1137608443202,5.845755231197,-3.997039458174));
#29512=CARTESIAN_POINT('Ctrl Pts',(0.09929412924214,5.73725831333,-3.971982867046));
#29513=CARTESIAN_POINT('Ctrl Pts',(0.08367513844526,5.656233648091,-3.944928749805));
#29514=CARTESIAN_POINT('Ctrl Pts',(0.07343513682107,5.615047318658,-3.927194345532));
#29515=CARTESIAN_POINT('Origin',(0.9394606772721,5.615046199005,-3.42719362363));
#29516=CARTESIAN_POINT('Origin',(-0.5,3.8,0.));
#29517=CARTESIAN_POINT('',(-0.500000724156137,5.57843318952544,-3.35815048826204));
#29518=CARTESIAN_POINT('Origin',(-0.5,5.81246117975,-3.8));
#29519=CARTESIAN_POINT('',(-0.5000000000008,6.6267742539821,-2.53955651975393));
#29520=CARTESIAN_POINT('Origin',(-0.5,3.8,0.));
#29521=CARTESIAN_POINT('Origin',(-0.5,6.9987182356,-2.873708692481));
#29522=CARTESIAN_POINT('Ctrl Pts',(0.1027377857463,7.348398502532,-1.993772793209));
#29523=CARTESIAN_POINT('Ctrl Pts',(0.1018795142078,7.347090839248,-1.99856950602));
#29524=CARTESIAN_POINT('Ctrl Pts',(0.08748606425769,7.324973749974,-2.07931804569));
#29525=CARTESIAN_POINT('Ctrl Pts',(0.06218815931635,7.280065532666,-2.23117883235));
#29526=CARTESIAN_POINT('Ctrl Pts',(0.03182029544443,7.206284734385,-2.449036815777));
#29527=CARTESIAN_POINT('Ctrl Pts',(0.008692153136156,7.121345659417,-2.66975021154));
#29528=CARTESIAN_POINT('Ctrl Pts',(0.000309930076861,7.05450915858,-2.821709674269));
#29529=CARTESIAN_POINT('Ctrl Pts',(-0.001018477605139,7.016398931017,-2.902151700762));
#29530=CARTESIAN_POINT('Ctrl Pts',(-0.001081418569356,7.014306738012,-2.906550131397));
#29531=CARTESIAN_POINT('Ctrl Pts',(-0.0399338660445,7.115798705959,-1.82477577565));
#29532=CARTESIAN_POINT('Ctrl Pts',(-0.04008326187015,7.11417406958,-1.82941037646));
#29533=CARTESIAN_POINT('Ctrl Pts',(-0.04249896901661,7.086774456842,-1.907411774627));
#29534=CARTESIAN_POINT('Ctrl Pts',(-0.04384834652326,7.033658223989,-2.053551607733));
#29535=CARTESIAN_POINT('Ctrl Pts',(-0.03627411384628,6.953727053625,-2.261605825128));
#29536=CARTESIAN_POINT('Ctrl Pts',(-0.01768977584952,6.869675880613,-2.470533055801));
#29537=CARTESIAN_POINT('Ctrl Pts',(0.004566050698255,6.810275339171,-2.612726145468));
#29538=CARTESIAN_POINT('Ctrl Pts',(0.01963083731976,6.778767570989,-2.687391402537));
#29539=CARTESIAN_POINT('Ctrl Pts',(0.02046458526668,6.777044591192,-2.691471916486));
#29540=CARTESIAN_POINT('Ctrl Pts',(-0.3385562814282,7.087745121797,-1.710515139935));
#29541=CARTESIAN_POINT('Ctrl Pts',(-0.3385854937958,7.085344330529,-1.715026264093));
#29542=CARTESIAN_POINT('Ctrl Pts',(-0.3389179244204,7.044875153857,-1.790931560509));
#29543=CARTESIAN_POINT('Ctrl Pts',(-0.3344184843395,6.967075079031,-1.932588547285));
#29544=CARTESIAN_POINT('Ctrl Pts',(-0.3129178506928,6.851934620108,-2.132671483461));
#29545=CARTESIAN_POINT('Ctrl Pts',(-0.2740805475891,6.733152916448,-2.331716051354));
#29546=CARTESIAN_POINT('Ctrl Pts',(-0.2328066607505,6.65131313147,-2.465517500439));
#29547=CARTESIAN_POINT('Ctrl Pts',(-0.2060460780354,6.608722577737,-2.535169689394));
#29548=CARTESIAN_POINT('Ctrl Pts',(-0.2045679022214,6.606396058465,-2.538974208362));
#29549=CARTESIAN_POINT('Ctrl Pts',(-0.592664250327,7.283070119461,-1.727694044175));
#29550=CARTESIAN_POINT('Ctrl Pts',(-0.5932426506397,7.279955024242,-1.732203216897));
#29551=CARTESIAN_POINT('Ctrl Pts',(-0.6027847744321,7.227402840675,-1.808070564299));
#29552=CARTESIAN_POINT('Ctrl Pts',(-0.6144625375172,7.12501335913,-1.949492146448));
#29553=CARTESIAN_POINT('Ctrl Pts',(-0.6123999906409,6.969240688534,-2.148787406838));
#29554=CARTESIAN_POINT('Ctrl Pts',(-0.5883650519266,6.803424624825,-2.346487045211));
#29555=CARTESIAN_POINT('Ctrl Pts',(-0.5524599168805,6.684333856262,-2.478904894028));
#29556=CARTESIAN_POINT('Ctrl Pts',(-0.5265523235192,6.62041514534,-2.547672988512));
#29557=CARTESIAN_POINT('Ctrl Pts',(-0.5251145852718,6.616917489925,-2.551428709617));
#29558=CARTESIAN_POINT('',(0.0865773249525527,7.32353859101868,-1.99264087060027));
#29559=CARTESIAN_POINT('Ctrl Pts',(0.0865773249525527,7.32353859101868,
-1.99264087060027));
#29560=CARTESIAN_POINT('Ctrl Pts',(0.0865771947823673,7.32353836781842,
-1.99264166097111));
#29561=CARTESIAN_POINT('Ctrl Pts',(0.086577064612313,7.32353814461806,-1.99264245134174));
#29562=CARTESIAN_POINT('Ctrl Pts',(0.0865769344423899,7.32353792141759,
-1.99264324171215));
#29563=CARTESIAN_POINT('Ctrl Pts',(0.0784200001016045,7.3095513450823,-2.04217080846305));
#29564=CARTESIAN_POINT('Ctrl Pts',(0.0707810911838816,7.2951582449645,-2.09085455336554));
#29565=CARTESIAN_POINT('Ctrl Pts',(0.0637332814097185,7.28051481411837,
-2.13835021065206));
#29566=CARTESIAN_POINT('Ctrl Pts',(0.0597136280219686,7.27216306821502,
-2.16543892130584));
#29567=CARTESIAN_POINT('Ctrl Pts',(0.0558856017076574,7.26373046498478,
-2.19214149885421));
#29568=CARTESIAN_POINT('Ctrl Pts',(0.0522572081991286,7.25525026918575,
-2.21839710659367));
#29569=CARTESIAN_POINT('Ctrl Pts',(0.0471928269707495,7.24341391672931,
-2.2550437400591));
#29570=CARTESIAN_POINT('Ctrl Pts',(0.0425107423662426,7.23148153503544,
-2.29081396288452));
#29571=CARTESIAN_POINT('Ctrl Pts',(0.0381540197775249,7.21930644129638,
-2.32622193849712));
#29572=CARTESIAN_POINT('Ctrl Pts',(0.0339164169989268,7.20746423422267,
-2.36066180304784));
#29573=CARTESIAN_POINT('Ctrl Pts',(0.0299862609982032,7.19539220723823,
-2.39475922278885));
#29574=CARTESIAN_POINT('Ctrl Pts',(0.0263406370665062,7.18292131512308,
-2.42897308992333));
#29575=CARTESIAN_POINT('Ctrl Pts',(0.0228702839175758,7.17104998650207,
-2.46154205583199));
#29576=CARTESIAN_POINT('Ctrl Pts',(0.0196579772059949,7.15881950455865,
-2.49421313164689));
#29577=CARTESIAN_POINT('Ctrl Pts',(0.0167223210419962,7.14605148199297,
-2.5273562255484));
#29578=CARTESIAN_POINT('Ctrl Pts',(0.0139677607901511,7.13407109822549,
-2.55845477523683));
#29579=CARTESIAN_POINT('Ctrl Pts',(0.0114564603782286,7.12161730275651,
-2.58996911427475));
#29580=CARTESIAN_POINT('Ctrl Pts',(0.00923922793207137,7.10851913572161,
-2.62218604510167));
#29581=CARTESIAN_POINT('Ctrl Pts',(0.00878499123308488,7.10583575980087,
-2.62878621565919));
#29582=CARTESIAN_POINT('Ctrl Pts',(0.00834323197844714,7.10312525936709,
-2.63541580115636));
#29583=CARTESIAN_POINT('Ctrl Pts',(0.00791460756887311,7.10038603852835,
-2.6420771479805));
#29584=CARTESIAN_POINT('Ctrl Pts',(0.00537502089604281,7.08415623784361,
-2.6815454265942));
#29585=CARTESIAN_POINT('Ctrl Pts',(0.00329666450163376,7.06693306420007,
-2.72213393301624));
#29586=CARTESIAN_POINT('Ctrl Pts',(0.00190428975516473,7.04869070748955,
-2.76359889037046));
#29587=CARTESIAN_POINT('Ctrl Pts',(0.000692060774264857,7.03280855109417,
-2.79969910198664));
#29588=CARTESIAN_POINT('Ctrl Pts',(3.33158514292476E-7,7.01615400055903,
-2.8364631507495));
#29589=CARTESIAN_POINT('Ctrl Pts',(1.31917426878845E-14,6.998718237797,
-2.873708690212));
#29590=CARTESIAN_POINT('',(-0.326860549423355,7.16212374689392,-1.77090033128315));
#29591=CARTESIAN_POINT('Ctrl Pts',(-0.326860549423355,7.16212374689392,
-1.77090033128315));
#29592=CARTESIAN_POINT('Ctrl Pts',(-0.341476935580464,7.14155250819475,
-1.80995513075379));
#29593=CARTESIAN_POINT('Ctrl Pts',(-0.355243357180322,7.1204502792182,-1.84836296151781));
#29594=CARTESIAN_POINT('Ctrl Pts',(-0.36807890051019,7.09898686777342,-1.88591138220589));
#29595=CARTESIAN_POINT('Ctrl Pts',(-0.377748086069401,7.08281819437489,
-1.9141971070683));
#29596=CARTESIAN_POINT('Ctrl Pts',(-0.38688975485068,7.06644508030668,-1.94199540467259));
#29597=CARTESIAN_POINT('Ctrl Pts',(-0.395485916070083,7.04994875753415,
-1.96922143838673));
#29598=CARTESIAN_POINT('Ctrl Pts',(-0.404085211517348,7.03344642007283,
-1.9964573989265));
#29599=CARTESIAN_POINT('Ctrl Pts',(-0.412118118968983,7.01682138823379,
-2.02312644173482));
#29600=CARTESIAN_POINT('Ctrl Pts',(-0.419672264309048,6.99993273664901,
-2.04949488838498));
#29601=CARTESIAN_POINT('Ctrl Pts',(-0.426990524612547,6.98357144852062,
-2.07503995638378));
#29602=CARTESIAN_POINT('Ctrl Pts',(-0.433859736224371,6.966962542256,-2.10030304038216));
#29603=CARTESIAN_POINT('Ctrl Pts',(-0.440323069309193,6.94994622360776,
-2.12552084006602));
#29604=CARTESIAN_POINT('Ctrl Pts',(-0.442710521659904,6.94366066638457,
-2.1348358938231));
#29605=CARTESIAN_POINT('Ctrl Pts',(-0.445042205251157,6.93731921540242,
-2.14414470422125));
#29606=CARTESIAN_POINT('Ctrl Pts',(-0.447318840123917,6.93091273586232,
-2.15345894792871));
#29607=CARTESIAN_POINT('Ctrl Pts',(-0.453065560394441,6.91474139179818,
-2.1769701195086));
#29608=CARTESIAN_POINT('Ctrl Pts',(-0.458453707982576,6.89815868002326,
-2.20051479902279));
#29609=CARTESIAN_POINT('Ctrl Pts',(-0.463470320481012,6.88099827454854,
-2.22428451544489));
#29610=CARTESIAN_POINT('Ctrl Pts',(-0.468181060798269,6.86488417086694,
-2.24660494811022));
#29611=CARTESIAN_POINT('Ctrl Pts',(-0.472564400803481,6.84826055599381,
-2.26912390370278));
#29612=CARTESIAN_POINT('Ctrl Pts',(-0.476570826991915,6.83096858818743,
-2.29199185391141));
#29613=CARTESIAN_POINT('Ctrl Pts',(-0.479287319175806,6.81924405036223,
-2.30749709601038));
#29614=CARTESIAN_POINT('Ctrl Pts',(-0.481829773480396,6.80721183561284,
-2.32316262215034));
#29615=CARTESIAN_POINT('Ctrl Pts',(-0.484170543101125,6.79481658859908,
-2.33903262068985));
#29616=CARTESIAN_POINT('Ctrl Pts',(-0.488905298622254,6.76974429454912,
-2.37113341460814));
#29617=CARTESIAN_POINT('Ctrl Pts',(-0.492850085687612,6.74319348125157,
-2.40405829232308));
#29618=CARTESIAN_POINT('Ctrl Pts',(-0.495623538805572,6.71517798283673,
-2.4375635794965));
#29619=CARTESIAN_POINT('Ctrl Pts',(-0.498396991923532,6.6871624844219,-2.47106886666992));
#29620=CARTESIAN_POINT('Ctrl Pts',(-0.499999415858718,6.65768246277223,
-2.50515434966105));
#29621=CARTESIAN_POINT('Ctrl Pts',(-0.500000000001596,6.62677425398226,
-2.53955651975406));
#29622=CARTESIAN_POINT('Origin',(-0.3268607615544,7.60451284409,-2.00391666631));
#29623=CARTESIAN_POINT('Origin',(0.5,-42.4,0.));
#29624=CARTESIAN_POINT('',(0.517449748472425,7.45443543149202,-3.56771915706352));
#29625=CARTESIAN_POINT('Origin',(0.5,6.956014650303,-3.532050807563));
#29626=CARTESIAN_POINT('',(0.517453499954001,7.54185174628463,-2.0013495955528));
#29627=CARTESIAN_POINT('Origin',(0.5,7.0425494055,-1.981381677743));
#29628=CARTESIAN_POINT('Origin',(0.5174497483513,-42.4,0.));
#29629=CARTESIAN_POINT('Ctrl Pts',(0.001285129943234,6.928768667338,-3.501024341666));
#29630=CARTESIAN_POINT('Ctrl Pts',(0.001003718906394,6.928092877268,-3.51066527064));
#29631=CARTESIAN_POINT('Ctrl Pts',(0.0002283234512161,6.924321936393,-3.563904385738));
#29632=CARTESIAN_POINT('Ctrl Pts',(0.00658911429773,6.917089265922,-3.660499255977));
#29633=CARTESIAN_POINT('Ctrl Pts',(0.03208935343955,6.906663907416,-3.788338152623));
#29634=CARTESIAN_POINT('Ctrl Pts',(0.07394580619339,6.895769141277,-3.911589220024));
#29635=CARTESIAN_POINT('Ctrl Pts',(0.1166553948127,6.887488515458,-3.998174012346));
#29636=CARTESIAN_POINT('Ctrl Pts',(0.1438590730748,6.882919565931,-4.043718798227));
#29637=CARTESIAN_POINT('Ctrl Pts',(0.1489300235062,6.882088247686,-4.051932578979));
#29638=CARTESIAN_POINT('Ctrl Pts',(-0.01806327553642,7.257042281495,-3.523522559884));
#29639=CARTESIAN_POINT('Ctrl Pts',(-0.01835336820514,7.256343395302,-3.5334930686));
#29640=CARTESIAN_POINT('Ctrl Pts',(-0.01915268912732,7.252443569868,-3.588552069544));
#29641=CARTESIAN_POINT('Ctrl Pts',(-0.01259578433519,7.244963592271,-3.688447745911));
#29642=CARTESIAN_POINT('Ctrl Pts',(0.01369008223242,7.234181570178,-3.820653304321));
#29643=CARTESIAN_POINT('Ctrl Pts',(0.05683526715279,7.222914110192,-3.948112582044));
#29644=CARTESIAN_POINT('Ctrl Pts',(0.1008602464213,7.214350258091,-4.037654288618));
#29645=CARTESIAN_POINT('Ctrl Pts',(0.1289014667209,7.209625219336,-4.084753946765));
#29646=CARTESIAN_POINT('Ctrl Pts',(0.1341285295189,7.208765508589,-4.093248118291));
#29647=CARTESIAN_POINT('Ctrl Pts',(0.2189431301382,7.484961949496,-3.546425270851));
#29648=CARTESIAN_POINT('Ctrl Pts',(0.2187175076249,7.484415939128,-3.554209822187));
#29649=CARTESIAN_POINT('Ctrl Pts',(0.2180958581636,7.481370070208,-3.597198589814));
#29650=CARTESIAN_POINT('Ctrl Pts',(0.2231964118796,7.475537193372,-3.675204532862));
#29651=CARTESIAN_POINT('Ctrl Pts',(0.2436481704901,7.467148227663,-3.778456557303));
#29652=CARTESIAN_POINT('Ctrl Pts',(0.2772231730612,7.458397511567,-3.87801747527));
#29653=CARTESIAN_POINT('Ctrl Pts',(0.3114799869555,7.451757587929,-3.947956342863));
#29654=CARTESIAN_POINT('Ctrl Pts',(0.3333015807294,7.448096469322,-3.984749318309));
#29655=CARTESIAN_POINT('Ctrl Pts',(0.3373693460768,7.447430403692,-3.99138493732));
#29656=CARTESIAN_POINT('Ctrl Pts',(0.5469709874831,7.453533131528,-3.553755766535));
#29657=CARTESIAN_POINT('Ctrl Pts',(0.5468380131604,7.453209324245,-3.558363725938));
#29658=CARTESIAN_POINT('Ctrl Pts',(0.5464716902076,7.451404541169,-3.583812218248));
#29659=CARTESIAN_POINT('Ctrl Pts',(0.5494793641476,7.447964171537,-3.630007953227));
#29660=CARTESIAN_POINT('Ctrl Pts',(0.561547096288,7.443048609365,-3.691183951173));
#29661=CARTESIAN_POINT('Ctrl Pts',(0.5813690679602,7.437948418878,-3.750201563262));
#29662=CARTESIAN_POINT('Ctrl Pts',(0.6015883374525,7.434097464698,-3.791652588125));
#29663=CARTESIAN_POINT('Ctrl Pts',(0.6144718870048,7.431978095285,-3.813467167341));
#29664=CARTESIAN_POINT('Ctrl Pts',(0.6168736596913,7.431592627446,-3.817401798674));
#29665=CARTESIAN_POINT('',(0.584439518575878,7.43337435977711,-3.82024990776836));
#29666=CARTESIAN_POINT('Origin',(0.5669897707333,6.935140821459,-3.782055090282));
#29667=CARTESIAN_POINT('Origin',(1.02904178594563,7.43196848844121,-3.56616243168394));
#29668=CARTESIAN_POINT('Ctrl Pts',(0.1075899274291,6.910200321737,-3.984624534481));
#29669=CARTESIAN_POINT('Ctrl Pts',(0.2365969974133,6.888757665974,-4.208071334229));
#29670=CARTESIAN_POINT('Ctrl Pts',(0.5917961608702,6.825498881099,-4.823294332142));
#29671=CARTESIAN_POINT('Ctrl Pts',(1.187797482473,6.69978878732,-5.855598902537));
#29672=CARTESIAN_POINT('Ctrl Pts',(1.927362895286,6.511611808779,-7.13656377305));
#29673=CARTESIAN_POINT('Ctrl Pts',(2.448474526329,6.35378224873,-8.039155594431));
#29674=CARTESIAN_POINT('Ctrl Pts',(2.72900660943,6.261296816161,-8.525051415516));
#29675=CARTESIAN_POINT('Ctrl Pts',(2.737553413063,6.258472120031,-8.53985491365));
#29676=CARTESIAN_POINT('Ctrl Pts',(0.1045493633812,7.227561823644,-4.016835013129));
#29677=CARTESIAN_POINT('Ctrl Pts',(0.2341802329362,7.206015484363,-4.241362265427));
#29678=CARTESIAN_POINT('Ctrl Pts',(0.591097759154,7.142450678831,-4.859561554948));
#29679=CARTESIAN_POINT('Ctrl Pts',(1.189986798084,7.016131565785,-5.896867798471));
#29680=CARTESIAN_POINT('Ctrl Pts',(1.933144313516,6.827040714483,-7.184054373226));
#29681=CARTESIAN_POINT('Ctrl Pts',(2.456795161336,6.668442221886,-8.091044247077));
#29682=CARTESIAN_POINT('Ctrl Pts',(2.738697034763,6.575505198669,-8.579312614601));
#29683=CARTESIAN_POINT('Ctrl Pts',(2.747285573639,6.572666709152,-8.594188400297));
#29684=CARTESIAN_POINT('Ctrl Pts',(0.3084981556159,7.45325258704,-3.920743118734));
#29685=CARTESIAN_POINT('Ctrl Pts',(0.4385726385281,7.431632513509,-4.146038731906));
#29686=CARTESIAN_POINT('Ctrl Pts',(0.7967121737199,7.367850082224,-4.766354603057));
#29687=CARTESIAN_POINT('Ctrl Pts',(1.397654804922,7.241097866794,-5.807217772734));
#29688=CARTESIAN_POINT('Ctrl Pts',(2.1433668343,7.051357117379,-7.098828895431));
#29689=CARTESIAN_POINT('Ctrl Pts',(2.668823439181,6.892211800505,-8.008946432258));
#29690=CARTESIAN_POINT('Ctrl Pts',(2.951699435248,6.798953629834,-8.498902029688));
#29691=CARTESIAN_POINT('Ctrl Pts',(2.960317654028,6.79610533119,-8.513829222485));
#29692=CARTESIAN_POINT('Ctrl Pts',(0.5837385360342,7.437108776495,-3.760283800157));
#29693=CARTESIAN_POINT('Ctrl Pts',(0.7137812869877,7.415493977224,-3.985524451965));
#29694=CARTESIAN_POINT('Ctrl Pts',(1.071833411064,7.351727112854,-4.605688922623));
#29695=CARTESIAN_POINT('Ctrl Pts',(1.672629147444,7.225005877526,-5.646297663004));
#29696=CARTESIAN_POINT('Ctrl Pts',(2.418158450738,7.035311615755,-6.937592294841));
#29697=CARTESIAN_POINT('Ctrl Pts',(2.943485888615,6.876205413586,-7.847486107853));
#29698=CARTESIAN_POINT('Ctrl Pts',(3.226292205042,6.782970214806,-8.337321016606));
#29699=CARTESIAN_POINT('Ctrl Pts',(3.234908300798,6.780122617815,-8.352244532218));
#29700=CARTESIAN_POINT('',(3.16400873498434,6.78858150430351,-8.33346840037192));
#29701=CARTESIAN_POINT('Origin',(-2.22649218408928,-42.9537256923742,1.07765501392591));
#29702=CARTESIAN_POINT('',(2.71354627844193,6.29590662476739,-8.50000002294956));
#29703=CARTESIAN_POINT('Origin',(3.146558987422,6.295906623345,-8.250000035222));
#29704=CARTESIAN_POINT('Ctrl Pts',(0.133975835628604,6.93514102322294,-4.03205295429546));
#29705=CARTESIAN_POINT('Ctrl Pts',(0.248035870487217,6.91600141019252,-4.22961072978345));
#29706=CARTESIAN_POINT('Ctrl Pts',(0.362516631904128,6.89557480007011,-4.42789722465242));
#29707=CARTESIAN_POINT('Ctrl Pts',(0.476791103889355,6.87398689887345,-4.62582641581095));
#29708=CARTESIAN_POINT('Ctrl Pts',(0.482878673537709,6.87283687954006,-4.63637039571904));
#29709=CARTESIAN_POINT('Ctrl Pts',(0.488965658428778,6.87168357686734,-4.64691336279973));
#29710=CARTESIAN_POINT('Ctrl Pts',(0.495051964002143,6.87052701398906,-4.65745515327007));
#29711=CARTESIAN_POINT('Ctrl Pts',(0.575619875510765,6.85521692899437,-4.79700286928915));
#29712=CARTESIAN_POINT('Ctrl Pts',(0.656068680033741,6.83933448907174,-4.93634428707301));
#29713=CARTESIAN_POINT('Ctrl Pts',(0.736179400348117,6.82294025017375,-5.07510012488849));
#29714=CARTESIAN_POINT('Ctrl Pts',(0.8221140916706,6.80535416614358,-5.22394337639183));
#29715=CARTESIAN_POINT('Ctrl Pts',(0.907658335949794,6.78715361300796,-5.37211035257136));
#29716=CARTESIAN_POINT('Ctrl Pts',(0.993626289906327,6.76817004995011,-5.52101121679085));
#29717=CARTESIAN_POINT('Ctrl Pts',(1.05313261411875,6.7550297807447,-5.62407919379812));
#29718=CARTESIAN_POINT('Ctrl Pts',(1.11284190195264,6.74151329238067,-5.7274987143937));
#29719=CARTESIAN_POINT('Ctrl Pts',(1.17302336159817,6.7275501453763,-5.83173606042337));
#29720=CARTESIAN_POINT('Ctrl Pts',(1.22800856343403,6.71479262070306,-5.92697322389587));
#29721=CARTESIAN_POINT('Ctrl Pts',(1.28338791583026,6.70166212210795,-6.02289307603832));
#29722=CARTESIAN_POINT('Ctrl Pts',(1.33936622442084,6.688095964508,-6.11985035063901));
#29723=CARTESIAN_POINT('Ctrl Pts',(1.43348966283431,6.66528546109131,-6.28287692815426));
#29724=CARTESIAN_POINT('Ctrl Pts',(1.52930637368736,6.64125189706976,-6.44883633960552));
#29725=CARTESIAN_POINT('Ctrl Pts',(1.62743110009301,6.6157179419123,-6.61879335115343));
#29726=CARTESIAN_POINT('Ctrl Pts',(1.71482541704086,6.59297624721713,-6.77016474834157));
#29727=CARTESIAN_POINT('Ctrl Pts',(1.80405054587966,6.56904390809249,-6.92470720466088));
#29728=CARTESIAN_POINT('Ctrl Pts',(1.89553771225012,6.54369067439583,-7.08316762517741));
#29729=CARTESIAN_POINT('Ctrl Pts',(1.92588369818274,6.53528109189779,-7.13572841465908));
#29730=CARTESIAN_POINT('Ctrl Pts',(1.95647853330762,6.52671490024969,-7.18872022360712));
#29731=CARTESIAN_POINT('Ctrl Pts',(1.98733784099078,6.51798285441075,-7.24217011240074));
#29732=CARTESIAN_POINT('Ctrl Pts',(2.15286381690566,6.47114510859792,-7.52886951265766));
#29733=CARTESIAN_POINT('Ctrl Pts',(2.32600373553534,6.41959121679276,-7.82875664840512));
#29734=CARTESIAN_POINT('Ctrl Pts',(2.50587483237852,6.36282325692957,-8.14030252705253));
#29735=CARTESIAN_POINT('Ctrl Pts',(2.57414529434987,6.34127685557299,-8.25855043588178));
#29736=CARTESIAN_POINT('Ctrl Pts',(2.64338533227658,6.31897976149477,-8.3784776994861));
#29737=CARTESIAN_POINT('Ctrl Pts',(2.71354626504585,6.295906630069,-8.49999999974909));
#29738=CARTESIAN_POINT('Origin',(3.002221399786,0.,-9.));
#29739=CARTESIAN_POINT('',(3.386180225107E-13,5.244818327676,-3.800000000001));
#29740=CARTESIAN_POINT('Ctrl Pts',(0.0734354173720697,5.61504677956584,
-3.92719387396377));
#29741=CARTESIAN_POINT('Ctrl Pts',(0.0689743793199208,5.59710734302576,
-3.91946712940295));
#29742=CARTESIAN_POINT('Ctrl Pts',(0.0646056578481124,5.5784360241764,-3.91190028184966));
#29743=CARTESIAN_POINT('Ctrl Pts',(0.0602886395540653,5.55918434054357,
-3.90442298682717));
#29744=CARTESIAN_POINT('Ctrl Pts',(0.0559715780169001,5.53993246406866,
-3.8969456169054));
#29745=CARTESIAN_POINT('Ctrl Pts',(0.0517062206933113,5.52010021118334,
-3.88955780130851));
#29746=CARTESIAN_POINT('Ctrl Pts',(0.0474222609735764,5.49942329140985,
-3.88213776541635));
#29747=CARTESIAN_POINT('Ctrl Pts',(0.0431383012538383,5.47874637163634,
-3.87471772952418));
#29748=CARTESIAN_POINT('Ctrl Pts',(0.0388357391379535,5.45722478497467,
-3.86726547333675));
#29749=CARTESIAN_POINT('Ctrl Pts',(0.034760148805027,5.4362886991235,-3.86020634380928));
#29750=CARTESIAN_POINT('Ctrl Pts',(0.0306845584721015,5.41535261327233,
-3.85314721428182));
#29751=CARTESIAN_POINT('Ctrl Pts',(0.0268359399221341,5.39500202823166,
-3.84648121141432));
#29752=CARTESIAN_POINT('Ctrl Pts',(0.0230645959593961,5.37465460666466,
-3.83994905205804));
#29753=CARTESIAN_POINT('Ctrl Pts',(0.0192932519966604,5.35430718509767,
-3.83341689270177));
#29754=CARTESIAN_POINT('Ctrl Pts',(0.0155991826211542,5.33396292700434,
-3.82701857685671));
#29755=CARTESIAN_POINT('Ctrl Pts',(0.011776540402697,5.31245424544518,-3.82039756631518));
#29756=CARTESIAN_POINT('Ctrl Pts',(0.00795389818423762,5.29094556388601,
-3.81377655577365));
#29757=CARTESIAN_POINT('Ctrl Pts',(0.0040026831228265,5.268272458861,-3.80693285053566));
#29758=CARTESIAN_POINT('Ctrl Pts',(3.76143560743003E-13,5.244818327676,
-3.80000000000098));
#29759=CARTESIAN_POINT('',(2.713546265044,1.304093369931,-8.499999999745));
#29760=CARTESIAN_POINT('',(2.713546265046,6.295906630069,-8.499999999749));
#29761=CARTESIAN_POINT('',(0.133974522815126,0.66485875628202,-4.03205067311006));
#29762=CARTESIAN_POINT('Ctrl Pts',(2.71354626504418,1.304093369931,-8.4999999997449));
#29763=CARTESIAN_POINT('Ctrl Pts',(2.61159997231137,1.27056729429867,-8.3234238410882));
#29764=CARTESIAN_POINT('Ctrl Pts',(2.50910501193143,1.2378821522437,-8.14589736143207));
#29765=CARTESIAN_POINT('Ctrl Pts',(2.40674837211237,1.20622891171289,-7.96861045946304));
#29766=CARTESIAN_POINT('Ctrl Pts',(2.30924947494878,1.17607790198004,-7.79973741464557));
#29767=CARTESIAN_POINT('Ctrl Pts',(2.21187614287338,1.14686278150517,-7.63108185950621));
#29768=CARTESIAN_POINT('Ctrl Pts',(2.11522487961953,1.11870492115182,-7.46367696093502));
#29769=CARTESIAN_POINT('Ctrl Pts',(2.09351075323304,1.11237884410014,-7.42606699079168));
#29770=CARTESIAN_POINT('Ctrl Pts',(2.07183288047179,1.10610895833824,-7.38851981327021));
#29771=CARTESIAN_POINT('Ctrl Pts',(2.05017111365136,1.09988905714736,-7.3510005318615));
#29772=CARTESIAN_POINT('Ctrl Pts',(1.97331024742889,1.07781943571198,-7.21787360398792));
#29773=CARTESIAN_POINT('Ctrl Pts',(1.89665242668735,1.05637516593552,-7.08509835967507));
#29774=CARTESIAN_POINT('Ctrl Pts',(1.81929488308289,1.0353118673009,-6.95111116385844));
#29775=CARTESIAN_POINT('Ctrl Pts',(1.74288942113456,1.01450780621848,-6.81877302184251));
#29776=CARTESIAN_POINT('Ctrl Pts',(1.665801326986,0.994075360144622,-6.68525252998749));
#29777=CARTESIAN_POINT('Ctrl Pts',(1.58715752976534,0.973829251194698,-6.54903747990535));
#29778=CARTESIAN_POINT('Ctrl Pts',(1.5631206815207,0.967641189763631,-6.50740443822663));
#29779=CARTESIAN_POINT('Ctrl Pts',(1.53893848254314,0.96147089723312,-6.46551964148831));
#29780=CARTESIAN_POINT('Ctrl Pts',(1.51458594875602,0.95531405854845,-6.42333981567596));
#29781=CARTESIAN_POINT('Ctrl Pts',(1.46961768989598,0.943945125929286,-6.34545250660246));
#29782=CARTESIAN_POINT('Ctrl Pts',(1.42406936453429,0.932612495198426,-6.26656049131749));
#29783=CARTESIAN_POINT('Ctrl Pts',(1.37795947539797,0.921336565457625,-6.18669581966957));
#29784=CARTESIAN_POINT('Ctrl Pts',(1.22462045111637,0.883838317322376,-5.9211048357299));
#29785=CARTESIAN_POINT('Ctrl Pts',(1.06507017471814,0.846970542877258,-5.64475565567324));
#29786=CARTESIAN_POINT('Ctrl Pts',(0.899997396731987,0.811456784908397,
-5.35884121775675));
#29787=CARTESIAN_POINT('Ctrl Pts',(0.885732238628493,0.808387778749686,
-5.33413323918689));
#29788=CARTESIAN_POINT('Ctrl Pts',(0.871425846050205,0.805328855185408,
-5.3093538403878));
#29789=CARTESIAN_POINT('Ctrl Pts',(0.857078667709878,0.802280463959259,
-5.28450379855709));
#29790=CARTESIAN_POINT('Ctrl Pts',(0.782414631538548,0.786416355534968,
-5.15518189441013));
#29791=CARTESIAN_POINT('Ctrl Pts',(0.706645722013296,0.77084087237109,-5.02394629316002));
#29792=CARTESIAN_POINT('Ctrl Pts',(0.629748301253577,0.755591732168624,
-4.89075605342435));
#29793=CARTESIAN_POINT('Ctrl Pts',(0.469464328013554,0.723806624735922,
-4.61313606811522));
#29794=CARTESIAN_POINT('Ctrl Pts',(0.304277117249445,0.693436027781902,
-4.32702342665655));
#29795=CARTESIAN_POINT('Ctrl Pts',(0.133974596315389,0.6648587720723,-4.03205080774139));
#29796=CARTESIAN_POINT('',(0.1339745962156,1.347528370654,-4.032050807569));
#29797=CARTESIAN_POINT('',(0.1339745962156,1.347528370654,-4.032050807569));
#29798=CARTESIAN_POINT('',(0.073424843718969,1.98498956165576,-3.92717625701886));
#29799=CARTESIAN_POINT('Origin',(-0.147569422083157,1.04172484501738,-3.54440667724998));
#29800=CARTESIAN_POINT('',(-1.29347819189345E-8,2.3551814754037,-3.79999997759638));
#29801=CARTESIAN_POINT('Origin',(-0.118328490245077,4.15913738516639,-3.59504904291298));
#29802=CARTESIAN_POINT('',(0.144337567297357,3.80000000094331,-4.05000000000003));
#29803=CARTESIAN_POINT('Ctrl Pts',(0.1443375672974,3.799999999999,-4.05));
#29804=CARTESIAN_POINT('Ctrl Pts',(0.1443378988472,3.641734883366,-4.050000360009));
#29805=CARTESIAN_POINT('Ctrl Pts',(0.1338002849907,3.32390084097,-4.031748979448));
#29806=CARTESIAN_POINT('Ctrl Pts',(0.09119286281607,2.871512797023,-3.957950685846));
#29807=CARTESIAN_POINT('Ctrl Pts',(0.03592693705457,2.529613680379,-3.86222718878));
#29808=CARTESIAN_POINT('Ctrl Pts',(1.940475558015E-12,2.35518167234,-3.800000000003));
#29809=CARTESIAN_POINT('Ctrl Pts',(3.386180225107E-13,5.244818327676,-3.800000000001));
#29810=CARTESIAN_POINT('Ctrl Pts',(0.03068642401925,5.095833738666,-3.85315021964));
#29811=CARTESIAN_POINT('Ctrl Pts',(0.08230825724947,4.790451591005,-3.942562156105));
#29812=CARTESIAN_POINT('Ctrl Pts',(0.1295377956624,4.345878065346,-4.024366128052));
#29813=CARTESIAN_POINT('Ctrl Pts',(0.1443374902468,3.988290562368,-4.049999621017));
#29814=CARTESIAN_POINT('Ctrl Pts',(0.1443375672974,3.799999999999,-4.05));
#29815=CARTESIAN_POINT('Ctrl Pts',(-0.01984074734411,5.778719106975,-3.658132002503));
#29816=CARTESIAN_POINT('Ctrl Pts',(-0.02151789291509,5.772219745287,-3.655227101155));
#29817=CARTESIAN_POINT('Ctrl Pts',(-0.02874571800289,5.743664386755,-3.642708140867));
#29818=CARTESIAN_POINT('Ctrl Pts',(-0.04083585898923,5.692008838292,-3.621767402488));
#29819=CARTESIAN_POINT('Ctrl Pts',(-0.05561412281504,5.623164700404,-3.596170698722));
#29820=CARTESIAN_POINT('Ctrl Pts',(-0.06929848073128,5.554723990994,-3.572468695329));
#29821=CARTESIAN_POINT('Ctrl Pts',(-0.08205687983033,5.487371187967,-3.55037050065));
#29822=CARTESIAN_POINT('Ctrl Pts',(-0.0944087317008,5.419259193829,-3.528976462696));
#29823=CARTESIAN_POINT('Ctrl Pts',(-0.1033895478633,5.367635088747,-3.513421241507));
#29824=CARTESIAN_POINT('Ctrl Pts',(-0.1084344694084,5.33794230972,-3.504684713301));
#29825=CARTESIAN_POINT('Ctrl Pts',(-0.1093975902414,5.332248875779,-3.503016900451));
#29826=CARTESIAN_POINT('Ctrl Pts',(-0.002985157552623,5.726476579393,-3.765100576803));
#29827=CARTESIAN_POINT('Ctrl Pts',(-0.004518714363548,5.720537561251,-3.762444378488));
#29828=CARTESIAN_POINT('Ctrl Pts',(-0.01117002684806,5.694267120759,-3.750923967326));
#29829=CARTESIAN_POINT('Ctrl Pts',(-0.02257083122652,5.645585694094,-3.731177194912));
#29830=CARTESIAN_POINT('Ctrl Pts',(-0.03671407770094,5.579712000861,-3.706680373465));
#29831=CARTESIAN_POINT('Ctrl Pts',(-0.04994669756034,5.513541725306,-3.68376080341));
#29832=CARTESIAN_POINT('Ctrl Pts',(-0.06239188724486,5.447846771628,-3.662205103075));
#29833=CARTESIAN_POINT('Ctrl Pts',(-0.0744755782777,5.381214825156,-3.641275534353));
#29834=CARTESIAN_POINT('Ctrl Pts',(-0.08329239205763,5.330536275783,-3.626004370564));
#29835=CARTESIAN_POINT('Ctrl Pts',(-0.08824062183765,5.301408245067,-3.617434778462));
#29836=CARTESIAN_POINT('Ctrl Pts',(-0.0891849730255,5.295824591682,-3.615799348484));
#29837=CARTESIAN_POINT('Ctrl Pts',(0.03425994679476,5.671886279934,-3.865541747954));
#29838=CARTESIAN_POINT('Ctrl Pts',(0.03287643160393,5.666532787098,-3.863145429351));
#29839=CARTESIAN_POINT('Ctrl Pts',(0.02682754011999,5.642649948543,-3.852668441972));
#29840=CARTESIAN_POINT('Ctrl Pts',(0.01614705102297,5.597076300293,-3.834169292197));
#29841=CARTESIAN_POINT('Ctrl Pts',(0.002667359496765,5.534306543082,-3.810821781622));
#29842=CARTESIAN_POINT('Ctrl Pts',(-0.01009322126234,5.470508734362,-3.78871980735));
#29843=CARTESIAN_POINT('Ctrl Pts',(-0.02221112594464,5.406546133551,-3.76773098098));
#29844=CARTESIAN_POINT('Ctrl Pts',(-0.03401460502959,5.34146074788,-3.747286754671));
#29845=CARTESIAN_POINT('Ctrl Pts',(-0.04266004618244,5.291770247358,-3.732312413783));
#29846=CARTESIAN_POINT('Ctrl Pts',(-0.04750725449303,5.263232420449,-3.723917232833));
#29847=CARTESIAN_POINT('Ctrl Pts',(-0.04843199622471,5.257763499078,-3.72231563461));
#29848=CARTESIAN_POINT('Ctrl Pts',(0.09069940064414,5.616699966831,-3.956232440606));
#29849=CARTESIAN_POINT('Ctrl Pts',(0.08946756522009,5.611938392032,-3.954098839065));
#29850=CARTESIAN_POINT('Ctrl Pts',(0.08402767193487,5.590469223109,-3.944676667507));
#29851=CARTESIAN_POINT('Ctrl Pts',(0.07407536246235,5.548037283815,-3.92743876185));
#29852=CARTESIAN_POINT('Ctrl Pts',(0.06126647054354,5.488405351215,-3.905253110252));
#29853=CARTESIAN_POINT('Ctrl Pts',(0.04898308257803,5.427005911782,-3.883977658227));
#29854=CARTESIAN_POINT('Ctrl Pts',(0.03719603617657,5.364794577562,-3.863561894917));
#29855=CARTESIAN_POINT('Ctrl Pts',(0.02567582837665,5.301272637951,-3.843608309962));
#29856=CARTESIAN_POINT('Ctrl Pts',(0.01720363088747,5.252580973739,-3.828934032668));
#29857=CARTESIAN_POINT('Ctrl Pts',(0.01245853205391,5.224639866974,-3.820715141208));
#29858=CARTESIAN_POINT('Ctrl Pts',(0.01155361033798,5.219286947419,-3.819147737991));
#29859=CARTESIAN_POINT('Ctrl Pts',(-0.0201784110928209,5.74664992548515,
-3.67573593484731));
#29860=CARTESIAN_POINT('Ctrl Pts',(-0.0201784354696587,5.74664939526823,
-3.67573612144244));
#29861=CARTESIAN_POINT('Ctrl Pts',(-0.0201784598462801,5.74664886505137,
-3.67573630803726));
#29862=CARTESIAN_POINT('Ctrl Pts',(-0.020178484222685,5.7466483348346,-3.67573649463177));
#29863=CARTESIAN_POINT('Ctrl Pts',(-0.0209814232443088,5.72918342386011,
-3.68188276676627));
#29864=CARTESIAN_POINT('Ctrl Pts',(-0.0215496981580626,5.71179450558293,
-3.68769910806057));
#29865=CARTESIAN_POINT('Ctrl Pts',(-0.0219239143907458,5.69464667663326,
-3.69319344038992));
#29866=CARTESIAN_POINT('Ctrl Pts',(-0.0222159929576374,5.68126266795729,
-3.69748180784334));
#29867=CARTESIAN_POINT('Ctrl Pts',(-0.0223899043208644,5.66802664780854,
-3.70157408075059));
#29868=CARTESIAN_POINT('Ctrl Pts',(-0.0224622993826163,5.65503849956244,
-3.70548017730559));
#29869=CARTESIAN_POINT('Ctrl Pts',(-0.0224623092421808,5.655036730692,-3.70548070928125));
#29870=CARTESIAN_POINT('Ctrl Pts',(-0.0224623190998546,5.65503496182611,
-3.7054812412535));
#29871=CARTESIAN_POINT('Ctrl Pts',(-0.0224623289556378,5.65503319296475,
-3.70548177322234));
#29872=CARTESIAN_POINT('Ctrl Pts',(-0.0225576168824433,5.63793144391809,
-3.7106249675194));
#29873=CARTESIAN_POINT('Ctrl Pts',(-0.0224803444260501,5.6212524460535,
-3.7154476654276));
#29874=CARTESIAN_POINT('Ctrl Pts',(-0.0222698926513762,5.60469313910181,
-3.72006135912167));
#29875=CARTESIAN_POINT('Ctrl Pts',(-0.0221157521730552,5.59256466217092,
-3.72344055111915));
#29876=CARTESIAN_POINT('Ctrl Pts',(-0.0218890281308965,5.58050088128577,
-3.72670819678444));
#29877=CARTESIAN_POINT('Ctrl Pts',(-0.021590073938272,5.56838931652737,
-3.72991372001025));
#29878=CARTESIAN_POINT('Ctrl Pts',(-0.0210930236774006,5.54825226352312,
-3.73524331964433));
#29879=CARTESIAN_POINT('Ctrl Pts',(-0.0203949237649873,5.52797573110029,
-3.74038852222518));
#29880=CARTESIAN_POINT('Ctrl Pts',(-0.019546685278498,5.50816848599496,
-3.74523501469395));
#29881=CARTESIAN_POINT('Ctrl Pts',(-0.0191881341317336,5.49979594624361,
-3.74728363128013));
#29882=CARTESIAN_POINT('Ctrl Pts',(-0.0188034447277056,5.49150724371414,
-3.7492787304572));
#29883=CARTESIAN_POINT('Ctrl Pts',(-0.0183991125698059,5.48334826563006,
-3.75121139305542));
#29884=CARTESIAN_POINT('Ctrl Pts',(-0.0183990893589477,5.48334779726048,
-3.75121150400073));
#29885=CARTESIAN_POINT('Ctrl Pts',(-0.0183990661480251,5.48334732889133,
-3.75121161494584));
#29886=CARTESIAN_POINT('Ctrl Pts',(-0.0183990429370381,5.4833468605226,
-3.75121172589074));
#29887=CARTESIAN_POINT('Ctrl Pts',(-0.0174959282178277,5.46512313347947,
-3.75552847352253));
#29888=CARTESIAN_POINT('Ctrl Pts',(-0.0164952009111264,5.44755019954919,
-3.75954106424298));
#29889=CARTESIAN_POINT('Ctrl Pts',(-0.0154116253866607,5.43029031610371,
-3.7633559520826));
#29890=CARTESIAN_POINT('Ctrl Pts',(-0.0148623564371937,5.42154120924962,
-3.76528973462815));
#29891=CARTESIAN_POINT('Ctrl Pts',(-0.0142910671327694,5.41287304683532,
-3.7671729788354));
#29892=CARTESIAN_POINT('Ctrl Pts',(-0.0136956716655769,5.40424442836318,
-3.76902069403971));
#29893=CARTESIAN_POINT('Ctrl Pts',(-0.0123428919870068,5.38463961044561,
-3.77321883077051));
#29894=CARTESIAN_POINT('Ctrl Pts',(-0.0108709353686572,5.36523333453026,
-3.77723016957813));
#29895=CARTESIAN_POINT('Ctrl Pts',(-0.00924390264763095,5.34538151671619,
-3.78118265844034));
#29896=CARTESIAN_POINT('Ctrl Pts',(-0.00874213708005937,5.33925935426422,
-3.78240157849747));
#29897=CARTESIAN_POINT('Ctrl Pts',(-0.00822524663056512,5.33309483828452,
-3.78361490643188));
#29898=CARTESIAN_POINT('Ctrl Pts',(-0.00769119476733997,5.32686912636376,
-3.78482636825632));
#29899=CARTESIAN_POINT('Ctrl Pts',(-0.00576649863884664,5.30443197286591,
-3.78919241590802));
#29900=CARTESIAN_POINT('Ctrl Pts',(-0.00361826650166239,5.28120087535866,
-3.79352982465151));
#29901=CARTESIAN_POINT('Ctrl Pts',(-0.00126811120227719,5.25747582420667,
-3.79776089073069));
#29902=CARTESIAN_POINT('Ctrl Pts',(-0.000851633964029754,5.2532714451243,
-3.79851068914442));
#29903=CARTESIAN_POINT('Ctrl Pts',(-0.00042886831096522,5.24905166975247,
-3.79925718508722));
#29904=CARTESIAN_POINT('Ctrl Pts',(4.14410515212417E-13,5.244818327676,
-3.80000000000096));
#29905=CARTESIAN_POINT('Ctrl Pts',(-0.01268225407336,5.772800830803,-3.694029050448));
#29906=CARTESIAN_POINT('Ctrl Pts',(-0.01301759475994,5.739068753102,-3.712030303038));
#29907=CARTESIAN_POINT('Ctrl Pts',(-0.01039416813831,5.648078305665,-3.759169807315));
#29908=CARTESIAN_POINT('Ctrl Pts',(0.007243773431018,5.489308134892,-3.83432961623));
#29909=CARTESIAN_POINT('Ctrl Pts',(0.03200461319616,5.356083219744,-3.889613921073));
#29910=CARTESIAN_POINT('Ctrl Pts',(0.04752295287887,5.284287176484,-3.917085317952));
#29911=CARTESIAN_POINT('Ctrl Pts',(0.04864194797635,5.279159326484,-3.919035833836));
#29912=CARTESIAN_POINT('Ctrl Pts',(-0.06997922621458,5.655780000582,-3.474398901289));
#29913=CARTESIAN_POINT('Ctrl Pts',(-0.07032635079946,5.623484779779,-3.49163753327));
#29914=CARTESIAN_POINT('Ctrl Pts',(-0.06761185683549,5.536547101997,-3.536642069158));
#29915=CARTESIAN_POINT('Ctrl Pts',(-0.04957369418306,5.385410837322,-3.607995938579));
#29916=CARTESIAN_POINT('Ctrl Pts',(-0.02442010904563,5.258978615888,-3.660231095361));
#29917=CARTESIAN_POINT('Ctrl Pts',(-0.008697108721838,5.190924849655,-3.686137282999));
#29918=CARTESIAN_POINT('Ctrl Pts',(-0.007563539672665,5.186064676355,-3.687976401988));
#29919=CARTESIAN_POINT('Ctrl Pts',(-0.2743702068952,5.585058547127,-3.338610219652));
#29920=CARTESIAN_POINT('Ctrl Pts',(-0.2747593672533,5.550259551039,-3.357212409689));
#29921=CARTESIAN_POINT('Ctrl Pts',(-0.2717200159241,5.457732776618,-3.404879810051));
#29922=CARTESIAN_POINT('Ctrl Pts',(-0.2522541760907,5.300544900304,-3.477833556881));
#29923=CARTESIAN_POINT('Ctrl Pts',(-0.2256995812873,5.171582624003,-3.529601984754));
#29924=CARTESIAN_POINT('Ctrl Pts',(-0.209246511161,5.102702800412,-3.554946751412));
#29925=CARTESIAN_POINT('Ctrl Pts',(-0.2080609536006,5.097786222214,-3.556744268162));
#29926=CARTESIAN_POINT('Ctrl Pts',(-0.5292956670922,5.5940470946,-3.350813053167));
#29927=CARTESIAN_POINT('Ctrl Pts',(-0.5297372563238,5.553986538552,-3.372260800208));
#29928=CARTESIAN_POINT('Ctrl Pts',(-0.5262927285377,5.448869233457,-3.426130892594));
#29929=CARTESIAN_POINT('Ctrl Pts',(-0.5050462266558,5.274803163949,-3.505334510713));
#29930=CARTESIAN_POINT('Ctrl Pts',(-0.4767442307066,5.135183346856,-3.559439123509));
#29931=CARTESIAN_POINT('Ctrl Pts',(-0.4593805852712,5.061299382153,-3.585491487082));
#29932=CARTESIAN_POINT('Ctrl Pts',(-0.458130185343,5.056028964579,-3.587336850212));
#29933=CARTESIAN_POINT('',(-0.4330127018922,5.076816196554,-3.579069767442));
#29934=CARTESIAN_POINT('Origin',(-0.4330127019006,5.244818327721,-4.049999999986));
#29935=CARTESIAN_POINT('Ctrl Pts',(-0.5000021724644,5.578412269071,-3.358161259976));
#29936=CARTESIAN_POINT('Ctrl Pts',(-0.5000045975026,5.526517536485,-3.385642436917));
#29937=CARTESIAN_POINT('Ctrl Pts',(-0.4942244627249,5.419967689217,-3.438990063122));
#29938=CARTESIAN_POINT('Ctrl Pts',(-0.4708077496976,5.252312611015,-3.513147270451));
#29939=CARTESIAN_POINT('Ctrl Pts',(-0.4468343747841,5.13611833078,-3.557914058777));
#29940=CARTESIAN_POINT('Ctrl Pts',(-0.4330127018922,5.076816196554,-3.579069767442));
#29941=CARTESIAN_POINT('Origin',(0.,3.8,0.));
#29942=CARTESIAN_POINT('',(-0.3268619336444,0.437875148065591,-1.77090837708039));
#29943=CARTESIAN_POINT('',(-4.03990376683404E-8,0.000376013360896276,-0.053456151853531));
#29944=CARTESIAN_POINT('Ctrl Pts',(-0.326861921820454,0.437875149890247,
-1.77090838054216));
#29945=CARTESIAN_POINT('Ctrl Pts',(-0.319542282990462,0.427568175634498,
-1.75134026812288));
#29946=CARTESIAN_POINT('Ctrl Pts',(-0.31241176881403,0.417107419064298,
-1.73105973218862));
#29947=CARTESIAN_POINT('Ctrl Pts',(-0.305543769648105,0.40674449660338,
-1.71050199902501));
#29948=CARTESIAN_POINT('Ctrl Pts',(-0.299865103021684,0.398176123120899,
-1.69350425187759));
#29949=CARTESIAN_POINT('Ctrl Pts',(-0.294365904146456,0.389669138737853,
-1.67631988987948));
#29950=CARTESIAN_POINT('Ctrl Pts',(-0.288814745499404,0.380887794442087,
-1.65821341382975));
#29951=CARTESIAN_POINT('Ctrl Pts',(-0.287652050165285,0.379048533723895,
-1.65442099560521));
#29952=CARTESIAN_POINT('Ctrl Pts',(-0.286487075372004,0.377197400306006,
-1.65058804734057));
#29953=CARTESIAN_POINT('Ctrl Pts',(-0.28531769463674,0.375331578522012,
-1.64670768593927));
#29954=CARTESIAN_POINT('Ctrl Pts',(-0.278565236555438,0.3645575996085,-1.62430097364065));
#29955=CARTESIAN_POINT('Ctrl Pts',(-0.271665868697669,0.353295923028537,
-1.60031225523217));
#29956=CARTESIAN_POINT('Ctrl Pts',(-0.264753638980834,0.341806749440673,
-1.57508712196688));
#29957=CARTESIAN_POINT('Ctrl Pts',(-0.257841409264,0.330317575852808,-1.54986198870159));
#29958=CARTESIAN_POINT('Ctrl Pts',(-0.2509163176881,0.318596673571711,-1.52340229432317));
#29959=CARTESIAN_POINT('Ctrl Pts',(-0.243933082800515,0.30663613302955,
-1.49546276882618));
#29960=CARTESIAN_POINT('Ctrl Pts',(-0.23694984791293,0.294675592487389,
-1.46752324332919));
#29961=CARTESIAN_POINT('Ctrl Pts',(-0.22990846971366,0.282477015449631,
-1.43810324340019));
#29962=CARTESIAN_POINT('Ctrl Pts',(-0.222822150024723,0.270145781900204,
-1.40717063605061));
#29963=CARTESIAN_POINT('Ctrl Pts',(-0.215735830335797,0.257814548350794,
-1.37623802870107));
#29964=CARTESIAN_POINT('Ctrl Pts',(-0.208604569157203,0.245348810589579,
-1.34379351988624));
#29965=CARTESIAN_POINT('Ctrl Pts',(-0.20139409589261,0.232798729978922,
-1.30960875804952));
#29966=CARTESIAN_POINT('Ctrl Pts',(-0.194183622628007,0.220248649368249,
-1.27542399621276));
#29967=CARTESIAN_POINT('Ctrl Pts',(-0.186893937277403,0.207614742487103,
-1.23949884094976));
#29968=CARTESIAN_POINT('Ctrl Pts',(-0.179513347151867,0.195008186424988,
-1.20167966782215));
#29969=CARTESIAN_POINT('Ctrl Pts',(-0.17213275702633,0.182401630362873,
-1.16386049469453));
#29970=CARTESIAN_POINT('Ctrl Pts',(-0.16466126212586,0.169824308636727,
-1.12414663060252));
#29971=CARTESIAN_POINT('Ctrl Pts',(-0.157115542594206,0.157467963405492,
-1.08257118120827));
#29972=CARTESIAN_POINT('Ctrl Pts',(-0.149569823062563,0.145111618174274,
-1.04099573181408));
#29973=CARTESIAN_POINT('Ctrl Pts',(-0.141949878899737,0.132972291505805,
-0.997559839050705));
#29974=CARTESIAN_POINT('Ctrl Pts',(-0.134207247927528,0.121174400699684,
-0.951967546680385));
#29975=CARTESIAN_POINT('Ctrl Pts',(-0.127569153529385,0.111059555610061,
-0.912879290806096));
#29976=CARTESIAN_POINT('Ctrl Pts',(-0.120840879677674,0.101195125658457,
-0.872206528992164));
#29977=CARTESIAN_POINT('Ctrl Pts',(-0.113972151341684,0.0916740642261438,
-0.829649777958719));
#29978=CARTESIAN_POINT('Ctrl Pts',(-0.112829238751193,0.0900898203234105,
-0.822568605988117));
#29979=CARTESIAN_POINT('Ctrl Pts',(-0.1116824374202,0.0885152001390327,
-0.815435269714428));
#29980=CARTESIAN_POINT('Ctrl Pts',(-0.110531515736002,0.0869507755337904,
-0.808248387991514));
#29981=CARTESIAN_POINT('Ctrl Pts',(-0.104093298235906,0.0781994364901921,
-0.768045211428898));
#29982=CARTESIAN_POINT('Ctrl Pts',(-0.0975261447367866,0.0697631999578778,
-0.726167000035645));
#29983=CARTESIAN_POINT('Ctrl Pts',(-0.0907979124502509,0.0617629058426914,
-0.682336740815209));
#29984=CARTESIAN_POINT('Ctrl Pts',(-0.0890949413787892,0.0597379654332153,
-0.671242940790433));
#29985=CARTESIAN_POINT('Ctrl Pts',(-0.0873816509906677,0.057741210889608,
-0.660024094936211));
#29986=CARTESIAN_POINT('Ctrl Pts',(-0.0856575200882579,0.0557751425005906,
-0.648675740631271));
#29987=CARTESIAN_POINT('Ctrl Pts',(-0.0780501822835085,0.0471003102349018,
-0.59860369296656));
#29988=CARTESIAN_POINT('Ctrl Pts',(-0.0702317996002882,0.0390194097716542,
-0.546009698564737));
#29989=CARTESIAN_POINT('Ctrl Pts',(-0.0621404289527874,0.0318265887957336,
-0.490784212351215));
#29990=CARTESIAN_POINT('Ctrl Pts',(-0.0611527179057972,0.0309485634219814,
-0.484042854775988));
#29991=CARTESIAN_POINT('Ctrl Pts',(-0.0601609390631264,0.03008383072053,
-0.477262309173059));
#29992=CARTESIAN_POINT('Ctrl Pts',(-0.0591649797527023,0.0292329757968122,
-0.470442397304746));
#29993=CARTESIAN_POINT('Ctrl Pts',(-0.0514071364498713,0.0226053966351349,
-0.417319938325012));
#29994=CARTESIAN_POINT('Ctrl Pts',(-0.0433956496731836,0.0168161405436987,
-0.361807975160488));
#29995=CARTESIAN_POINT('Ctrl Pts',(-0.0351244935793345,0.0121644665601162,
-0.303812395418932));
#29996=CARTESIAN_POINT('Ctrl Pts',(-0.0336349978225925,0.0113267785051844,
-0.29336836934148));
#29997=CARTESIAN_POINT('Ctrl Pts',(-0.0321370810062191,0.0105261042260805,
-0.282843860181119));
#29998=CARTESIAN_POINT('Ctrl Pts',(-0.0306307079387777,0.00976435400706599,
-0.272238402589581));
#29999=CARTESIAN_POINT('Ctrl Pts',(-0.0215805482745863,0.00518782429120783,
-0.208521726694507));
#30000=CARTESIAN_POINT('Ctrl Pts',(-0.012225159981005,0.00201431597951373,
-0.141880460699178));
#30001=CARTESIAN_POINT('Ctrl Pts',(-0.00262039848169704,0.000690311987880055,
-0.0724285480818705));
#30002=CARTESIAN_POINT('Ctrl Pts',(-0.00174900083682787,0.000570190945812525,
-0.0661274823978614));
#30003=CARTESIAN_POINT('Ctrl Pts',(-0.000875550568057551,0.00046531029951653,
-0.0598033132919511));
#30004=CARTESIAN_POINT('Ctrl Pts',(-8.93867835446334E-8,0.000376013267725295,
-0.0534561450979849));
#30005=CARTESIAN_POINT('',(-1.33322010970278E-6,0.000376061138413409,0.0534595472478362));
#30006=CARTESIAN_POINT('Ctrl Pts',(-6.386159645368E-8,0.000376010664161264,
-0.0534559600381995));
#30007=CARTESIAN_POINT('Ctrl Pts',(-0.001454973133866,0.000313323311071578,
-0.0490001730603571));
#30008=CARTESIAN_POINT('Ctrl Pts',(-0.002708403504571,0.000259316092946519,
-0.0446031753896197));
#30009=CARTESIAN_POINT('Ctrl Pts',(-0.0037727890176825,0.00021347008401007,
-0.040278121468098));
#30010=CARTESIAN_POINT('Ctrl Pts',(-0.004837174530794,0.000167624075073621,
-0.0359530675465762));
#30011=CARTESIAN_POINT('Ctrl Pts',(-0.005712515186312,0.000129899434652782,
-0.0316999576221515));
#30012=CARTESIAN_POINT('Ctrl Pts',(-0.00641840706118967,9.94838426637834E-5,
-0.027496678112308));
#30013=CARTESIAN_POINT('Ctrl Pts',(-0.00712429893606733,6.90682506747847E-5,
-0.0232933986024644));
#30014=CARTESIAN_POINT('Ctrl Pts',(-0.00766074203030467,4.59440949101007E-5,
-0.0191399497061853));
#30015=CARTESIAN_POINT('Ctrl Pts',(-0.008040469737835,2.95933637711743E-5,
-0.0149969559875762));
#30016=CARTESIAN_POINT('Ctrl Pts',(-0.00842019744536534,1.32426326322479E-5,
-0.010853962268967));
#30017=CARTESIAN_POINT('Ctrl Pts',(-0.00864320976618867,3.62518085065978E-6,
-0.00672142386867571));
#30018=CARTESIAN_POINT('Ctrl Pts',(-0.00870785447653417,8.37616607740621E-7,
-0.00252307065227364));
#30019=CARTESIAN_POINT('Ctrl Pts',(-0.00877249918687967,-1.94994763517854E-6,
0.00167528256412843));
#30020=CARTESIAN_POINT('Ctrl Pts',(-0.00867877628674733,2.10261831921796E-6,
0.00593945050831973));
#30021=CARTESIAN_POINT('Ctrl Pts',(-0.00840122364752867,1.40468953585549E-5,
0.0103322895530075));
#30022=CARTESIAN_POINT('Ctrl Pts',(-0.00812367100831,2.59911723978918E-5,
0.0147251285976952));
#30023=CARTESIAN_POINT('Ctrl Pts',(-0.007662288630005,4.58884199110661E-5,
0.0192466386013889));
#30024=CARTESIAN_POINT('Ctrl Pts',(-0.006982466553949,7.51792644959615E-5,
0.0239030700590784));
#30025=CARTESIAN_POINT('Ctrl Pts',(-0.006302644477893,0.000104470109080857,
0.028559501516768));
#30026=CARTESIAN_POINT('Ctrl Pts',(-0.005404382704086,0.00014315841789564,
0.0333508544250512));
#30027=CARTESIAN_POINT('Ctrl Pts',(-0.00425226433895525,0.000192812210902948,
0.0382797025368775));
#30028=CARTESIAN_POINT('Ctrl Pts',(-0.0031002340599688,0.000242462207589229,
0.0432081738096228));
#30029=CARTESIAN_POINT('Ctrl Pts',(-0.00169438600579797,0.000303103761307874,
0.0482741189859386));
#30030=CARTESIAN_POINT('Ctrl Pts',(-1.29817508026421E-6,0.000376060972450354,
0.0534595358076361));
#30031=CARTESIAN_POINT('',(-0.3268604435632,0.437871921569987,1.77090225146181));
#30032=CARTESIAN_POINT('Ctrl Pts',(-9.098011382209E-7,0.000376077707954448,
0.0534607252664227));
#30033=CARTESIAN_POINT('Ctrl Pts',(-0.00956218302788966,0.00135153777727009,
0.12278977750321));
#30034=CARTESIAN_POINT('Ctrl Pts',(-0.0188675944382579,0.00418251178063798,
0.189245247763867));
#30035=CARTESIAN_POINT('Ctrl Pts',(-0.0278578211264471,0.00841146826043904,
0.252698250846818));
#30036=CARTESIAN_POINT('Ctrl Pts',(-0.0292960008120538,0.00908798060117399,
0.262848920367146));
#30037=CARTESIAN_POINT('Ctrl Pts',(-0.0307261146470735,0.00980032046044534,
0.272922849151112));
#30038=CARTESIAN_POINT('Ctrl Pts',(-0.0321479197748909,0.010546676423365,
0.282919614791902));
#30039=CARTESIAN_POINT('Ctrl Pts',(-0.0401348344435378,0.0147392913405909,
0.339075913973366));
#30040=CARTESIAN_POINT('Ctrl Pts',(-0.0478595619690656,0.020001171173114,
0.39279475688745));
#30041=CARTESIAN_POINT('Ctrl Pts',(-0.0553373273401742,0.0260513509579798,
0.444197697420766));
#30042=CARTESIAN_POINT('Ctrl Pts',(-0.057512014228688,0.0278108668023969,
0.459146722331438));
#30043=CARTESIAN_POINT('Ctrl Pts',(-0.0596658139179924,0.0296373695094689,
0.473900004286979));
#30044=CARTESIAN_POINT('Ctrl Pts',(-0.0617991008907227,0.0315247081520194,
0.488460822104781));
#30045=CARTESIAN_POINT('Ctrl Pts',(-0.0689256003236805,0.0378295878695011,
0.537102969761623));
#30046=CARTESIAN_POINT('Ctrl Pts',(-0.0758231832410947,0.0448090998317559,
0.583595570635645));
#30047=CARTESIAN_POINT('Ctrl Pts',(-0.0825535997623161,0.0522799773424927,
0.628167678070125));
#30048=CARTESIAN_POINT('Ctrl Pts',(-0.0847656203519447,0.0547353580495018,
0.642816759454217));
#30049=CARTESIAN_POINT('Ctrl Pts',(-0.0869595840318742,0.0572442360284669,
0.657258458865084));
#30050=CARTESIAN_POINT('Ctrl Pts',(-0.0891376829985573,0.0598012999793553,
0.671501068028844));
#30051=CARTESIAN_POINT('Ctrl Pts',(-0.0960094214768027,0.067868644490065,
0.716435429101639));
#30052=CARTESIAN_POINT('Ctrl Pts',(-0.10272324972924,0.0764114112181864,
0.759387035815182));
#30053=CARTESIAN_POINT('Ctrl Pts',(-0.109312534271131,0.08530222388455,
0.800637516060127));
#30054=CARTESIAN_POINT('Ctrl Pts',(-0.111166622769007,0.0878039148339511,
0.81224454873079));
#30055=CARTESIAN_POINT('Ctrl Pts',(-0.113010850602073,0.090333482418393,
0.823716907565805));
#30056=CARTESIAN_POINT('Ctrl Pts',(-0.114845961110231,0.0928888168290825,
0.835060881378789));
#30057=CARTESIAN_POINT('Ctrl Pts',(-0.122674528197928,0.10378985345693,
0.883454185019746));
#30058=CARTESIAN_POINT('Ctrl Pts',(-0.13033717192211,0.115155692463132,
0.929509774252189));
#30059=CARTESIAN_POINT('Ctrl Pts',(-0.137873485130416,0.126799435650295,
0.973446256380397));
#30060=CARTESIAN_POINT('Ctrl Pts',(-0.138382141414221,0.127585319009367,
0.976411707404667));
#30061=CARTESIAN_POINT('Ctrl Pts',(-0.138890222206121,0.128372487781146,
0.979367506754383));
#30062=CARTESIAN_POINT('Ctrl Pts',(-0.139397739679552,0.129160892803958,
0.982313722331195));
#30063=CARTESIAN_POINT('Ctrl Pts',(-0.147424697608637,0.141630402289828,
1.02891142531315));
#30064=CARTESIAN_POINT('Ctrl Pts',(-0.155310741595373,0.15440539912281,
1.07311084051338));
#30065=CARTESIAN_POINT('Ctrl Pts',(-0.16306962602991,0.167286308004598,
1.11507454100124));
#30066=CARTESIAN_POINT('Ctrl Pts',(-0.170828510464437,0.180167216886368,
1.15703824148905));
#30067=CARTESIAN_POINT('Ctrl Pts',(-0.178460235346763,0.193153903003862,
1.19676630295696));
#30068=CARTESIAN_POINT('Ctrl Pts',(-0.18598165758879,0.206100818291459,
1.23445885784609));
#30069=CARTESIAN_POINT('Ctrl Pts',(-0.193503079830827,0.219047733579073,
1.27215141273528));
#30070=CARTESIAN_POINT('Ctrl Pts',(-0.200914199432563,0.231953458456882,
1.30780888797803));
#30071=CARTESIAN_POINT('Ctrl Pts',(-0.208273146571748,0.244783459547113,
1.34180302223918));
#30072=CARTESIAN_POINT('Ctrl Pts',(-0.215632093710933,0.257613460637344,
1.37579715650034));
#30073=CARTESIAN_POINT('Ctrl Pts',(-0.222938868387567,0.270373085084809,
1.40812595456548));
#30074=CARTESIAN_POINT('Ctrl Pts',(-0.230130727084885,0.282842535025996,
1.43861161074754));
#30075=CARTESIAN_POINT('Ctrl Pts',(-0.237322585782203,0.295311984967184,
1.4690972669296));
#30076=CARTESIAN_POINT('Ctrl Pts',(-0.244399528500206,0.307485397722405,
1.49774227400769));
#30077=CARTESIAN_POINT('Ctrl Pts',(-0.251454846116976,0.319459465500557,
1.52506969929454));
#30078=CARTESIAN_POINT('Ctrl Pts',(-0.256901118650271,0.328702711516436,
1.54616479576357));
#30079=CARTESIAN_POINT('Ctrl Pts',(-0.262334505016738,0.337825935927688,
1.56647526973609));
#30080=CARTESIAN_POINT('Ctrl Pts',(-0.2679496648376,0.347106534542236,1.58667158422878));
#30081=CARTESIAN_POINT('Ctrl Pts',(-0.269608605929401,0.349848391744766,
1.59263837717569));
#30082=CARTESIAN_POINT('Ctrl Pts',(-0.271283413046643,0.352604303264488,
1.59859506771931));
#30083=CARTESIAN_POINT('Ctrl Pts',(-0.272979105942957,0.355382209947033,
1.6045585936483));
#30084=CARTESIAN_POINT('Ctrl Pts',(-0.278853400615903,0.36500555770221,
1.62521770513763));
#30085=CARTESIAN_POINT('Ctrl Pts',(-0.284978345303742,0.37488926894645,
1.64596018554789));
#30086=CARTESIAN_POINT('Ctrl Pts',(-0.291647922676962,0.385350896245332,
1.66738462816095));
#30087=CARTESIAN_POINT('Ctrl Pts',(-0.293420205285631,0.388130826529165,
1.67307766760241));
#30088=CARTESIAN_POINT('Ctrl Pts',(-0.295230944683588,0.390951814871058,
1.67881873367062));
#30089=CARTESIAN_POINT('Ctrl Pts',(-0.297085656889315,0.393820379335401,
1.68461876748693));
#30090=CARTESIAN_POINT('Ctrl Pts',(-0.3059201512701,0.407484125421129,1.71224589260116));
#30091=CARTESIAN_POINT('Ctrl Pts',(-0.3157523331598,0.422231828276934,1.74120891476497));
#30092=CARTESIAN_POINT('Ctrl Pts',(-0.3268604435632,0.437871921569987,1.77090225146181));
#30093=CARTESIAN_POINT('',(-0.500000000199844,0.97322574578055,2.53955651948966));
#30094=CARTESIAN_POINT('Ctrl Pts',(-0.326860601705563,0.437872144139036,
1.7709026740179));
#30095=CARTESIAN_POINT('Ctrl Pts',(-0.343264928911304,0.460959547950471,
1.81473501139747));
#30096=CARTESIAN_POINT('Ctrl Pts',(-0.358589100390692,0.484717356933362,
1.85775178565521));
#30097=CARTESIAN_POINT('Ctrl Pts',(-0.372741964402922,0.508903336490866,
1.89965332401442));
#30098=CARTESIAN_POINT('Ctrl Pts',(-0.380698914410039,0.522501052829122,
1.92321099019828));
#30099=CARTESIAN_POINT('Ctrl Pts',(-0.388285631095653,0.536233297733624,
1.94641668345229));
#30100=CARTESIAN_POINT('Ctrl Pts',(-0.39548591606965,0.550051242464931,
1.9692214383853));
#30101=CARTESIAN_POINT('Ctrl Pts',(-0.405489578841325,0.569249101964776,
2.00090505629269));
#30102=CARTESIAN_POINT('Ctrl Pts',(-0.414747322949087,0.588607187415817,
2.03181712306189));
#30103=CARTESIAN_POINT('Ctrl Pts',(-0.42335439481679,0.608360124090959,
2.06238573077572));
#30104=CARTESIAN_POINT('Ctrl Pts',(-0.431961466684492,0.628113060766101,
2.09295433848956));
#30105=CARTESIAN_POINT('Ctrl Pts',(-0.439917866312133,0.648261031775009,
2.123179700578));
#30106=CARTESIAN_POINT('Ctrl Pts',(-0.447318840123567,0.669087264136625,
2.15345894792739));
#30107=CARTESIAN_POINT('Ctrl Pts',(-0.45421077773461,0.688481076054676,
2.18165560001105));
#30108=CARTESIAN_POINT('Ctrl Pts',(-0.460621065969921,0.708461418171445,
2.20989678565934));
#30109=CARTESIAN_POINT('Ctrl Pts',(-0.466459965279737,0.729327019690268,
2.23851903007228));
#30110=CARTESIAN_POINT('Ctrl Pts',(-0.472128453601352,0.749583648937855,
2.2663059209886));
#30111=CARTESIAN_POINT('Ctrl Pts',(-0.477258418795676,0.770674668551129,
2.29445219657496));
#30112=CARTESIAN_POINT('Ctrl Pts',(-0.481767751497067,0.792911044852894,
2.32323395632732));
#30113=CARTESIAN_POINT('Ctrl Pts',(-0.482589455892488,0.796963025346541,
2.32847865661062));
#30114=CARTESIAN_POINT('Ctrl Pts',(-0.483390552035199,0.801053140541715,
2.33374436452152));
#30115=CARTESIAN_POINT('Ctrl Pts',(-0.484170543101058,0.805183411400594,
2.33903262068955));
#30116=CARTESIAN_POINT('Ctrl Pts',(-0.490194241371115,0.83708057858172,
2.37987265197359));
#30117=CARTESIAN_POINT('Ctrl Pts',(-0.494959205242138,0.871375098538481,
2.42205463170978));
#30118=CARTESIAN_POINT('Ctrl Pts',(-0.497629691854722,0.908027737205445,
2.46505505642915));
#30119=CARTESIAN_POINT('Ctrl Pts',(-0.499157324262198,0.928994612075099,
2.48965313605516));
#30120=CARTESIAN_POINT('Ctrl Pts',(-0.499999574874154,0.950732289475268,
2.51451910737286));
#30121=CARTESIAN_POINT('Ctrl Pts',(-0.500000000001591,0.973225745780587,
2.53955651948963));
#30122=CARTESIAN_POINT('',(-0.499999999994609,0.973224638042631,-2.53955528646987));
#30123=CARTESIAN_POINT('Origin',(-0.5,3.8,0.));
#30124=CARTESIAN_POINT('Ctrl Pts',(-0.499999999983828,0.973224638043246,
-2.53955528646932));
#30125=CARTESIAN_POINT('Ctrl Pts',(-0.499999467882099,0.941147572377687,
-2.50385035049475));
#30126=CARTESIAN_POINT('Ctrl Pts',(-0.498254574300839,0.910151441566798,
-2.46798114716292));
#30127=CARTESIAN_POINT('Ctrl Pts',(-0.495166769763196,0.880433227438514,
-2.43230957333866));
#30128=CARTESIAN_POINT('Ctrl Pts',(-0.493039810620746,0.859962557593052,
-2.40773807629404));
#30129=CARTESIAN_POINT('Ctrl Pts',(-0.49027566594079,0.84009728363555,-2.38326105062791));
#30130=CARTESIAN_POINT('Ctrl Pts',(-0.487005543648317,0.820889599255338,
-2.35900428574748));
#30131=CARTESIAN_POINT('Ctrl Pts',(-0.483408131607902,0.799759516378343,
-2.33231978583039));
#30132=CARTESIAN_POINT('Ctrl Pts',(-0.479198392185239,0.77942166446121,
-2.30590616238722));
#30133=CARTESIAN_POINT('Ctrl Pts',(-0.474372740319575,0.759556839873406,
-2.27940900016636));
#30134=CARTESIAN_POINT('Ctrl Pts',(-0.469513754567056,0.739554796142232,
-2.25272880497254));
#30135=CARTESIAN_POINT('Ctrl Pts',(-0.464030317974717,0.72003223987174,
-2.22596369837556));
#30136=CARTESIAN_POINT('Ctrl Pts',(-0.457918770674461,0.700704659399275,
-2.19871971650109));
#30137=CARTESIAN_POINT('Ctrl Pts',(-0.456572555292686,0.696447294636109,
-2.19271857380214));
#30138=CARTESIAN_POINT('Ctrl Pts',(-0.455195863561821,0.692199552781376,
-2.18669407899222));
#30139=CARTESIAN_POINT('Ctrl Pts',(-0.453788656365767,0.687958672214371,
-2.18064182619573));
#30140=CARTESIAN_POINT('Ctrl Pts',(-0.445663500202611,0.663472003177413,
-2.14569636880452));
#30141=CARTESIAN_POINT('Ctrl Pts',(-0.436521001197423,0.639212875904072,
-2.10983035256481));
#30142=CARTESIAN_POINT('Ctrl Pts',(-0.426223710361425,0.615068477761928,
-2.0727303728788));
#30143=CARTESIAN_POINT('Ctrl Pts',(-0.418600565927401,0.597194239067346,
-2.04526504164263));
#30144=CARTESIAN_POINT('Ctrl Pts',(-0.410344534688079,0.579383691340677,
-2.01712292969517));
#30145=CARTESIAN_POINT('Ctrl Pts',(-0.401399849929217,0.561607734175777,
-1.98816888936777));
#30146=CARTESIAN_POINT('Ctrl Pts',(-0.385702969888419,0.530412999565221,
-1.93735792062286));
#30147=CARTESIAN_POINT('Ctrl Pts',(-0.367885301289346,0.499330809129928,
-1.88404149274837));
#30148=CARTESIAN_POINT('Ctrl Pts',(-0.347930442098136,0.468787969912562,
-1.82839448987376));
#30149=CARTESIAN_POINT('Ctrl Pts',(-0.34115432792523,0.458416472738944,
-1.80949831820724));
#30150=CARTESIAN_POINT('Ctrl Pts',(-0.334131775937924,0.448106966312162,
-1.79033379514828));
#30151=CARTESIAN_POINT('Ctrl Pts',(-0.3268621439014,0.437875462608086,-1.77090897424662));
#30152=CARTESIAN_POINT('Origin',(0.,3.8,0.));
#30153=CARTESIAN_POINT('',(-1.3332021415609E-6,7.59962393886241,-0.0534595471885383));
#30154=CARTESIAN_POINT('Ctrl Pts',(-9.097914536952E-7,7.5996239222932,-0.0534607251840784));
#30155=CARTESIAN_POINT('Ctrl Pts',(-0.00956218223484543,7.5986484623053,
-0.122789771741156));
#30156=CARTESIAN_POINT('Ctrl Pts',(-0.0188675928807159,7.59581748869241,
-0.189245236636373));
#30157=CARTESIAN_POINT('Ctrl Pts',(-0.0278578188629172,7.5915885328044,
-0.252698234869587));
#30158=CARTESIAN_POINT('Ctrl Pts',(-0.0292959993115927,7.59091202014626,
-0.262848909796949));
#30159=CARTESIAN_POINT('Ctrl Pts',(-0.0307261139013526,7.59019967993104,
-0.272922843907623));
#30160=CARTESIAN_POINT('Ctrl Pts',(-0.0321479197753001,7.58945332357642,
-0.282919614794823));
#30161=CARTESIAN_POINT('Ctrl Pts',(-0.0401348345801153,7.58526070858752,
-0.339075914935605));
#30162=CARTESIAN_POINT('Ctrl Pts',(-0.0478595622363532,7.57999882864497,
-0.39279475874736));
#30163=CARTESIAN_POINT('Ctrl Pts',(-0.0553373277299044,7.57394864872664,
-0.444197700100289));
#30164=CARTESIAN_POINT('Ctrl Pts',(-0.0575120144862837,7.57218913297912,
-0.459146724096235));
#30165=CARTESIAN_POINT('Ctrl Pts',(-0.0596658140459766,7.57036263037731,
-0.473900005160658));
#30166=CARTESIAN_POINT('Ctrl Pts',(-0.0617991008914628,7.56847529184733,
-0.488460822109806));
#30167=CARTESIAN_POINT('Ctrl Pts',(-0.0689256002967675,7.56217041215431,
-0.53710296957742));
#30168=CARTESIAN_POINT('Ctrl Pts',(-0.0758231831874148,7.55519090022252,
-0.583595570273457));
#30169=CARTESIAN_POINT('Ctrl Pts',(-0.0825535996829062,7.54772002274568,
-0.628167677544045));
#30170=CARTESIAN_POINT('Ctrl Pts',(-0.0847656202997536,7.54526464201022,
-0.642816759110531));
#30171=CARTESIAN_POINT('Ctrl Pts',(-0.0869595840064315,7.54275576400144,
-0.657258458698621));
#30172=CARTESIAN_POINT('Ctrl Pts',(-0.089137682999504,7.54019870001955,
-0.671501068034935));
#30173=CARTESIAN_POINT('Ctrl Pts',(-0.0960094214851858,7.53213135550004,
-0.716435429156335));
#30174=CARTESIAN_POINT('Ctrl Pts',(-0.102723249744971,7.52358858876181,
-0.759387035915678));
#30175=CARTESIAN_POINT('Ctrl Pts',(-0.109312534293958,7.51469777608467,
-0.800637516202912));
#30176=CARTESIAN_POINT('Ctrl Pts',(-0.111166622784501,7.51219608514483,
-0.812244548827073));
#30177=CARTESIAN_POINT('Ctrl Pts',(-0.113010850610315,7.50966651757017,
-0.823716907616661));
#30178=CARTESIAN_POINT('Ctrl Pts',(-0.114845961111285,7.50711118316948,
-0.835060881385187));
#30179=CARTESIAN_POINT('Ctrl Pts',(-0.122674528194227,7.49621014654818,
-0.883454184996663));
#30180=CARTESIAN_POINT('Ctrl Pts',(-0.130337171913731,7.48484430754926,
-0.92950977420178));
#30181=CARTESIAN_POINT('Ctrl Pts',(-0.13787348511751,7.47320056436962,-0.973446256305266));
#30182=CARTESIAN_POINT('Ctrl Pts',(-0.138382141405972,7.47241468100338,
-0.976411707356797));
#30183=CARTESIAN_POINT('Ctrl Pts',(-0.138890222202518,7.47162751222442,
-0.979367506733599));
#30184=CARTESIAN_POINT('Ctrl Pts',(-0.139397739680585,7.4708391071944,-0.982313722337323));
#30185=CARTESIAN_POINT('Ctrl Pts',(-0.147424697609637,7.45836959770851,
-1.02891142531904));
#30186=CARTESIAN_POINT('Ctrl Pts',(-0.155310741596374,7.44559460087546,
-1.07311084051926));
#30187=CARTESIAN_POINT('Ctrl Pts',(-0.16306962603091,7.43271369199364,-1.11507454100697));
#30188=CARTESIAN_POINT('Ctrl Pts',(-0.170828510465437,7.41983278311185,
-1.15703824149462));
#30189=CARTESIAN_POINT('Ctrl Pts',(-0.178460235347763,7.40684609699437,
-1.19676630296227));
#30190=CARTESIAN_POINT('Ctrl Pts',(-0.18598165758979,7.39389918170677,-1.23445885785126));
#30191=CARTESIAN_POINT('Ctrl Pts',(-0.193503079831827,7.38095226641914,
-1.27215141274029));
#30192=CARTESIAN_POINT('Ctrl Pts',(-0.200914199433564,7.36804654154129,
-1.30780888798301));
#30193=CARTESIAN_POINT('Ctrl Pts',(-0.208273146572715,7.35521654045108,
-1.34180302224396));
#30194=CARTESIAN_POINT('Ctrl Pts',(-0.215632093711867,7.34238653936088,
-1.37579715650491));
#30195=CARTESIAN_POINT('Ctrl Pts',(-0.222938868388433,7.32962691491351,
-1.40812595456969));
#30196=CARTESIAN_POINT('Ctrl Pts',(-0.230130727085702,7.31715746497242,
-1.43861161075141));
#30197=CARTESIAN_POINT('Ctrl Pts',(-0.23732258578297,7.30468801503134,-1.46909726693312));
#30198=CARTESIAN_POINT('Ctrl Pts',(-0.244399528500939,7.29251460227622,
-1.49774227401089));
#30199=CARTESIAN_POINT('Ctrl Pts',(-0.251454846117659,7.28054053449819,
-1.52506969929741));
#30200=CARTESIAN_POINT('Ctrl Pts',(-0.25690111865087,7.27129728848248,-1.546164795766));
#30201=CARTESIAN_POINT('Ctrl Pts',(-0.262334505017244,7.2621740640714,-1.56647526973809));
#30202=CARTESIAN_POINT('Ctrl Pts',(-0.267949664838005,7.25289346545703,
-1.58667158423037));
#30203=CARTESIAN_POINT('Ctrl Pts',(-0.269608605929838,7.25015160825446,
-1.59263837717737));
#30204=CARTESIAN_POINT('Ctrl Pts',(-0.271283413047111,7.24739569673469,
-1.59859506772109));
#30205=CARTESIAN_POINT('Ctrl Pts',(-0.272979105943457,7.24461779005209,
-1.60455859365018));
#30206=CARTESIAN_POINT('Ctrl Pts',(-0.278853400616557,7.23499444229667,
-1.62521770514));
#30207=CARTESIAN_POINT('Ctrl Pts',(-0.28497834530457,7.22511073105216,-1.64596018555078));
#30208=CARTESIAN_POINT('Ctrl Pts',(-0.291647922678002,7.21464910375299,
-1.6673846281644));
#30209=CARTESIAN_POINT('Ctrl Pts',(-0.29342020528643,7.21186917346954,-1.67307766760504));
#30210=CARTESIAN_POINT('Ctrl Pts',(-0.295230944684135,7.20904818512805,
-1.67881873367243));
#30211=CARTESIAN_POINT('Ctrl Pts',(-0.297085656889598,7.20617962066412,
-1.68461876748789));
#30212=CARTESIAN_POINT('Ctrl Pts',(-0.3059201512703,7.19251587457857,-1.71224589260175));
#30213=CARTESIAN_POINT('Ctrl Pts',(-0.3157523331599,7.177768171723,-1.7412089147651));
#30214=CARTESIAN_POINT('Ctrl Pts',(-0.3268604435631,7.16212807842995,-1.77090225146193));
#30215=CARTESIAN_POINT('',(-0.499999999994609,6.62677536195992,2.53955528646714));
#30216=CARTESIAN_POINT('Origin',(-0.5,3.8,0.));
#30217=CARTESIAN_POINT('',(-0.326861933644355,7.16212485193451,1.77090837708044));
#30218=CARTESIAN_POINT('Ctrl Pts',(-0.499999999983828,6.62677536195925,
2.53955528646654));
#30219=CARTESIAN_POINT('Ctrl Pts',(-0.499999467882044,6.65885242763283,
2.50385035048297));
#30220=CARTESIAN_POINT('Ctrl Pts',(-0.498254574299847,6.68984855845096,
2.46798114714233));
#30221=CARTESIAN_POINT('Ctrl Pts',(-0.495166769760691,6.71956677258583,
2.43230957330944));
#30222=CARTESIAN_POINT('Ctrl Pts',(-0.493039810618576,6.74003744242258,
2.40773807627478));
#30223=CARTESIAN_POINT('Ctrl Pts',(-0.490275665939506,6.75990271637183,
2.38326105061858));
#30224=CARTESIAN_POINT('Ctrl Pts',(-0.487005543648317,6.7791104007444,2.35900428574781));
#30225=CARTESIAN_POINT('Ctrl Pts',(-0.483408131607721,6.80024048362235,
2.33231978582952));
#30226=CARTESIAN_POINT('Ctrl Pts',(-0.479198392184817,6.82057833554045,
2.30590616238507));
#30227=CARTESIAN_POINT('Ctrl Pts',(-0.474372740318849,6.84044316012923,
2.27940900016284));
#30228=CARTESIAN_POINT('Ctrl Pts',(-0.469513754566043,6.86044520386132,
2.25272880496774));
#30229=CARTESIAN_POINT('Ctrl Pts',(-0.46403031797336,6.87996776013273,2.2259636983694));
#30230=CARTESIAN_POINT('Ctrl Pts',(-0.457918770672701,6.89929534060611,
2.1987197164935));
#30231=CARTESIAN_POINT('Ctrl Pts',(-0.456572555291486,6.90355270536742,
2.19271857379713));
#30232=CARTESIAN_POINT('Ctrl Pts',(-0.455195863561208,6.90780044722032,
2.1866940789898));
#30233=CARTESIAN_POINT('Ctrl Pts',(-0.453788656365767,6.91204132778548,
2.18064182619594));
#30234=CARTESIAN_POINT('Ctrl Pts',(-0.44566350020286,6.93652799682176,2.14569636880571));
#30235=CARTESIAN_POINT('Ctrl Pts',(-0.436521001197984,6.96078712409439,
2.10983035256709));
#30236=CARTESIAN_POINT('Ctrl Pts',(-0.426223710362374,6.98493152223582,
2.07273037288226));
#30237=CARTESIAN_POINT('Ctrl Pts',(-0.418600565928086,7.00280576093116,
2.04526504164499));
#30238=CARTESIAN_POINT('Ctrl Pts',(-0.41034453468845,7.02061630865858,2.01712292969638));
#30239=CARTESIAN_POINT('Ctrl Pts',(-0.401399849929217,7.03839226582423,
1.98816888936776));
#30240=CARTESIAN_POINT('Ctrl Pts',(-0.3857029698909,7.06958700042988,1.93735792063084));
#30241=CARTESIAN_POINT('Ctrl Pts',(-0.367885301294979,7.10066919086031,
1.8840414927651));
#30242=CARTESIAN_POINT('Ctrl Pts',(-0.347930442107598,7.13121203007297,
1.82839448990012));
#30243=CARTESIAN_POINT('Ctrl Pts',(-0.341154327931767,7.14158352725146,
1.80949831822508));
#30244=CARTESIAN_POINT('Ctrl Pts',(-0.334131775941308,7.15189303368305,
1.79033379515737));
#30245=CARTESIAN_POINT('Ctrl Pts',(-0.3268621439014,7.16212453739185,1.77090897424674));
#30246=CARTESIAN_POINT('',(-3.64874277834443E-8,7.59962390164863,0.0534561363041487));
#30247=CARTESIAN_POINT('Ctrl Pts',(-0.326861921820406,7.16212485010976,
1.77090838054216));
#30248=CARTESIAN_POINT('Ctrl Pts',(-0.31954228299043,7.17243182436564,1.75134026812263));
#30249=CARTESIAN_POINT('Ctrl Pts',(-0.312411768814016,7.18289258093581,
1.73105973218841));
#30250=CARTESIAN_POINT('Ctrl Pts',(-0.305543769648105,7.19325550339669,
1.71050199902487));
#30251=CARTESIAN_POINT('Ctrl Pts',(-0.299865103021706,7.20182387687912,
1.69350425187754));
#30252=CARTESIAN_POINT('Ctrl Pts',(-0.294365904146499,7.21033086126211,
1.67631988987955));
#30253=CARTESIAN_POINT('Ctrl Pts',(-0.288814745499469,7.21911220555782,
1.65821341382993));
#30254=CARTESIAN_POINT('Ctrl Pts',(-0.287652050165329,7.22095146627604,
1.65442099560534));
#30255=CARTESIAN_POINT('Ctrl Pts',(-0.286487075372026,7.22280259969396,
1.65058804734064));
#30256=CARTESIAN_POINT('Ctrl Pts',(-0.28531769463674,7.22466842147799,1.64670768593927));
#30257=CARTESIAN_POINT('Ctrl Pts',(-0.278565236555438,7.23544240039147,
1.6243009736407));
#30258=CARTESIAN_POINT('Ctrl Pts',(-0.271665868697669,7.24670407697142,
1.60031225523227));
#30259=CARTESIAN_POINT('Ctrl Pts',(-0.264753638980818,7.25819325055929,
1.57508712196697));
#30260=CARTESIAN_POINT('Ctrl Pts',(-0.257841409263967,7.26968242414716,
1.54986198870167));
#30261=CARTESIAN_POINT('Ctrl Pts',(-0.250916317688033,7.28140332642829,
1.52340229432317));
#30262=CARTESIAN_POINT('Ctrl Pts',(-0.243933082800448,7.29336386697047,
1.49546276882614));
#30263=CARTESIAN_POINT('Ctrl Pts',(-0.236949847912863,7.30532440751264,
1.46752324332912));
#30264=CARTESIAN_POINT('Ctrl Pts',(-0.229908469713627,7.3175229845504,1.43810324340012));
#30265=CARTESIAN_POINT('Ctrl Pts',(-0.222822150024707,7.32985421809982,
1.40717063605055));
#30266=CARTESIAN_POINT('Ctrl Pts',(-0.215735830335797,7.34218545164923,
1.37623802870101));
#30267=CARTESIAN_POINT('Ctrl Pts',(-0.208604569157203,7.35465118941044,
1.34379351988619));
#30268=CARTESIAN_POINT('Ctrl Pts',(-0.20139409589261,7.3672012700211,1.30960875804947));
#30269=CARTESIAN_POINT('Ctrl Pts',(-0.194183622628007,7.37975135063177,
1.27542399621269));
#30270=CARTESIAN_POINT('Ctrl Pts',(-0.186893937277403,7.39238525751293,
1.23949884094967));
#30271=CARTESIAN_POINT('Ctrl Pts',(-0.179513347151867,7.40499181357504,
1.20167966782207));
#30272=CARTESIAN_POINT('Ctrl Pts',(-0.17213275702633,7.41759836963715,1.16386049469447));
#30273=CARTESIAN_POINT('Ctrl Pts',(-0.16466126212586,7.43017569136328,1.1241466306025));
#30274=CARTESIAN_POINT('Ctrl Pts',(-0.157115542594223,7.4425320365945,1.08257118120829));
#30275=CARTESIAN_POINT('Ctrl Pts',(-0.149569823062597,7.45488838182571,
1.04099573181413));
#30276=CARTESIAN_POINT('Ctrl Pts',(-0.141949878899804,7.46702770849417,
0.997559839050793));
#30277=CARTESIAN_POINT('Ctrl Pts',(-0.134207247927611,7.47882559930028,
0.951967546680531));
#30278=CARTESIAN_POINT('Ctrl Pts',(-0.127569153529608,7.4889404443897,0.912879290807032));
#30279=CARTESIAN_POINT('Ctrl Pts',(-0.120840879678029,7.49880487434111,
0.872206528993969));
#30280=CARTESIAN_POINT('Ctrl Pts',(-0.113972151342168,7.50832593577324,
0.829649777961458));
#30281=CARTESIAN_POINT('Ctrl Pts',(-0.112829238751547,7.50991017967616,
0.822568605990071));
#30282=CARTESIAN_POINT('Ctrl Pts',(-0.111682437420423,7.51148479986071,
0.815435269715585));
#30283=CARTESIAN_POINT('Ctrl Pts',(-0.110531515736092,7.51304922446613,
0.808248387991861));
#30284=CARTESIAN_POINT('Ctrl Pts',(-0.104093298236056,7.52180056350963,
0.768045211429718));
#30285=CARTESIAN_POINT('Ctrl Pts',(-0.0975261447369932,7.53023680004186,
0.726167000036956));
#30286=CARTESIAN_POINT('Ctrl Pts',(-0.0907979124505207,7.53823709415698,
0.682336740817026));
#30287=CARTESIAN_POINT('Ctrl Pts',(-0.0890949413789858,7.54026203456654,
0.671242940791797));
#30288=CARTESIAN_POINT('Ctrl Pts',(-0.0873816509907904,7.54225878911023,
0.660024094937112));
#30289=CARTESIAN_POINT('Ctrl Pts',(-0.0856575200883063,7.54422485749934,
0.648675740631694));
#30290=CARTESIAN_POINT('Ctrl Pts',(-0.0780501822834028,7.5528996897652,
0.598603692966023));
#30291=CARTESIAN_POINT('Ctrl Pts',(-0.0702317996000271,7.5609805902286,
0.546009698563104));
#30292=CARTESIAN_POINT('Ctrl Pts',(-0.0621404289523591,7.56817341120464,
0.490784212348375));
#30293=CARTESIAN_POINT('Ctrl Pts',(-0.0611527179055199,7.56905143657825,
0.48404285477417));
#30294=CARTESIAN_POINT('Ctrl Pts',(-0.0601609390630012,7.56991616927957,
0.477262309172276));
#30295=CARTESIAN_POINT('Ctrl Pts',(-0.0591649797527306,7.57076702420316,
0.47044239730501));
#30296=CARTESIAN_POINT('Ctrl Pts',(-0.0514071364497827,7.57739460336494,
0.417319938324441));
#30297=CARTESIAN_POINT('Ctrl Pts',(-0.0433956496729695,7.58318385945646,
0.361807975159004));
#30298=CARTESIAN_POINT('Ctrl Pts',(-0.0351244935789875,7.58783553344008,
0.30381239541647));
#30299=CARTESIAN_POINT('Ctrl Pts',(-0.0336349978223634,7.58867322149494,
0.293368369339836));
#30300=CARTESIAN_POINT('Ctrl Pts',(-0.0321370810061093,7.58947389577398,
0.282843860180307));
#30301=CARTESIAN_POINT('Ctrl Pts',(-0.0306307079387886,7.59023564599293,
0.272238402589614));
#30302=CARTESIAN_POINT('Ctrl Pts',(-0.0215805482817282,7.59481217570519,
0.20852172674472));
#30303=CARTESIAN_POINT('Ctrl Pts',(-0.0122251599957601,7.59798568401548,
0.141880460804193));
#30304=CARTESIAN_POINT('Ctrl Pts',(-0.0026203985044172,7.59930968800899,
0.0724285482460437));
#30305=CARTESIAN_POINT('Ctrl Pts',(-0.00174900018331175,7.59942980914455,
0.0661274776723202));
#30306=CARTESIAN_POINT('Ctrl Pts',(-0.000875549235118814,7.59953468986068,
0.0598033036408318));
#30307=CARTESIAN_POINT('Ctrl Pts',(-8.73713329792359E-8,7.59962398693785,
0.0534561304856728));
#30308=CARTESIAN_POINT('Ctrl Pts',(-6.386159488164E-8,7.59962398933584,
0.053455960038065));
#30309=CARTESIAN_POINT('Ctrl Pts',(-0.001454973167811,7.59968667669039,
0.0490001729562442));
#30310=CARTESIAN_POINT('Ctrl Pts',(-0.0027084035629715,7.59974068390958,
0.0446031751838687));
#30311=CARTESIAN_POINT('Ctrl Pts',(-0.00377278909219608,7.59978652991921,
0.0402781211647162));
#30312=CARTESIAN_POINT('Ctrl Pts',(-0.00483717462142067,7.59983237592883,
0.0359530671455637));
#30313=CARTESIAN_POINT('Ctrl Pts',(-0.00571251528470933,7.59987010056958,
0.031699957127514));
#30314=CARTESIAN_POINT('Ctrl Pts',(-0.00641840715996133,7.59990051616159,
0.0274966775244882));
#30315=CARTESIAN_POINT('Ctrl Pts',(-0.00712429903521333,7.5999309317536,
0.0232933979214624));
#30316=CARTESIAN_POINT('Ctrl Pts',(-0.00766074212242867,7.59995405590909,
0.0191399489324386));
#30317=CARTESIAN_POINT('Ctrl Pts',(-0.008040469817144,7.59997040663964,
0.0149969551230673));
#30318=CARTESIAN_POINT('Ctrl Pts',(-0.00842019751185934,7.5999867573702,
0.0108539613136959));
#30319=CARTESIAN_POINT('Ctrl Pts',(-0.00864320981407467,7.59999637482113,
0.00672142282462303));
#30320=CARTESIAN_POINT('Ctrl Pts',(-0.008707854494372,7.59999916238416,
0.00252306949195798));
#30321=CARTESIAN_POINT('Ctrl Pts',(-0.00877249917466933,7.6000019499472,
-0.00167528384070706));
#30322=CARTESIAN_POINT('Ctrl Pts',(-0.00867877623304867,7.59999789737958,
-0.00593945192864444));
#30323=CARTESIAN_POINT('Ctrl Pts',(-0.0084012235511355,7.5999859531005,
-0.0103322910770659));
#30324=CARTESIAN_POINT('Ctrl Pts',(-0.00812367086922233,7.59997400882142,
-0.0147251302254874));
#30325=CARTESIAN_POINT('Ctrl Pts',(-0.00766228844701667,7.59995411157182,
-0.0192466402929024));
#30326=CARTESIAN_POINT('Ctrl Pts',(-0.00698246627103333,7.59992482072332,
-0.0239030719956763));
#30327=CARTESIAN_POINT('Ctrl Pts',(-0.00630264409505,7.59989552987482,-0.0285595036984501));
#30328=CARTESIAN_POINT('Ctrl Pts',(-0.005404382165289,7.59985684155893,
-0.0333508570331727));
#30329=CARTESIAN_POINT('Ctrl Pts',(-0.0042522637803775,7.59980718776503,
-0.038279704925825));
#30330=CARTESIAN_POINT('Ctrl Pts',(-0.0031002334799121,7.59975753776738,
-0.0432081759866854));
#30331=CARTESIAN_POINT('Ctrl Pts',(-0.00169438553966578,7.59969689622004,
-0.0482741203060225));
#30332=CARTESIAN_POINT('Ctrl Pts',(-1.29815779802503E-6,7.59962393902838,
-0.0534595357485616));
#30333=CARTESIAN_POINT('Origin',(0.,3.8,0.));
#30334=CARTESIAN_POINT('',(-0.5,2.02155349221333,-3.35814353757271));
#30335=CARTESIAN_POINT('Origin',(-0.5,3.8,0.));
#30336=CARTESIAN_POINT('',(-0.2886751345948,3.80000000040883,-3.8));
#30337=CARTESIAN_POINT('Ctrl Pts',(-0.4330127018922,5.076816196554,-3.57906976744201));
#30338=CARTESIAN_POINT('Ctrl Pts',(-0.421461672428874,5.02725333529887,
-3.59675108356883));
#30339=CARTESIAN_POINT('Ctrl Pts',(-0.410577745135395,4.97711104164099,
-3.61347395830865));
#30340=CARTESIAN_POINT('Ctrl Pts',(-0.400383395751461,4.92671602852758,
-3.62911986452074));
#30341=CARTESIAN_POINT('Ctrl Pts',(-0.390148390356685,4.87612003542787,
-3.64482816805792));
#30342=CARTESIAN_POINT('Ctrl Pts',(-0.38060847404043,4.82526964336495,-3.65945078408262));
#30343=CARTESIAN_POINT('Ctrl Pts',(-0.37178639252225,4.77451034843562,-3.67291840105275));
#30344=CARTESIAN_POINT('Ctrl Pts',(-0.366141025004971,4.74202879924528,
-3.68153650860726));
#30345=CARTESIAN_POINT('Ctrl Pts',(-0.360789602986865,4.70958483923676,
-3.68968269340426));
#30346=CARTESIAN_POINT('Ctrl Pts',(-0.355738086699606,4.67727116194173,
-3.69734976820227));
#30347=CARTESIAN_POINT('Ctrl Pts',(-0.349682038096245,4.63853166490287,
-3.70654149895834));
#30348=CARTESIAN_POINT('Ctrl Pts',(-0.344057031854475,4.59998676204821,
-3.71504840903257));
#30349=CARTESIAN_POINT('Ctrl Pts',(-0.338840070970698,4.56124717707513,
-3.7229696124727));
#30350=CARTESIAN_POINT('Ctrl Pts',(-0.333642550907729,4.52265195379967,
-3.73086129782748));
#30351=CARTESIAN_POINT('Ctrl Pts',(-0.328850040735808,4.48386323128829,
-3.73817168621647));
#30352=CARTESIAN_POINT('Ctrl Pts',(-0.324439799587048,4.44448617446809,
-3.7449482734638));
#30353=CARTESIAN_POINT('Ctrl Pts',(-0.320114530549047,4.40586779535293,
-3.75159429621302));
#30354=CARTESIAN_POINT('Ctrl Pts',(-0.316156942085466,4.36668328229687,
-3.7577269598045));
#30355=CARTESIAN_POINT('Ctrl Pts',(-0.312545582610481,4.3265544635123,-3.76334165296685));
#30356=CARTESIAN_POINT('Ctrl Pts',(-0.310835779677329,4.30755542103619,
-3.76599993689129));
#30357=CARTESIAN_POINT('Ctrl Pts',(-0.309203586104177,4.28834464558913,
-3.76854138443604));
#30358=CARTESIAN_POINT('Ctrl Pts',(-0.307646725297922,4.26888179333454,
-3.77096139782409));
#30359=CARTESIAN_POINT('Ctrl Pts',(-0.303204116915783,4.21334321838992,
-3.77786707090637));
#30360=CARTESIAN_POINT('Ctrl Pts',(-0.299374932036076,4.15576288358911,
-3.78377686396753));
#30361=CARTESIAN_POINT('Ctrl Pts',(-0.296343544491563,4.09649174472707,
-3.78841558508418));
#30362=CARTESIAN_POINT('Ctrl Pts',(-0.29341632601102,4.03925736921679,-3.79289490354127));
#30363=CARTESIAN_POINT('Ctrl Pts',(-0.291233016738444,3.98044673527077,
-3.79618867850224));
#30364=CARTESIAN_POINT('Ctrl Pts',(-0.289959628991768,3.92039772486898,
-3.79809220370522));
#30365=CARTESIAN_POINT('Ctrl Pts',(-0.289119295393155,3.88077020282327,
-3.7993483773947));
#30366=CARTESIAN_POINT('Ctrl Pts',(-0.288675227111371,3.84060382170757,
-3.79999999999563));
#30367=CARTESIAN_POINT('Ctrl Pts',(-0.288675134594801,3.80000000040882,
-3.8));
#30368=CARTESIAN_POINT('',(-0.433012748163602,2.52318359238809,-3.57906969214748));
#30369=CARTESIAN_POINT('Ctrl Pts',(-0.2886751345948,3.799999999988,-3.8));
#30370=CARTESIAN_POINT('Ctrl Pts',(-0.288675077415421,3.74533021445964,
-3.79999999999983));
#30371=CARTESIAN_POINT('Ctrl Pts',(-0.289487908451124,3.69041088673595,
-3.79881587771527));
#30372=CARTESIAN_POINT('Ctrl Pts',(-0.291063540487692,3.63558198909325,
-3.79644132282977));
#30373=CARTESIAN_POINT('Ctrl Pts',(-0.292642987709118,3.58062033051703,
-3.79406101827327));
#30374=CARTESIAN_POINT('Ctrl Pts',(-0.294988934447464,3.52574990970548,
-3.79048451816112));
#30375=CARTESIAN_POINT('Ctrl Pts',(-0.298050928768093,3.47131045792295,
-3.78575794061495));
#30376=CARTESIAN_POINT('Ctrl Pts',(-0.299717636057897,3.4416779303485,-3.78318516600236));
#30377=CARTESIAN_POINT('Ctrl Pts',(-0.301596497624397,3.41217301177703,
-3.78027255366643));
#30378=CARTESIAN_POINT('Ctrl Pts',(-0.303679376872831,3.38284956903489,
-3.77703395774325));
#30379=CARTESIAN_POINT('Ctrl Pts',(-0.306623102617713,3.34140685295161,
-3.77245686178173));
#30380=CARTESIAN_POINT('Ctrl Pts',(-0.309974334650717,3.30033191238049,
-3.76723435458545));
#30381=CARTESIAN_POINT('Ctrl Pts',(-0.313797594204672,3.25924674056197,
-3.76132767947797));
#30382=CARTESIAN_POINT('Ctrl Pts',(-0.317605535936777,3.21832617575843,
-3.75544466935995));
#30383=CARTESIAN_POINT('Ctrl Pts',(-0.321881730426927,3.17739517904764,
-3.74888292969922));
#30384=CARTESIAN_POINT('Ctrl Pts',(-0.326689926501334,3.13608827366232,
-3.74155331642238));
#30385=CARTESIAN_POINT('Ctrl Pts',(-0.33141297166874,3.09551289428063,-3.73435350717368));
#30386=CARTESIAN_POINT('Ctrl Pts',(-0.336649342271546,3.05457452467595,
-3.72641276750167));
#30387=CARTESIAN_POINT('Ctrl Pts',(-0.342459459876233,3.0129385834656,-3.71759792427891));
#30388=CARTESIAN_POINT('Ctrl Pts',(-0.344418554584142,2.99889949551009,
-3.71462567588676));
#30389=CARTESIAN_POINT('Ctrl Pts',(-0.346442881404941,2.98478121679129,
-3.71155363126647));
#30390=CARTESIAN_POINT('Ctrl Pts',(-0.348534756685023,2.9705713231386,-3.70837539496744));
#30391=CARTESIAN_POINT('Ctrl Pts',(-0.356659453339846,2.91538109429238,
-3.69603134842088));
#30392=CARTESIAN_POINT('Ctrl Pts',(-0.365803112449362,2.85881925761048,
-3.68208281858365));
#30393=CARTESIAN_POINT('Ctrl Pts',(-0.37604091649859,2.80129090113052,-3.66641243395166));
#30394=CARTESIAN_POINT('Ctrl Pts',(-0.385983162284082,2.74542334818568,
-3.65119444239651));
#30395=CARTESIAN_POINT('Ctrl Pts',(-0.396957290506915,2.68864469579488,
-3.6343524254303));
#30396=CARTESIAN_POINT('Ctrl Pts',(-0.409032158424929,2.63132978639543,
-3.61582769664616));
#30397=CARTESIAN_POINT('Ctrl Pts',(-0.416588932442298,2.59546058922504,
-3.60423442787457));
#30398=CARTESIAN_POINT('Ctrl Pts',(-0.424576821049575,2.55938141989069,
-3.59198309575253));
#30399=CARTESIAN_POINT('Ctrl Pts',(-0.4330127018923,2.52318380344511,-3.57906976744169));
#30400=CARTESIAN_POINT('Ctrl Pts',(-0.433012750939953,2.52318359296197,
-3.57906969235237));
#30401=CARTESIAN_POINT('Ctrl Pts',(-0.448008301212658,2.45883169965399,
-3.55611221221238));
#30402=CARTESIAN_POINT('Ctrl Pts',(-0.47294675063507,2.33599978785211,-3.50837670153741));
#30403=CARTESIAN_POINT('Ctrl Pts',(-0.4951282325919,2.169475318356,-3.433897201164));
#30404=CARTESIAN_POINT('Ctrl Pts',(-0.5000030708506,2.069070757037,-3.383302730847));
#30405=CARTESIAN_POINT('Ctrl Pts',(-0.5000027938226,2.021563351426,-3.358143198296));
#30406=CARTESIAN_POINT('Origin',(0.,3.8,0.));
#30407=CARTESIAN_POINT('',(-0.2886751345948,3.79999999959147,3.8));
#30408=CARTESIAN_POINT('',(-0.433012748163509,5.07681640761144,3.57906969214753));
#30409=CARTESIAN_POINT('Ctrl Pts',(-0.2886751345948,3.800000000012,3.8));
#30410=CARTESIAN_POINT('Ctrl Pts',(-0.288675077512002,3.854680470407,3.79999999999983));
#30411=CARTESIAN_POINT('Ctrl Pts',(-0.289488192254766,3.90961078877838,
3.79881541653737));
#30412=CARTESIAN_POINT('Ctrl Pts',(-0.29106443631587,3.96445101878628,3.79643989316572));
#30413=CARTESIAN_POINT('Ctrl Pts',(-0.292644478808979,4.01942340274798,
3.79405864525926));
#30414=CARTESIAN_POINT('Ctrl Pts',(-0.294991333029181,4.07430489435071,
3.79048071962058));
#30415=CARTESIAN_POINT('Ctrl Pts',(-0.298054593819528,4.12875580671285,
3.78575218675927));
#30416=CARTESIAN_POINT('Ctrl Pts',(-0.299720336973532,4.15836518074405,
3.78318090021813));
#30417=CARTESIAN_POINT('Ctrl Pts',(-0.301597919992156,4.18784731408018,
3.78027029368594));
#30418=CARTESIAN_POINT('Ctrl Pts',(-0.303679237984622,4.21714850636058,
3.77703417030362));
#30419=CARTESIAN_POINT('Ctrl Pts',(-0.306623704527528,4.25860126881648,
3.77245598616143));
#30420=CARTESIAN_POINT('Ctrl Pts',(-0.309975928571019,4.29968660146913,
3.76723201769777));
#30421=CARTESIAN_POINT('Ctrl Pts',(-0.313800430565152,4.34078239401191,
3.76132349078443));
#30422=CARTESIAN_POINT('Ctrl Pts',(-0.31760959484575,4.38171337673252,3.75543865932041));
#30423=CARTESIAN_POINT('Ctrl Pts',(-0.321887256642832,4.4226550181757,3.74887471626853));
#30424=CARTESIAN_POINT('Ctrl Pts',(-0.326697163260439,4.46397267254489,
3.74154250144424));
#30425=CARTESIAN_POINT('Ctrl Pts',(-0.331421911964052,4.50455881057979,
3.73434010122323));
#30426=CARTESIAN_POINT('Ctrl Pts',(-0.336660225862619,4.54550804309632,
3.72639637912335));
#30427=CARTESIAN_POINT('Ctrl Pts',(-0.342472525973247,4.58715483660548,
3.71757814486913));
#30428=CARTESIAN_POINT('Ctrl Pts',(-0.344428109536364,4.60116715243447,
3.7146111965638));
#30429=CARTESIAN_POINT('Ctrl Pts',(-0.346448669875045,4.61525831485455,
3.71154483758887));
#30430=CARTESIAN_POINT('Ctrl Pts',(-0.348536508288431,4.62944066318899,
3.70837271404165));
#30431=CARTESIAN_POINT('Ctrl Pts',(-0.356662858901035,4.68464164729618,
3.69602607458624));
#30432=CARTESIAN_POINT('Ctrl Pts',(-0.365808436465691,4.74121366106227,
3.68207456931469));
#30433=CARTESIAN_POINT('Ctrl Pts',(-0.376048419508924,4.79875168152469,
3.66640083442217));
#30434=CARTESIAN_POINT('Ctrl Pts',(-0.385992977863913,4.85462972348075,
3.65117928858355));
#30435=CARTESIAN_POINT('Ctrl Pts',(-0.396969705155249,4.91141841694761,
3.63433329970587));
#30436=CARTESIAN_POINT('Ctrl Pts',(-0.409047459096639,4.96874295603494,
3.61580418478638));
#30437=CARTESIAN_POINT('Ctrl Pts',(-0.416599751629854,5.00458833677544,
3.60421781724382));
#30438=CARTESIAN_POINT('Ctrl Pts',(-0.424582554004133,5.04064317972623,
3.59197431995565));
#30439=CARTESIAN_POINT('Ctrl Pts',(-0.4330127018923,5.07681619655489,3.57906976744169));
#30440=CARTESIAN_POINT('',(-0.500001202747678,5.57843980229415,3.35814469502115));
#30441=CARTESIAN_POINT('Ctrl Pts',(-0.433012750939854,5.07681640703761,
3.57906969235253));
#30442=CARTESIAN_POINT('Ctrl Pts',(-0.448008301217003,5.14116830036308,
3.55611221220637));
#30443=CARTESIAN_POINT('Ctrl Pts',(-0.472946750665154,5.26399868565327,
3.50837750997614));
#30444=CARTESIAN_POINT('Ctrl Pts',(-0.495128010756759,5.4305283596975,3.43389511617736));
#30445=CARTESIAN_POINT('Ctrl Pts',(-0.500002924832392,5.53091478323016,
3.38331031137448));
#30446=CARTESIAN_POINT('Ctrl Pts',(-0.500002793997349,5.57842093152281,
3.35815152191705));
#30447=CARTESIAN_POINT('',(-0.5,3.76245328712248,3.7998145013082));
#30448=CARTESIAN_POINT('Origin',(-0.5,3.8,0.));
#30449=CARTESIAN_POINT('',(-0.500000724156204,2.02156681047555,3.35815048826256));
#30450=CARTESIAN_POINT('Origin',(-0.5,3.8,0.));
#30451=CARTESIAN_POINT('',(-0.4330127018922,2.523183803446,3.579069767442));
#30452=CARTESIAN_POINT('Ctrl Pts',(-0.5000021724646,2.021587730931,3.358161259977));
#30453=CARTESIAN_POINT('Ctrl Pts',(-0.5000045975033,2.07348246476,3.385642437576));
#30454=CARTESIAN_POINT('Ctrl Pts',(-0.4942244624564,2.180032313752,3.438990064545));
#30455=CARTESIAN_POINT('Ctrl Pts',(-0.4708077491425,2.347687391963,3.513147271656));
#30456=CARTESIAN_POINT('Ctrl Pts',(-0.4468343744848,2.463881670505,3.557914059235));
#30457=CARTESIAN_POINT('Ctrl Pts',(-0.4330127018922,2.523183803446,3.579069767442));
#30458=CARTESIAN_POINT('Ctrl Pts',(-0.4330127018922,2.523183803446,3.57906976744201));
#30459=CARTESIAN_POINT('Ctrl Pts',(-0.421461955081707,2.57274545228049,
3.59675065104351));
#30460=CARTESIAN_POINT('Ctrl Pts',(-0.410578361600438,2.62288617598632,
3.61347302244933));
#30461=CARTESIAN_POINT('Ctrl Pts',(-0.400384366707824,2.67327924047737,
3.62911839570725));
#30462=CARTESIAN_POINT('Ctrl Pts',(-0.390149610775323,2.72387380337345,
3.64482632752932));
#30463=CARTESIAN_POINT('Ctrl Pts',(-0.380609979224414,2.77472238881455,
3.65944851944638));
#30464=CARTESIAN_POINT('Ctrl Pts',(-0.371788187636978,2.82547947224395,
3.6729157002281));
#30465=CARTESIAN_POINT('Ctrl Pts',(-0.366141409425059,2.85796879031149,
3.68153596542712));
#30466=CARTESIAN_POINT('Ctrl Pts',(-0.360788745083571,2.89042033217581,
3.68968403564874));
#30467=CARTESIAN_POINT('Ctrl Pts',(-0.355736151997639,2.92274131878139,
3.69735272948451));
#30468=CARTESIAN_POINT('Ctrl Pts',(-0.349680482227613,2.96147889732692,
3.70654386691575));
#30469=CARTESIAN_POINT('Ctrl Pts',(-0.344055854981136,3.00002159271372,
3.71505018110053));
#30470=CARTESIAN_POINT('Ctrl Pts',(-0.338839256994681,3.03875870384398,
3.72297081495769));
#30471=CARTESIAN_POINT('Ctrl Pts',(-0.333642070583658,3.07735166962192,
3.7308619752035));
#30472=CARTESIAN_POINT('Ctrl Pts',(-0.328849882432668,3.11613787231206,
3.73817185829506));
#30473=CARTESIAN_POINT('Ctrl Pts',(-0.324439935228584,3.15551217709503,
3.74494798977599));
#30474=CARTESIAN_POINT('Ctrl Pts',(-0.320114937030083,3.19412801292544,
3.75159359234028));
#30475=CARTESIAN_POINT('Ctrl Pts',(-0.316157595366561,3.23330976389502,
3.75772587921199));
#30476=CARTESIAN_POINT('Ctrl Pts',(-0.312546442879592,3.27343563631605,
3.76334026775392));
#30477=CARTESIAN_POINT('Ctrl Pts',(-0.310836075108498,3.29244064904359,
3.76599943799144));
#30478=CARTESIAN_POINT('Ctrl Pts',(-0.309203367954887,3.31165751762995,
3.76854169759761));
#30479=CARTESIAN_POINT('Ctrl Pts',(-0.307646040500939,3.33112663667463,
3.77096244600287));
#30480=CARTESIAN_POINT('Ctrl Pts',(-0.303203848073521,3.38666124692601,
3.7778675000474));
#30481=CARTESIAN_POINT('Ctrl Pts',(-0.299374978655613,3.44423741493144,
3.78377682303441));
#30482=CARTESIAN_POINT('Ctrl Pts',(-0.296343776557985,3.50350417053243,
3.78841526539902));
#30483=CARTESIAN_POINT('Ctrl Pts',(-0.293416735114649,3.56073435323517,
3.79289431780017));
#30484=CARTESIAN_POINT('Ctrl Pts',(-0.29123348268165,3.61954059473043,3.79618800351884));
#30485=CARTESIAN_POINT('Ctrl Pts',(-0.289960005341534,3.67958500427146,
3.79809165618784));
#30486=CARTESIAN_POINT('Ctrl Pts',(-0.289119428723424,3.71921816076234,
3.79934818888941));
#30487=CARTESIAN_POINT('Ctrl Pts',(-0.288675227064339,3.75939032158238,
3.79999999999563));
#30488=CARTESIAN_POINT('Ctrl Pts',(-0.288675134594801,3.79999999959147,
3.8));
#30489=CARTESIAN_POINT('Ctrl Pts',(0.09332729536784,0.2663525855947,-2.027339375446));
#30490=CARTESIAN_POINT('Ctrl Pts',(0.0956460765109,0.2627254329722,-2.020940474449));
#30491=CARTESIAN_POINT('Ctrl Pts',(0.1067234777855,0.2452163007571,-1.98987166704));
#30492=CARTESIAN_POINT('Ctrl Pts',(0.1252614819808,0.2144240760922,-1.933661042191));
#30493=CARTESIAN_POINT('Ctrl Pts',(0.1483230597314,0.1738236541099,-1.855915420958));
#30494=CARTESIAN_POINT('Ctrl Pts',(0.1706856731413,0.1325495117081,-1.772637372698));
#30495=CARTESIAN_POINT('Ctrl Pts',(0.1930020158897,0.08995564733656,-1.681442257421));
#30496=CARTESIAN_POINT('Ctrl Pts',(0.2153249421398,0.04637396170794,-1.581617848906));
#30497=CARTESIAN_POINT('Ctrl Pts',(0.237760929357,0.002207589586509,-1.472368077024));
#30498=CARTESIAN_POINT('Ctrl Pts',(0.2604508155607,-0.04209002824358,-1.352628361368));
#30499=CARTESIAN_POINT('Ctrl Pts',(0.2834723960102,-0.08579256744141,-1.221593810851));
#30500=CARTESIAN_POINT('Ctrl Pts',(0.3069634986954,-0.1280921905644,-1.078167578903));
#30501=CARTESIAN_POINT('Ctrl Pts',(0.3311487111769,-0.1680644146237,-0.9208497005944));
#30502=CARTESIAN_POINT('Ctrl Pts',(0.3564829869058,-0.2046987259317,-0.7467239997496));
#30503=CARTESIAN_POINT('Ctrl Pts',(0.383183258108,-0.2361911499073,-0.5536747851934));
#30504=CARTESIAN_POINT('Ctrl Pts',(0.4118738384147,-0.2601195235891,-0.3402017808901));
#30505=CARTESIAN_POINT('Ctrl Pts',(0.4323948723823,-0.2689470860258,-0.1832271812612));
#30506=CARTESIAN_POINT('Ctrl Pts',(0.4433244432103,-0.2710639706472,-0.09819688475105));
#30507=CARTESIAN_POINT('Ctrl Pts',(0.4441525558925,-0.2712093650815,-0.09174594482558));
#30508=CARTESIAN_POINT('Ctrl Pts',(0.004133716395932,0.4140946903737,-1.91818759396));
#30509=CARTESIAN_POINT('Ctrl Pts',(0.006375610685108,0.4107521532303,-1.912236954105));
#30510=CARTESIAN_POINT('Ctrl Pts',(0.01709859516906,0.3946002443624,-1.883314369697));
#30511=CARTESIAN_POINT('Ctrl Pts',(0.03514371433922,0.3660649704597,-1.830747145249));
#30512=CARTESIAN_POINT('Ctrl Pts',(0.05770123147569,0.3282842837314,-1.757747888332));
#30513=CARTESIAN_POINT('Ctrl Pts',(0.0796798615306,0.2897221082235,-1.679243883391));
#30514=CARTESIAN_POINT('Ctrl Pts',(0.1016848560021,0.2498171933258,-1.593045679998));
#30515=CARTESIAN_POINT('Ctrl Pts',(0.123750946579,0.2089035319323,-1.498504779354));
#30516=CARTESIAN_POINT('Ctrl Pts',(0.1459810956979,0.1673646699477,-1.394842391727));
#30517=CARTESIAN_POINT('Ctrl Pts',(0.1685009069597,0.1256530218562,-1.281076556188));
#30518=CARTESIAN_POINT('Ctrl Pts',(0.1913848392552,0.08446552394875,-1.156432362992));
#30519=CARTESIAN_POINT('Ctrl Pts',(0.2147620673246,0.04458670410526,-1.019885111451));
#30520=CARTESIAN_POINT('Ctrl Pts',(0.2388605698404,0.006899880930569,-0.8699663883086));
#30521=CARTESIAN_POINT('Ctrl Pts',(0.2641204729043,-0.02760311364001,-0.7039575843831));
#30522=CARTESIAN_POINT('Ctrl Pts',(0.2907706259586,-0.05720484323787,-0.5197608497958));
#30523=CARTESIAN_POINT('Ctrl Pts',(0.3194378379588,-0.07956950255824,-0.3159115398517));
#30524=CARTESIAN_POINT('Ctrl Pts',(0.3399248718625,-0.08765027203072,-0.166143302502));
#30525=CARTESIAN_POINT('Ctrl Pts',(0.3508467599435,-0.08948791449151,-0.08495485013422));
#30526=CARTESIAN_POINT('Ctrl Pts',(0.3516743579076,-0.08961280997143,-0.07879497185162));
#30527=CARTESIAN_POINT('Ctrl Pts',(-0.1656119288838,0.4794541755272,-1.825386409491));
#30528=CARTESIAN_POINT('Ctrl Pts',(-0.1635163591258,0.4764802331255,-1.81996392764));
#30529=CARTESIAN_POINT('Ctrl Pts',(-0.1534678705812,0.4620697875466,-1.79353716736));
#30530=CARTESIAN_POINT('Ctrl Pts',(-0.1363607683355,0.4363025257814,-1.744942128327));
#30531=CARTESIAN_POINT('Ctrl Pts',(-0.1147625365557,0.401817534727,-1.676772747774));
#30532=CARTESIAN_POINT('Ctrl Pts',(-0.09351467101445,0.3662552687182,-1.602739197825));
#30533=CARTESIAN_POINT('Ctrl Pts',(-0.07210220814432,0.3291973603179,-1.520912659697));
#30534=CARTESIAN_POINT('Ctrl Pts',(-0.05052490541033,0.2910078739752,-1.430734790665));
#30535=CARTESIAN_POINT('Ctrl Pts',(-0.02868648988052,0.2520567001868,-1.331405236481));
#30536=CARTESIAN_POINT('Ctrl Pts',(-0.006490350805663,0.2128285287965,-1.222048142703));
#30537=CARTESIAN_POINT('Ctrl Pts',(0.01613162121186,0.1740090831683,-1.101895162335));
#30538=CARTESIAN_POINT('Ctrl Pts',(0.03929213278289,0.1363916820305,-0.9700014892297));
#30539=CARTESIAN_POINT('Ctrl Pts',(0.0632256162551,0.1008368490525,-0.8248557918097));
#30540=CARTESIAN_POINT('Ctrl Pts',(0.08834397957883,0.06837116739273,-0.6639649220209));
#30541=CARTESIAN_POINT('Ctrl Pts',(0.1148987520299,0.04065350496847,-0.4851100355562));
#30542=CARTESIAN_POINT('Ctrl Pts',(0.1435214914534,0.02000868274697,-0.2867927966161));
#30543=CARTESIAN_POINT('Ctrl Pts',(0.163943819323,0.01294768061339,-0.1413866086486));
#30544=CARTESIAN_POINT('Ctrl Pts',(0.1748512775237,0.01158181464608,-0.06242107600965));
#30545=CARTESIAN_POINT('Ctrl Pts',(0.1756779116267,0.01149231638014,-0.05642892400297));
#30546=CARTESIAN_POINT('Ctrl Pts',(-0.3607780994109,0.4412029905006,-1.779076638338));
#30547=CARTESIAN_POINT('Ctrl Pts',(-0.3588507672437,0.4385619065362,-1.774090671374));
#30548=CARTESIAN_POINT('Ctrl Pts',(-0.3495777848353,0.4257115558353,-1.749698719792));
#30549=CARTESIAN_POINT('Ctrl Pts',(-0.3335491737094,0.402324347319,-1.70411452853));
#30550=CARTESIAN_POINT('Ctrl Pts',(-0.3130538865687,0.370540606216,-1.639289845029));
#30551=CARTESIAN_POINT('Ctrl Pts',(-0.2926462223267,0.3372918543045,-1.567971206541));
#30552=CARTESIAN_POINT('Ctrl Pts',(-0.2719150265569,0.3023143326515,-1.488471217684));
#30553=CARTESIAN_POINT('Ctrl Pts',(-0.2508997108556,0.2660203897208,-1.400318838748));
#30554=CARTESIAN_POINT('Ctrl Pts',(-0.2295116935927,0.2287766291807,-1.302660309974));
#30555=CARTESIAN_POINT('Ctrl Pts',(-0.2076876987407,0.191122835208,-1.194714908186));
#30556=CARTESIAN_POINT('Ctrl Pts',(-0.1853669172732,0.1537553352,-1.07569529903));
#30557=CARTESIAN_POINT('Ctrl Pts',(-0.1624555769196,0.1175054839721,-0.9447183706796));
#30558=CARTESIAN_POINT('Ctrl Pts',(-0.1387118251765,0.08323678325404,-0.80016934265));
#30559=CARTESIAN_POINT('Ctrl Pts',(-0.1137561980987,0.05205271358332,-0.6397351948212));
#30560=CARTESIAN_POINT('Ctrl Pts',(-0.08731109012258,0.02560056658367,-0.4609765504096));
#30561=CARTESIAN_POINT('Ctrl Pts',(-0.05873948333614,0.006273119797196,
-0.2623030025696));
#30562=CARTESIAN_POINT('Ctrl Pts',(-0.03839155165444,0.0001736500266636,
-0.1169978048482));
#30563=CARTESIAN_POINT('Ctrl Pts',(-0.02750058379875,-0.0006811329928475,
-0.03791428735169));
#30564=CARTESIAN_POINT('Ctrl Pts',(-0.02667504964837,-0.0007318324155962,
-0.03191205058213));
#30565=CARTESIAN_POINT('',(0.0865744907536029,0.276461867453166,-1.99263825429456));
#30566=CARTESIAN_POINT('Ctrl Pts',(0.086572192368048,0.27646163366543,-1.99263802090364));
#30567=CARTESIAN_POINT('Ctrl Pts',(0.0865723894795379,0.276461279743604,
-1.99263643431398));
#30568=CARTESIAN_POINT('Ctrl Pts',(0.0865725865894618,0.276460925821444,
-1.99263484772351));
#30569=CARTESIAN_POINT('Ctrl Pts',(0.0865727836978197,0.27646057189895,
-1.99263326113225));
#30570=CARTESIAN_POINT('Ctrl Pts',(0.0891567115206156,0.271820940228061,
-1.97183435972548));
#30571=CARTESIAN_POINT('Ctrl Pts',(0.0914671231050367,0.267125712631713,
-1.95089962877548));
#30572=CARTESIAN_POINT('Ctrl Pts',(0.0935122293987559,0.262455035110272,
-1.93012905924239));
#30573=CARTESIAN_POINT('Ctrl Pts',(0.0941596821290163,0.260976362376874,
-1.92355338051383));
#30574=CARTESIAN_POINT('Ctrl Pts',(0.0947809196141619,0.259499997507271,
-1.91699407057979));
#30575=CARTESIAN_POINT('Ctrl Pts',(0.0953771352104668,0.258028107912017,
-1.91046048468356));
#30576=CARTESIAN_POINT('Ctrl Pts',(0.0955557312246131,0.257587204291573,
-1.90850335305805));
#30577=CARTESIAN_POINT('Ctrl Pts',(0.0957319805226283,0.257146849192486,
-1.9065485833918));
#30578=CARTESIAN_POINT('Ctrl Pts',(0.0959060097778447,0.256706880517564,
-1.90459553014602));
#30579=CARTESIAN_POINT('Ctrl Pts',(0.097493810682784,0.252692712558751,
-1.88677634389946));
#30580=CARTESIAN_POINT('Ctrl Pts',(0.0989008011237806,0.24870884944417,
-1.8690992935969));
#30581=CARTESIAN_POINT('Ctrl Pts',(0.10017829812544,0.244656350480217,-1.85110290858136));
#30582=CARTESIAN_POINT('Ctrl Pts',(0.100704848599869,0.242986017595427,
-1.84368527468036));
#30583=CARTESIAN_POINT('Ctrl Pts',(0.101208840073355,0.241304288351045,
-1.83621349856648));
#30584=CARTESIAN_POINT('Ctrl Pts',(0.101691640129157,0.239605341791607,
-1.82865576303145));
#30585=CARTESIAN_POINT('Ctrl Pts',(0.101946581634144,0.238708216806738,
-1.82466491744549));
#30586=CARTESIAN_POINT('Ctrl Pts',(0.102195936452327,0.237805832916687,
-1.8206499048855));
#30587=CARTESIAN_POINT('Ctrl Pts',(0.102439497850678,0.23689865123378,-1.81661186663138));
#30588=CARTESIAN_POINT('Ctrl Pts',(0.103898903583166,0.231462871354842,
-1.79241617627995));
#30589=CARTESIAN_POINT('Ctrl Pts',(0.105146699251486,0.225856178570456,
-1.76739479128144));
#30590=CARTESIAN_POINT('Ctrl Pts',(0.106164852738633,0.220154712920121,
-1.74175866230358));
#30591=CARTESIAN_POINT('Ctrl Pts',(0.106419458818648,0.218728967354355,
-1.73534792523084));
#30592=CARTESIAN_POINT('Ctrl Pts',(0.106659590009949,0.217297634713757,
-1.72889885721906));
#30593=CARTESIAN_POINT('Ctrl Pts',(0.106885499617317,0.21586057372366,-1.72240913586726));
#30594=CARTESIAN_POINT('Ctrl Pts',(0.107713756972225,0.21059184545503,-1.69861572794831));
#30595=CARTESIAN_POINT('Ctrl Pts',(0.108351090819835,0.20524572023201,-1.67427586744531));
#30596=CARTESIAN_POINT('Ctrl Pts',(0.108791121039501,0.199822429937497,
-1.64928232445734));
#30597=CARTESIAN_POINT('Ctrl Pts',(0.108951156646876,0.197850020958601,
-1.64019236505506));
#30598=CARTESIAN_POINT('Ctrl Pts',(0.109085136510625,0.195867422628958,
-1.63101618866698));
#30599=CARTESIAN_POINT('Ctrl Pts',(0.109193134880891,0.193875368857428,
-1.62175335534115));
#30600=CARTESIAN_POINT('Ctrl Pts',(0.109463080273659,0.188896166519022,
-1.59860060614561));
#30601=CARTESIAN_POINT('Ctrl Pts',(0.109570286280441,0.183857804617195,
-1.57490650509088));
#30602=CARTESIAN_POINT('Ctrl Pts',(0.10951482512735,0.178775962091305,-1.55067263118934));
#30603=CARTESIAN_POINT('Ctrl Pts',(0.109487072033164,0.176232977562583,
-1.53854585510594));
#30604=CARTESIAN_POINT('Ctrl Pts',(0.109418566296671,0.173679123371706,
-1.52628331173168));
#30605=CARTESIAN_POINT('Ctrl Pts',(0.109308883011478,0.171115928526719,
-1.51387842705374));
#30606=CARTESIAN_POINT('Ctrl Pts',(0.109111685863714,0.166507617317722,
-1.49157595979515));
#30607=CARTESIAN_POINT('Ctrl Pts',(0.10878136088443,0.161869001571485,-1.46881339834872));
#30608=CARTESIAN_POINT('Ctrl Pts',(0.108313218868863,0.157208146484988,
-1.44554692938918));
#30609=CARTESIAN_POINT('Ctrl Pts',(0.108001033258028,0.154100004417399,
-1.43003143071021));
#30610=CARTESIAN_POINT('Ctrl Pts',(0.107627386646029,0.150982306259349,
-1.41429254314733));
#30611=CARTESIAN_POINT('Ctrl Pts',(0.10719200013546,0.14785739335023,-1.39831770099805));
#30612=CARTESIAN_POINT('Ctrl Pts',(0.106611352561574,0.14368989377172,-1.37701305992163));
#30613=CARTESIAN_POINT('Ctrl Pts',(0.10592087243008,0.139509507623095,-1.35528876480802));
#30614=CARTESIAN_POINT('Ctrl Pts',(0.105117695700426,0.135324079865163,
-1.33311775486119));
#30615=CARTESIAN_POINT('Ctrl Pts',(0.104415231498044,0.131663474343298,
-1.31372682850179));
#30616=CARTESIAN_POINT('Ctrl Pts',(0.103626886060035,0.127998649213348,
-1.29399350119365));
#30617=CARTESIAN_POINT('Ctrl Pts',(0.102751909024411,0.124339054087829,
-1.27391565922516));
#30618=CARTESIAN_POINT('Ctrl Pts',(0.101876317049589,0.120676886976531,
-1.25382370642686));
#30619=CARTESIAN_POINT('Ctrl Pts',(0.100913986009255,0.117019958340212,
-1.2333867545795));
#30620=CARTESIAN_POINT('Ctrl Pts',(0.099864286261075,0.113377625644681,
-1.21260144449221));
#30621=CARTESIAN_POINT('Ctrl Pts',(0.0986644170002263,0.109214222684237,
-1.18884259850392));
#30622=CARTESIAN_POINT('Ctrl Pts',(0.0973503045944713,0.105070115399845,
-1.16462961242153));
#30623=CARTESIAN_POINT('Ctrl Pts',(0.0959208955659195,0.100960008497594,
-1.13995065515804));
#30624=CARTESIAN_POINT('Ctrl Pts',(0.0948501598641185,0.0978812269098513,
-1.12146424567172));
#30625=CARTESIAN_POINT('Ctrl Pts',(0.0937147709341765,0.0948215515490566,
-1.10271639655319));
#30626=CARTESIAN_POINT('Ctrl Pts',(0.0925141428635644,0.0917876969243179,
-1.08370349261096));
#30627=CARTESIAN_POINT('Ctrl Pts',(0.090711884050162,0.087233587812719,
-1.05516328558349));
#30628=CARTESIAN_POINT('Ctrl Pts',(0.0887624161433915,0.0827369922636152,
-1.02602400443288));
#30629=CARTESIAN_POINT('Ctrl Pts',(0.0866635512471383,0.078311623003293,
-0.996203974437649));
#30630=CARTESIAN_POINT('Ctrl Pts',(0.085497600329366,0.0758532640304192,
-0.979638500688956));
#30631=CARTESIAN_POINT('Ctrl Pts',(0.0842855705515153,0.0734169891445541,
-0.962862931509203));
#30632=CARTESIAN_POINT('Ctrl Pts',(0.0830271621620788,0.0710055491604767,
-0.945861979442115));
#30633=CARTESIAN_POINT('Ctrl Pts',(0.0805113794233251,0.0661846506839502,
-0.91187404507058));
#30634=CARTESIAN_POINT('Ctrl Pts',(0.0778094210554922,0.0614631819880825,
-0.876988620646972));
#30635=CARTESIAN_POINT('Ctrl Pts',(0.0749072538413882,0.0568696075407514,
-0.841041215753322));
#30636=CARTESIAN_POINT('Ctrl Pts',(0.0737445261640158,0.0550292324851632,
-0.826639205284582));
#30637=CARTESIAN_POINT('Ctrl Pts',(0.0725496940810796,0.0532095281332425,
-0.812066792693763));
#30638=CARTESIAN_POINT('Ctrl Pts',(0.071321326187919,0.0514129525452542,
-0.797314202957885));
#30639=CARTESIAN_POINT('Ctrl Pts',(0.0679485646593548,0.0464800484372401,
-0.756807635353096));
#30640=CARTESIAN_POINT('Ctrl Pts',(0.0643257157371699,0.0417180858650663,
-0.714939461591492));
#30641=CARTESIAN_POINT('Ctrl Pts',(0.0604397797041336,0.0371900436535931,
-0.671518074178239));
#30642=CARTESIAN_POINT('Ctrl Pts',(0.0593779426029125,0.0359527501996705,
-0.659653123301561));
#30643=CARTESIAN_POINT('Ctrl Pts',(0.058296514394975,0.0347330482780736,
-0.647672164086912));
#30644=CARTESIAN_POINT('Ctrl Pts',(0.0571958008445849,0.0335324230205638,
-0.635571162783657));
#30645=CARTESIAN_POINT('Ctrl Pts',(0.0528001609141237,0.0287377911006063,
-0.587246469671356));
#30646=CARTESIAN_POINT('Ctrl Pts',(0.0480918396870737,0.0242470394462572,
-0.537007861922811));
#30647=CARTESIAN_POINT('Ctrl Pts',(0.0430831220032363,0.0201948414791885,
-0.484762336726024));
#30648=CARTESIAN_POINT('Ctrl Pts',(0.0422475647486355,0.0195188514110342,
-0.476046707226787));
#30649=CARTESIAN_POINT('Ctrl Pts',(0.0414037495294555,0.0188551002544172,
-0.467275222038145));
#30650=CARTESIAN_POINT('Ctrl Pts',(0.0405515875419014,0.0182042309408489,
-0.45844730531979));
#30651=CARTESIAN_POINT('Ctrl Pts',(0.0358409313489692,0.0146062981445854,
-0.409647568688297));
#30652=CARTESIAN_POINT('Ctrl Pts',(0.0308772748861987,0.0114003528827624,
-0.359129169797274));
#30653=CARTESIAN_POINT('Ctrl Pts',(0.0256599441662973,0.00870164296594191,
-0.306772181437106));
#30654=CARTESIAN_POINT('Ctrl Pts',(0.0247474568793358,0.0082296509411883,
-0.297615183572278));
#30655=CARTESIAN_POINT('Ctrl Pts',(0.023827246648876,0.007773234547942,
-0.288402053146454));
#30656=CARTESIAN_POINT('Ctrl Pts',(0.0228993572944685,0.0073330928560306,
-0.279132302431854));
#30657=CARTESIAN_POINT('Ctrl Pts',(0.0224196995669689,0.00710556856909132,
-0.274340451397965));
#30658=CARTESIAN_POINT('Ctrl Pts',(0.0219379899997736,0.00688239373712214,
-0.269533471847087));
#30659=CARTESIAN_POINT('Ctrl Pts',(0.0214542272153199,0.00666366350834061,
-0.264711292193313));
#30660=CARTESIAN_POINT('Ctrl Pts',(0.0168726023431542,0.00459211131647106,
-0.219041350333829));
#30661=CARTESIAN_POINT('Ctrl Pts',(0.012107704008177,0.00291832101405385,
-0.171999057778165));
#30662=CARTESIAN_POINT('Ctrl Pts',(0.0071767230354041,0.00173218952277883,
-0.123647703296785));
#30663=CARTESIAN_POINT('Ctrl Pts',(0.00482106357237431,0.00116554327383814,
-0.100548987977606));
#30664=CARTESIAN_POINT('Ctrl Pts',(0.00242773055893293,0.000710192814652613,
-0.0771508945150003));
#30665=CARTESIAN_POINT('Ctrl Pts',(-4.41691394796437E-8,0.000376013360727031,
-0.0534561522398133));
#30666=CARTESIAN_POINT('Origin',(-0.3268616990873,-0.004510051500619,-2.00392196632));
#30667=CARTESIAN_POINT('Ctrl Pts',(0.001363716877125,0.5959039627023,-1.995067420053));
#30668=CARTESIAN_POINT('Ctrl Pts',(-0.0002547629821562,0.5664635602052,
-1.947200740707));
#30669=CARTESIAN_POINT('Ctrl Pts',(-0.004372367677236,0.4912734831306,-1.819803089527));
#30670=CARTESIAN_POINT('Ctrl Pts',(-0.010697518644,0.3716703089505,-1.590379225775));
#30671=CARTESIAN_POINT('Ctrl Pts',(-0.01714467798321,0.2420950677737,-1.288569665529));
#30672=CARTESIAN_POINT('Ctrl Pts',(-0.02256867464757,0.1250955634456,-0.9310228511924));
#30673=CARTESIAN_POINT('Ctrl Pts',(-0.02637651263401,0.03561097409294,-0.5171914444459));
#30674=CARTESIAN_POINT('Ctrl Pts',(-0.02742725699744,0.00614471551626,-0.2127089892193));
#30675=CARTESIAN_POINT('Ctrl Pts',(-0.0274982583504,0.0009348878949177,
-0.05030904096571));
#30676=CARTESIAN_POINT('Ctrl Pts',(-0.02750035356637,0.0007368753892566,
-0.0435739000559));
#30677=CARTESIAN_POINT('Ctrl Pts',(-0.02360189154764,0.2674772673847,-2.008012314209));
#30678=CARTESIAN_POINT('Ctrl Pts',(-0.007100235964077,0.2366788583949,-1.961090142431));
#30679=CARTESIAN_POINT('Ctrl Pts',(0.0350348100739,0.1618430617063,-1.831220908937));
#30680=CARTESIAN_POINT('Ctrl Pts',(0.1002819388271,0.05748454313784,-1.58377920092));
#30681=CARTESIAN_POINT('Ctrl Pts',(0.1674804264519,-0.03345159548168,-1.25031815927));
#30682=CARTESIAN_POINT('Ctrl Pts',(0.2248447651455,-0.08751112646634,-0.8568392396615));
#30683=CARTESIAN_POINT('Ctrl Pts',(0.2662490974893,-0.08993933952185,-0.4123496126141));
#30684=CARTESIAN_POINT('Ctrl Pts',(0.2789069387192,-0.04935013640268,-0.09830602538954));
#30685=CARTESIAN_POINT('Ctrl Pts',(0.280659326246,-0.01693316005029,0.06530116546309));
#30686=CARTESIAN_POINT('Ctrl Pts',(0.2807233254675,-0.01557036011737,0.07207992811515));
#30687=CARTESIAN_POINT('Ctrl Pts',(0.2095583867952,0.03476773911214,-2.019596510591));
#30688=CARTESIAN_POINT('Ctrl Pts',(0.2389857802896,0.01651651743335,-1.964918501646));
#30689=CARTESIAN_POINT('Ctrl Pts',(0.3101581568231,-0.02378135277356,-1.8140793846));
#30690=CARTESIAN_POINT('Ctrl Pts',(0.4068616564537,-0.06360695540912,-1.532524925838));
#30691=CARTESIAN_POINT('Ctrl Pts',(0.4886889080963,-0.07025856326138,-1.166376398116));
#30692=CARTESIAN_POINT('Ctrl Pts',(0.5374668975788,-0.0301895956346,-0.7523865517121));
#30693=CARTESIAN_POINT('Ctrl Pts',(0.5443422263587,0.06410224085544,-0.306016547345));
#30694=CARTESIAN_POINT('Ctrl Pts',(0.5164520353949,0.1626419470658,-0.005351407090899));
#30695=CARTESIAN_POINT('Ctrl Pts',(0.4928891039187,0.2211875903434,0.1483861234045));
#30696=CARTESIAN_POINT('Ctrl Pts',(0.4918968454427,0.2236257229715,0.1547511527327));
#30697=CARTESIAN_POINT('Ctrl Pts',(0.5381945238366,0.06011096769621,-2.021739002091));
#30698=CARTESIAN_POINT('Ctrl Pts',(0.5663364060878,0.05955934821613,-1.956015197361));
#30699=CARTESIAN_POINT('Ctrl Pts',(0.6290746726958,0.06388977555888,-1.780336254063));
#30700=CARTESIAN_POINT('Ctrl Pts',(0.6951750183963,0.09286790168404,-1.472370815216));
#30701=CARTESIAN_POINT('Ctrl Pts',(0.722409287336,0.1573502975438,-1.095301225048));
#30702=CARTESIAN_POINT('Ctrl Pts',(0.6972159851597,0.2570732908323,-0.6905298257101));
#30703=CARTESIAN_POINT('Ctrl Pts',(0.6139081869808,0.390278014667,-0.2723690173986));
#30704=CARTESIAN_POINT('Ctrl Pts',(0.5194992042508,0.4942376361727,0.001310753365298));
#30705=CARTESIAN_POINT('Ctrl Pts',(0.4611419320742,0.5491867406386,0.140986686312));
#30706=CARTESIAN_POINT('Ctrl Pts',(0.4587078974379,0.5514645860387,0.1467692430352));
#30707=CARTESIAN_POINT('',(0.517453073023301,0.0581490680041601,-2.00135351550452));
#30708=CARTESIAN_POINT('Origin',(0.5,0.5574505945004,-1.981381677743));
#30709=CARTESIAN_POINT('',(0.0174497466342749,0.000631384652492612,-0.0468912686246816));
#30710=CARTESIAN_POINT('Ctrl Pts',(0.5174542977566,0.05814216397504,-2.00131664892));
#30711=CARTESIAN_POINT('Ctrl Pts',(0.5174639416778,0.05475396251608,-1.917084695768));
#30712=CARTESIAN_POINT('Ctrl Pts',(0.5075557516816,0.04777984816496,-1.740184484562));
#30713=CARTESIAN_POINT('Ctrl Pts',(0.4629797196812,0.03689526489914,-1.449958596358));
#30714=CARTESIAN_POINT('Ctrl Pts',(0.3893196154359,0.02615576871374,-1.136163711401));
#30715=CARTESIAN_POINT('Ctrl Pts',(0.2880099327639,0.01602335717792,-0.7982355138282));
#30716=CARTESIAN_POINT('Ctrl Pts',(0.1627480055582,0.007130463259151,-0.4370888248374));
#30717=CARTESIAN_POINT('Ctrl Pts',(0.06701238076293,0.002487361406222,-0.1800461149003));
#30718=CARTESIAN_POINT('Ctrl Pts',(0.01744974438142,0.0006314603528128,
-0.04689126959127));
#30719=CARTESIAN_POINT('Origin',(-1.165507207395E-9,0.5003265405398,-0.04642263385298));
#30720=CARTESIAN_POINT('Ctrl Pts',(0.006092677297575,0.0006211886451104,
-0.06868317847516));
#30721=CARTESIAN_POINT('Ctrl Pts',(0.003734755652693,0.0005321863950901,
-0.06378738842989));
#30722=CARTESIAN_POINT('Ctrl Pts',(-0.0004662461385957,0.0003735846093764,
-0.0539892436276));
#30723=CARTESIAN_POINT('Ctrl Pts',(-0.005281917808373,0.000191741613253,
-0.03903695947574));
#30724=CARTESIAN_POINT('Ctrl Pts',(-0.008492810860386,7.047881929461E-5,
-0.02433820698463));
#30725=CARTESIAN_POINT('Ctrl Pts',(-0.01020745238675,5.717916985109E-6,
-0.009761485291432));
#30726=CARTESIAN_POINT('Ctrl Pts',(-0.01046402050289,-3.972854523874E-6,
0.005086971193826));
#30727=CARTESIAN_POINT('Ctrl Pts',(-0.009120895507617,4.675707571391E-5,
0.0206052220199));
#30728=CARTESIAN_POINT('Ctrl Pts',(-0.005888618210501,0.0001688308862598,
0.03701638652806));
#30729=CARTESIAN_POINT('Ctrl Pts',(-0.0007646346092876,0.000362319517914,
0.05329605733798));
#30730=CARTESIAN_POINT('Ctrl Pts',(0.003740802969237,0.000532414618925,
0.06380088841363));
#30731=CARTESIAN_POINT('Ctrl Pts',(0.006102566108989,0.0006215605327993,
0.06870005168943));
#30732=CARTESIAN_POINT('Ctrl Pts',(0.01191131197223,0.0005749797399242,
-0.0658677090212));
#30733=CARTESIAN_POINT('Ctrl Pts',(0.00963371057603,0.0004892299014565,
-0.06113683657842));
#30734=CARTESIAN_POINT('Ctrl Pts',(0.005585856909428,0.0003368091360034,
-0.05169022499205));
#30735=CARTESIAN_POINT('Ctrl Pts',(0.0009633490093534,0.0001627225989566,
-0.03732842304272));
#30736=CARTESIAN_POINT('Ctrl Pts',(-0.002109362176125,4.698878340268E-5,
-0.02325255344655));
#30737=CARTESIAN_POINT('Ctrl Pts',(-0.003746892799021,-1.469338550221E-5,
-0.009321455256237));
#30738=CARTESIAN_POINT('Ctrl Pts',(-0.003991703710451,-2.39151618659E-5,
0.004857311811217));
#30739=CARTESIAN_POINT('Ctrl Pts',(-0.002709569206432,2.438079570959E-5,
0.01968209560004));
#30740=CARTESIAN_POINT('Ctrl Pts',(0.0003816499484515,0.0001408144285733,
0.03538922245701));
#30741=CARTESIAN_POINT('Ctrl Pts',(0.005298322943173,0.000325982175415,
0.05102182560571));
#30742=CARTESIAN_POINT('Ctrl Pts',(0.009639551536444,0.0004894497837499,
0.06114990277001));
#30743=CARTESIAN_POINT('Ctrl Pts',(0.01192093360861,0.0005753410642185,
0.06588431050857));
#30744=CARTESIAN_POINT('Ctrl Pts',(0.01772876858441,0.0006541169916031,
-0.06305053973395));
#30745=CARTESIAN_POINT('Ctrl Pts',(0.01553153160975,0.0005716213667831,
-0.05848468665063));
#30746=CARTESIAN_POINT('Ctrl Pts',(0.01163691029307,0.0004253850445901,
-0.04938982358326));
#30747=CARTESIAN_POINT('Ctrl Pts',(0.007207672394919,0.0002590592591866,
-0.03561886171171));
#30748=CARTESIAN_POINT('Ctrl Pts',(0.004273219070382,0.0001488574804655,
-0.0221662498297));
#30749=CARTESIAN_POINT('Ctrl Pts',(0.002712841758818,9.02557475416E-5,-0.008881161993923));
#30750=CARTESIAN_POINT('Ctrl Pts',(0.002479794518074,8.150322565388E-5,
0.004627515065121));
#30751=CARTESIAN_POINT('Ctrl Pts',(0.003700904988553,0.0001273638646299,
0.01875841664537));
#30752=CARTESIAN_POINT('Ctrl Pts',(0.006650988424963,0.0002381542001466,
0.03376108270538));
#30753=CARTESIAN_POINT('Ctrl Pts',(0.01136023680079,0.0004149964575127,
0.04874622628719));
#30754=CARTESIAN_POINT('Ctrl Pts',(0.01553716610055,0.0005718329029132,
0.05849731878084));
#30755=CARTESIAN_POINT('Ctrl Pts',(0.01773812289881,0.000654467746636,0.06306686930469));
#30756=CARTESIAN_POINT('Ctrl Pts',(0.02354285942016,0.0008585706397761,
-0.06023273003868));
#30757=CARTESIAN_POINT('Ctrl Pts',(0.02142600081806,0.0007793298069184,
-0.05583193601455));
#30758=CARTESIAN_POINT('Ctrl Pts',(0.01768463845196,0.0006392790252621,
-0.04708890449065));
#30759=CARTESIAN_POINT('Ctrl Pts',(0.01344870410678,0.0004807153655589,
-0.0339089183807));
#30760=CARTESIAN_POINT('Ctrl Pts',(0.01065253264431,0.0003760466017198,
-0.02107970464963));
#30761=CARTESIAN_POINT('Ctrl Pts',(0.009169322037649,0.0003205258489241,
-0.008440771081267));
#30762=CARTESIAN_POINT('Ctrl Pts',(0.008948040509729,0.0003122426643748,
0.00439766737295));
#30763=CARTESIAN_POINT('Ctrl Pts',(0.01010811635309,0.0003556675546408,
0.01783453251478));
#30764=CARTESIAN_POINT('Ctrl Pts',(0.01291703957031,0.0004608135953648,
0.03213257955172));
#30765=CARTESIAN_POINT('Ctrl Pts',(0.01741882731899,0.0006293288894782,
0.04647011514478));
#30766=CARTESIAN_POINT('Ctrl Pts',(0.0214314288034,0.0007795329954019,0.05584413397741));
#30767=CARTESIAN_POINT('Ctrl Pts',(0.02355194636618,0.0008589108236551,
0.06024878760529));
#30768=CARTESIAN_POINT('',(0.01744974833007,0.0006313468236252,0.04689126965548));
#30769=CARTESIAN_POINT('Ctrl Pts',(0.0174497479592083,0.000631346809740766,
-0.0468912686588925));
#30770=CARTESIAN_POINT('Ctrl Pts',(0.0157883609881824,0.000569144385170808,
-0.042428263604913));
#30771=CARTESIAN_POINT('Ctrl Pts',(0.0143880925285003,0.000516716746237668,
-0.0380261499390857));
#30772=CARTESIAN_POINT('Ctrl Pts',(0.0132318096816563,0.000473426719980336,
-0.0337070287085344));
#30773=CARTESIAN_POINT('Ctrl Pts',(0.012075526745096,0.000430136690364122,
-0.0293879071428618));
#30774=CARTESIAN_POINT('Ctrl Pts',(0.0111632296390876,0.00039597912474571,
-0.0251517780112341));
#30775=CARTESIAN_POINT('Ctrl Pts',(0.0104662607830076,0.000369883996918147,
-0.0209620713811407));
#30776=CARTESIAN_POINT('Ctrl Pts',(0.00976929192692803,0.000343788869090604,
-0.0167723647510503));
#30777=CARTESIAN_POINT('Ctrl Pts',(0.00928765138909347,0.000325754222720897,
-0.0126290806302953));
#30778=CARTESIAN_POINT('Ctrl Pts',(0.00900722076971805,0.000315257154874697,
-0.00847390166297909));
#30779=CARTESIAN_POINT('Ctrl Pts',(0.00872679015034244,0.00030476008702849,
-0.00431872269566002));
#30780=CARTESIAN_POINT('Ctrl Pts',(0.00864756965543408,0.000301794698414069,
-0.000151648881534076));
#30781=CARTESIAN_POINT('Ctrl Pts',(0.00879065645835876,0.00030714892521388,
0.00415254495726168));
#30782=CARTESIAN_POINT('Ctrl Pts',(0.00893374326128334,0.000312503152013687,
0.00845673879605441));
#30783=CARTESIAN_POINT('Ctrl Pts',(0.00929913705597671,0.000326185758752549,
0.0128980526579098));
#30784=CARTESIAN_POINT('Ctrl Pts',(0.00993647955010509,0.000350048854730892,
0.017490916144555));
#30785=CARTESIAN_POINT('Ctrl Pts',(0.0105738220442339,0.000373911950709252,
0.0220837796312034));
#30786=CARTESIAN_POINT('Ctrl Pts',(0.0114831132114847,0.000407956289444159,
0.0268281927430151));
#30787=CARTESIAN_POINT('Ctrl Pts',(0.0127186536112733,0.000454214065906362,
0.0317313795019498));
#30788=CARTESIAN_POINT('Ctrl Pts',(0.013954194011061,0.000500471842368533,
0.0366345662608811));
#30789=CARTESIAN_POINT('Ctrl Pts',(0.0155159835211523,0.000558946556874616,
0.0416965266644137));
#30790=CARTESIAN_POINT('Ctrl Pts',(0.01744974833007,0.000631346823626039,
0.04689126965548));
#30791=CARTESIAN_POINT('Origin',(-3.054478024959E-10,0.500326540572,0.0464226361404));
#30792=CARTESIAN_POINT('Ctrl Pts',(-0.02750316139292,0.000737046107151,
0.04358922770264));
#30793=CARTESIAN_POINT('Ctrl Pts',(-0.02750089427334,0.0009349916310092,
0.0503203531369));
#30794=CARTESIAN_POINT('Ctrl Pts',(-0.02742485534677,0.006227555794608,
0.215269551417));
#30795=CARTESIAN_POINT('Ctrl Pts',(-0.02635280173773,0.03636739278822,0.5234275620995));
#30796=CARTESIAN_POINT('Ctrl Pts',(-0.02245453925619,0.1277268866354,0.9410069594231));
#30797=CARTESIAN_POINT('Ctrl Pts',(-0.01694441566883,0.2463169338229,1.299793310531));
#30798=CARTESIAN_POINT('Ctrl Pts',(-0.0104233500914,0.3770396234592,1.601669677065));
#30799=CARTESIAN_POINT('Ctrl Pts',(-0.004150342494761,0.4953591802118,1.82694866898));
#30800=CARTESIAN_POINT('Ctrl Pts',(-0.0001379825129479,0.5685899304984,
1.950653360374));
#30801=CARTESIAN_POINT('Ctrl Pts',(0.00136439425857,0.5959155261576,1.995080420042));
#30802=CARTESIAN_POINT('Ctrl Pts',(0.2807219033002,-0.01557494114624,-0.07206410546613));
#30803=CARTESIAN_POINT('Ctrl Pts',(0.2806561737658,-0.01693705404338,-0.06529447791634));
#30804=CARTESIAN_POINT('Ctrl Pts',(0.2788362287107,-0.04986605013889,0.1007651614235));
#30805=CARTESIAN_POINT('Ctrl Pts',(0.2659383333367,-0.09061371251157,0.418903610299));
#30806=CARTESIAN_POINT('Ctrl Pts',(0.2235950281925,-0.08686708797216,0.867690420062));
#30807=CARTESIAN_POINT('Ctrl Pts',(0.1653583372217,-0.03098330080804,1.262746140425));
#30808=CARTESIAN_POINT('Ctrl Pts',(0.09742648092702,0.06171309111801,1.596177405319));
#30809=CARTESIAN_POINT('Ctrl Pts',(0.0327510301912,0.1657560048726,1.838700874606));
#30810=CARTESIAN_POINT('Ctrl Pts',(-0.008292099066429,0.2388992121263,1.964475131896));
#30811=CARTESIAN_POINT('Ctrl Pts',(-0.02360837126204,0.26748382362,2.008025395665));
#30812=CARTESIAN_POINT('Ctrl Pts',(0.4918992607781,0.2236194238177,-0.154735914236));
#30813=CARTESIAN_POINT('Ctrl Pts',(0.4928878083092,0.2211824821229,-0.1483835574529));
#30814=CARTESIAN_POINT('Ctrl Pts',(0.5167500083103,0.1617115780388,0.007565532273837));
#30815=CARTESIAN_POINT('Ctrl Pts',(0.5448287089644,0.06217287105558,0.3123858450131));
#30816=CARTESIAN_POINT('Ctrl Pts',(0.5368240119861,-0.03202577563772,0.7634855185153));
#30817=CARTESIAN_POINT('Ctrl Pts',(0.4864905623783,-0.07085440170093,1.179726783911));
#30818=CARTESIAN_POINT('Ctrl Pts',(0.4030125096111,-0.06257200120437,1.546392400176));
#30819=CARTESIAN_POINT('Ctrl Pts',(0.3064646604076,-0.02184495218348,1.822739961703));
#30820=CARTESIAN_POINT('Ctrl Pts',(0.2368627668342,0.01782842154317,1.968863315844));
#30821=CARTESIAN_POINT('Ctrl Pts',(0.20954953649,0.0347661639898,2.019612509741));
#30822=CARTESIAN_POINT('Ctrl Pts',(0.4587131901114,0.5514599684041,-0.1467549726057));
#30823=CARTESIAN_POINT('Ctrl Pts',(0.4611428327526,0.5491832199421,-0.1409845745533));
#30824=CARTESIAN_POINT('Ctrl Pts',(0.5203496374827,0.4933654935977,0.0006860175196782));
#30825=CARTESIAN_POINT('Ctrl Pts',(0.6157665169565,0.3881443830302,0.2781802504261));
#30826=CARTESIAN_POINT('Ctrl Pts',(0.6987262516413,0.2539939406104,0.7010848027865));
#30827=CARTESIAN_POINT('Ctrl Pts',(0.7224328581585,0.1545174083523,1.108648913658));
#30828=CARTESIAN_POINT('Ctrl Pts',(0.6931602429224,0.09088468309498,1.487044303164));
#30829=CARTESIAN_POINT('Ctrl Pts',(0.6260499982531,0.06342531207403,1.790200141908));
#30830=CARTESIAN_POINT('Ctrl Pts',(0.5643084424037,0.05959486348343,1.96075674842));
#30831=CARTESIAN_POINT('Ctrl Pts',(0.5381889316308,0.06010461940414,2.021758679482));
#30832=CARTESIAN_POINT('',(0.0865743867590526,0.276459412161963,1.99264095059477));
#30833=CARTESIAN_POINT('Ctrl Pts',(-9.09801138851544E-7,0.000376077721329259,
0.0534607252662348));
#30834=CARTESIAN_POINT('Ctrl Pts',(0.00652835314144758,0.00127246330365846,
0.117157269627312));
#30835=CARTESIAN_POINT('Ctrl Pts',(0.0127944512297398,0.0030456007331035,
0.178629296439096));
#30836=CARTESIAN_POINT('Ctrl Pts',(0.0187482386330756,0.00549398588579434,
0.237760295451468));
#30837=CARTESIAN_POINT('Ctrl Pts',(0.0205286495875721,0.0062261470214498,
0.255442733748302));
#30838=CARTESIAN_POINT('Ctrl Pts',(0.0222814724261678,0.0070187559964705,
0.272915929701867));
#30839=CARTESIAN_POINT('Ctrl Pts',(0.0240062157849765,0.00786654683602309,
0.290177057805191));
#30840=CARTESIAN_POINT('Ctrl Pts',(0.0299524099712426,0.0107893752879032,
0.349686212632305));
#30841=CARTESIAN_POINT('Ctrl Pts',(0.0355590334273618,0.0143650914300685,
0.406673541011523));
#30842=CARTESIAN_POINT('Ctrl Pts',(0.040830769447185,0.0184196009791735,
0.461351968844045));
#30843=CARTESIAN_POINT('Ctrl Pts',(0.0422015721807883,0.0194738898799141,
0.475569930073535));
#30844=CARTESIAN_POINT('Ctrl Pts',(0.0435499058409064,0.0205607528992102,
0.489631863372403));
#30845=CARTESIAN_POINT('Ctrl Pts',(0.0448761834508286,0.0216775220448886,
0.50354169221264));
#30846=CARTESIAN_POINT('Ctrl Pts',(0.0450702352677852,0.0218409200244811,
0.505576882688457));
#30847=CARTESIAN_POINT('Ctrl Pts',(0.0452638122696533,0.0220049588166182,
0.507608814414488));
#30848=CARTESIAN_POINT('Ctrl Pts',(0.0454569139116692,0.0221696311704481,
0.509637503452834));
#30849=CARTESIAN_POINT('Ctrl Pts',(0.0504911582929488,0.0264627115573665,
0.562526315200067));
#30850=CARTESIAN_POINT('Ctrl Pts',(0.0552009765120379,0.0311819748374701,
0.613211073235368));
#30851=CARTESIAN_POINT('Ctrl Pts',(0.059585318651173,0.0362023190716366,
0.661979072375273));
#30852=CARTESIAN_POINT('Ctrl Pts',(0.0606025057087322,0.0373670614702519,
0.673293467094923));
#30853=CARTESIAN_POINT('Ctrl Pts',(0.0616022346451153,0.0385482249859112,
0.684504695746438));
#30854=CARTESIAN_POINT('Ctrl Pts',(0.0625845886509375,0.039744617250358,
0.695616355729162));
#30855=CARTESIAN_POINT('Ctrl Pts',(0.067314054123752,0.0455045529488005,
0.749112561702244));
#30856=CARTESIAN_POINT('Ctrl Pts',(0.0716395927107308,0.0516133879646876,
0.800300379856481));
#30857=CARTESIAN_POINT('Ctrl Pts',(0.0755946966027367,0.0579677961016361,
0.849588598140686));
#30858=CARTESIAN_POINT('Ctrl Pts',(0.076137857342939,0.0588404571293751,
0.856357427950849));
#30859=CARTESIAN_POINT('Ctrl Pts',(0.0766740369127634,0.0597178291689939,
0.863090434392253));
#30860=CARTESIAN_POINT('Ctrl Pts',(0.0772033241577391,0.0605997177594687,
0.869788678677261));
#30861=CARTESIAN_POINT('Ctrl Pts',(0.0785440273149263,0.062833572492906,
0.886755566403666));
#30862=CARTESIAN_POINT('Ctrl Pts',(0.079840730238549,0.0650962458724791,
0.903499201468074));
#30863=CARTESIAN_POINT('Ctrl Pts',(0.0810937204906553,0.0673839988051382,
0.920028260063856));
#30864=CARTESIAN_POINT('Ctrl Pts',(0.083937326066278,0.0725759522014398,
0.95754022243048));
#30865=CARTESIAN_POINT('Ctrl Pts',(0.0865557106728475,0.077896178421874,
0.993947062286089));
#30866=CARTESIAN_POINT('Ctrl Pts',(0.0889539161279948,0.0833020208043715,
1.02934740992229));
#30867=CARTESIAN_POINT('Ctrl Pts',(0.0924088532493085,0.091089862950746,
1.08034636620153));
#30868=CARTESIAN_POINT('Ctrl Pts',(0.0954064872304019,0.0990548371110723,
1.12925696354537));
#30869=CARTESIAN_POINT('Ctrl Pts',(0.097957198115787,0.107078805606651,
1.17620683708701));
#30870=CARTESIAN_POINT('Ctrl Pts',(0.0999421648726084,0.113323069044253,
1.21274329394345));
#30871=CARTESIAN_POINT('Ctrl Pts',(0.101656839723861,0.11960376445875,1.24809198876482));
#30872=CARTESIAN_POINT('Ctrl Pts',(0.103114408059529,0.125879416749678,
1.28234280769469));
#30873=CARTESIAN_POINT('Ctrl Pts',(0.103529836038383,0.127668068083146,
1.2921047846353));
#30874=CARTESIAN_POINT('Ctrl Pts',(0.103924381198634,0.12945636796932,1.30177759316701));
#30875=CARTESIAN_POINT('Ctrl Pts',(0.104298386010344,0.131243356550118,
1.31136316830229));
#30876=CARTESIAN_POINT('Ctrl Pts',(0.105984622059922,0.139300163496924,
1.35458063995765));
#30877=CARTESIAN_POINT('Ctrl Pts',(0.107252382666339,0.147329259312068,
1.39602675468255));
#30878=CARTESIAN_POINT('Ctrl Pts',(0.108116417619743,0.155318344975294,
1.43608914702022));
#30879=CARTESIAN_POINT('Ctrl Pts',(0.108980452573148,0.163307430638519,
1.47615153935789));
#30880=CARTESIAN_POINT('Ctrl Pts',(0.109440821161486,0.171256644751982,
1.51483017857233));
#30881=CARTESIAN_POINT('Ctrl Pts',(0.109518134026559,0.179029875568212,
1.55188588983053));
#30882=CARTESIAN_POINT('Ctrl Pts',(0.10954937952823,0.182171377260427,1.56686171936345));
#30883=CARTESIAN_POINT('Ctrl Pts',(0.109517733598986,0.1852845885706,1.58157153761736));
#30884=CARTESIAN_POINT('Ctrl Pts',(0.109424701710558,0.188373020356353,
1.59605530105348));
#30885=CARTESIAN_POINT('Ctrl Pts',(0.109287538484396,0.192926504915998,
1.61740969634115));
#30886=CARTESIAN_POINT('Ctrl Pts',(0.10901734790502,0.197425875042288,1.63827290332916));
#30887=CARTESIAN_POINT('Ctrl Pts',(0.108614123231663,0.201885013497263,
1.65876475480962));
#30888=CARTESIAN_POINT('Ctrl Pts',(0.108197298559382,0.206494550184769,
1.67994775734428));
#30889=CARTESIAN_POINT('Ctrl Pts',(0.107636013113304,0.211064909866213,
1.7007318090833));
#30890=CARTESIAN_POINT('Ctrl Pts',(0.106916313695468,0.21567514026169,1.72156283502369));
#30891=CARTESIAN_POINT('Ctrl Pts',(0.106467581648172,0.218549615455923,
1.73455096407572));
#30892=CARTESIAN_POINT('Ctrl Pts',(0.105956508353049,0.221439865662645,
1.74755699928328));
#30893=CARTESIAN_POINT('Ctrl Pts',(0.105370932926517,0.224367934091294,
1.76068425372678));
#30894=CARTESIAN_POINT('Ctrl Pts',(0.104614139175432,0.228152150076371,
1.7776498292643));
#30895=CARTESIAN_POINT('Ctrl Pts',(0.103730622287019,0.232003387630288,
1.7948137637274));
#30896=CARTESIAN_POINT('Ctrl Pts',(0.102682811222916,0.235980870867143,
1.81251182586718));
#30897=CARTESIAN_POINT('Ctrl Pts',(0.101740077804292,0.239559480120153,
1.82843507309721));
#30898=CARTESIAN_POINT('Ctrl Pts',(0.100664403176851,0.243240281303386,
1.84479084066647));
#30899=CARTESIAN_POINT('Ctrl Pts',(0.0993976726189429,0.247073344449856,
1.86180605447616));
#30900=CARTESIAN_POINT('Ctrl Pts',(0.0992357132674213,0.247563425325909,
1.86398155500184));
#30901=CARTESIAN_POINT('Ctrl Pts',(0.0990705841490034,0.248056005652083,
1.86616780777675));
#30902=CARTESIAN_POINT('Ctrl Pts',(0.0989021290735271,0.24855119856692,
1.86836524213669));
#30903=CARTESIAN_POINT('Ctrl Pts',(0.0971030164000728,0.253839895546632,
1.8918340037331));
#30904=CARTESIAN_POINT('Ctrl Pts',(0.0949363222751762,0.259415398134344,
1.91658901567945));
#30905=CARTESIAN_POINT('Ctrl Pts',(0.0922869113983242,0.265180778941099,
1.94227889863466));
#30906=CARTESIAN_POINT('Ctrl Pts',(0.0905915320651791,0.268870092498646,
1.95871806139862));
#30907=CARTESIAN_POINT('Ctrl Pts',(0.0886979474295743,0.272637052898358,
1.97553922388023));
#30908=CARTESIAN_POINT('Ctrl Pts',(0.0865694808505399,0.276456078074887,
1.99264108439717));
#30909=CARTESIAN_POINT('',(0.517453499953991,0.0581482537155648,2.00134959555289));
#30910=CARTESIAN_POINT('Ctrl Pts',(0.01744974833007,0.0006313468236252,
0.04689126965548));
#30911=CARTESIAN_POINT('Ctrl Pts',(0.06753743330703,0.002506810781753,0.1814388238611));
#30912=CARTESIAN_POINT('Ctrl Pts',(0.1639979857046,0.007200545681001,0.4404924524998));
#30913=CARTESIAN_POINT('Ctrl Pts',(0.2891401437734,0.0161206324859,0.8017214821276));
#30914=CARTESIAN_POINT('Ctrl Pts',(0.3899548010611,0.02623514120806,1.138584886082));
#30915=CARTESIAN_POINT('Ctrl Pts',(0.4632860851713,0.03695536152136,1.451600247463));
#30916=CARTESIAN_POINT('Ctrl Pts',(0.5076215437038,0.04781101990821,1.74099111528));
#30917=CARTESIAN_POINT('Ctrl Pts',(0.5174627880836,0.05476666475408,1.917359950681));
#30918=CARTESIAN_POINT('Ctrl Pts',(0.5174549507661,0.05813997872694,2.001305923414));
#30919=CARTESIAN_POINT('Origin',(0.5,0.5574505945004,1.981381677743));
#30920=CARTESIAN_POINT('Ctrl Pts',(0.4441505898026,-0.2712136506453,0.09177744215382));
#30921=CARTESIAN_POINT('Ctrl Pts',(0.4433243095181,-0.2710682902751,0.0982149450773));
#30922=CARTESIAN_POINT('Ctrl Pts',(0.4319126563181,-0.2688550636628,0.1870059243145));
#30923=CARTESIAN_POINT('Ctrl Pts',(0.4105084687887,-0.2594278398504,0.3505980872243));
#30924=CARTESIAN_POINT('Ctrl Pts',(0.3806737777615,-0.2337260742433,0.5722228281209));
#30925=CARTESIAN_POINT('Ctrl Pts',(0.353019478122,-0.2001401451587,0.7712432567423));
#30926=CARTESIAN_POINT('Ctrl Pts',(0.3268098245248,-0.1612906812422,0.949891806445));
#30927=CARTESIAN_POINT('Ctrl Pts',(0.301767398999,-0.1190354334272,1.110873752657));
#30928=CARTESIAN_POINT('Ctrl Pts',(0.2775004469511,-0.07465283465729,1.256626058425));
#30929=CARTESIAN_POINT('Ctrl Pts',(0.2538473285855,-0.02929051310002,1.388548718725));
#30930=CARTESIAN_POINT('Ctrl Pts',(0.2306285320361,0.01624208910001,1.508164313338));
#30931=CARTESIAN_POINT('Ctrl Pts',(0.207745940936,0.06125122341503,1.61657011171));
#30932=CARTESIAN_POINT('Ctrl Pts',(0.1848495979175,0.1056635488392,1.715813080168));
#30933=CARTESIAN_POINT('Ctrl Pts',(0.1609461047857,0.1507778699002,1.810174952061));
#30934=CARTESIAN_POINT('Ctrl Pts',(0.1337042946383,0.2000534730528,1.907032302569));
#30935=CARTESIAN_POINT('Ctrl Pts',(0.1104061460155,0.2393905012997,1.979544729913));
#30936=CARTESIAN_POINT('Ctrl Pts',(0.09567837415139,0.2626728328007,2.020855911046));
#30937=CARTESIAN_POINT('Ctrl Pts',(0.09337813193119,0.2662727193221,2.027206328594));
#30938=CARTESIAN_POINT('Ctrl Pts',(0.3516735936865,-0.08961443345137,0.07882304454895));
#30939=CARTESIAN_POINT('Ctrl Pts',(0.350847645443,-0.08948955446609,0.08497125195283));
#30940=CARTESIAN_POINT('Ctrl Pts',(0.3394417549389,-0.08756810521069,0.1697648837853));
#30941=CARTESIAN_POINT('Ctrl Pts',(0.3180756196171,-0.0789298656086,0.3258309287581));
#30942=CARTESIAN_POINT('Ctrl Pts',(0.2882640593895,-0.05489063086291,0.5374733705197));
#30943=CARTESIAN_POINT('Ctrl Pts',(0.2606668037211,-0.02331128782057,0.727339125934));
#30944=CARTESIAN_POINT('Ctrl Pts',(0.2345362971097,0.01328668833229,0.8976506379832));
#30945=CARTESIAN_POINT('Ctrl Pts',(0.2095892877488,0.05312819491485,1.051034607763));
#30946=CARTESIAN_POINT('Ctrl Pts',(0.1854463195438,0.09496901379647,1.18976893841));
#30947=CARTESIAN_POINT('Ctrl Pts',(0.1619437477539,0.1377124771179,1.315220328414));
#30948=CARTESIAN_POINT('Ctrl Pts',(0.138910375473,0.180572989123,1.428824558866));
#30949=CARTESIAN_POINT('Ctrl Pts',(0.116252767292,0.222883140253,1.531631702806));
#30950=CARTESIAN_POINT('Ctrl Pts',(0.09364048231002,0.2645458762256,1.625553474633));
#30951=CARTESIAN_POINT('Ctrl Pts',(0.07009425725316,0.3067759181797,1.714671038853));
#30952=CARTESIAN_POINT('Ctrl Pts',(0.04337896997847,0.3527292312924,1.805808681844));
#30953=CARTESIAN_POINT('Ctrl Pts',(0.02066764874299,0.3892243623864,1.87369224103));
#30954=CARTESIAN_POINT('Ctrl Pts',(0.006407516092703,0.4107061153768,1.912158009393));
#30955=CARTESIAN_POINT('Ctrl Pts',(0.004182600943537,0.4140246350262,1.918065761637));
#30956=CARTESIAN_POINT('Ctrl Pts',(0.1756764843761,0.01149244822416,0.05645169963164));
#30957=CARTESIAN_POINT('Ctrl Pts',(0.17485115759,0.01158197569545,0.06243513417433));
#30958=CARTESIAN_POINT('Ctrl Pts',(0.1634561005124,0.01301067790449,0.1449398854909));
#30959=CARTESIAN_POINT('Ctrl Pts',(0.142162384109,0.0205792288548,0.2964239473772));
#30960=CARTESIAN_POINT('Ctrl Pts',(0.1123948451772,0.04280987956687,0.5023434273092));
#30961=CARTESIAN_POINT('Ctrl Pts',(0.08490615253173,0.07240212532535,0.6866379321782));
#30962=CARTESIAN_POINT('Ctrl Pts',(0.05892627421398,0.1068593421783,0.851677617466));
#30963=CARTESIAN_POINT('Ctrl Pts',(0.03416085577481,0.1444520696214,1.000117458598));
#30964=CARTESIAN_POINT('Ctrl Pts',(0.01025384696266,0.1839161130489,1.134060645629));
#30965=CARTESIAN_POINT('Ctrl Pts',(-0.01296221266782,0.2241827829663,1.254905212894));
#30966=CARTESIAN_POINT('Ctrl Pts',(-0.03564269543703,0.2644587861952,1.364006309255));
#30967=CARTESIAN_POINT('Ctrl Pts',(-0.05787212820653,0.3040834971127,1.462390721409));
#30968=CARTESIAN_POINT('Ctrl Pts',(-0.07994380918533,0.3429004915365,1.551819675945));
#30969=CARTESIAN_POINT('Ctrl Pts',(-0.1028101008249,0.3820329385455,1.636246280064));
#30970=CARTESIAN_POINT('Ctrl Pts',(-0.128523338039,0.4242129766637,1.721805374643));
#30971=CARTESIAN_POINT('Ctrl Pts',(-0.1501178408998,0.4572657293956,1.78472613206));
#30972=CARTESIAN_POINT('Ctrl Pts',(-0.1634879877075,0.4764412198706,1.819892205208));
#30973=CARTESIAN_POINT('Ctrl Pts',(-0.1655695444196,0.47939642768,1.825280786222));
#30974=CARTESIAN_POINT('Ctrl Pts',(-0.02667784573403,-0.0007319642824258,
0.03192949709643));
#30975=CARTESIAN_POINT('Ctrl Pts',(-0.02750246349207,-0.0006811764769736,
0.03792619875474));
#30976=CARTESIAN_POINT('Ctrl Pts',(-0.03888513505006,0.0002138505247069,
0.1205939522374));
#30977=CARTESIAN_POINT('Ctrl Pts',(-0.06009558709032,0.006779437368235,
0.2719283687744));
#30978=CARTESIAN_POINT('Ctrl Pts',(-0.08981251210483,0.02764286901391,0.4782430106847));
#30979=CARTESIAN_POINT('Ctrl Pts',(-0.1171763833478,0.05591290450752,0.6623591991827));
#30980=CARTESIAN_POINT('Ctrl Pts',(-0.1429830753047,0.08903539736197,0.8269045289161));
#30981=CARTESIAN_POINT('Ctrl Pts',(-0.1675397077971,0.1252746988455,0.9746599149559));
#30982=CARTESIAN_POINT('Ctrl Pts',(-0.1911754199786,0.1632989348384,1.107594926954));
#30983=CARTESIAN_POINT('Ctrl Pts',(-0.2140620594383,0.2020353250487,1.227193389706));
#30984=CARTESIAN_POINT('Ctrl Pts',(-0.2363368040236,0.240653835145,1.334762175212));
#30985=CARTESIAN_POINT('Ctrl Pts',(-0.2580739379061,0.2784788650227,1.431336257167));
#30986=CARTESIAN_POINT('Ctrl Pts',(-0.2795240541198,0.3152782469921,1.518560016079));
#30987=CARTESIAN_POINT('Ctrl Pts',(-0.3016085856314,0.3521058650065,1.600372605688));
#30988=CARTESIAN_POINT('Ctrl Pts',(-0.3261697059412,0.3912871821253,1.682306192781));
#30989=CARTESIAN_POINT('Ctrl Pts',(-0.346480135901,0.4214151408305,1.741542105517));
#30990=CARTESIAN_POINT('Ctrl Pts',(-0.3588270127402,0.4385277461565,1.774025923849));
#30991=CARTESIAN_POINT('Ctrl Pts',(-0.3607437416807,0.4411556988437,1.778987451663));
#30992=CARTESIAN_POINT('Origin',(-0.3268607615544,-0.004512844089665,2.00391666631));
#30993=CARTESIAN_POINT('Ctrl Pts',(0.1027377857463,0.2516014974679,1.993772793209));
#30994=CARTESIAN_POINT('Ctrl Pts',(0.1018795142078,0.2529091607515,1.99856950602));
#30995=CARTESIAN_POINT('Ctrl Pts',(0.08748606425778,0.2750262500263,2.079318045689));
#30996=CARTESIAN_POINT('Ctrl Pts',(0.06218815931651,0.3199344673338,2.231178832349));
#30997=CARTESIAN_POINT('Ctrl Pts',(0.03182029544458,0.3937152656143,2.449036815776));
#30998=CARTESIAN_POINT('Ctrl Pts',(0.008692153136202,0.4786543405831,2.669750211539));
#30999=CARTESIAN_POINT('Ctrl Pts',(0.0003099300768639,0.5454908414197,2.821709674268));
#31000=CARTESIAN_POINT('Ctrl Pts',(-0.001018477605139,0.5836010689834,2.902151700762));
#31001=CARTESIAN_POINT('Ctrl Pts',(-0.001081418569355,0.5856932619884,2.906550131397));
#31002=CARTESIAN_POINT('Ctrl Pts',(-0.03993386604451,0.4842012940407,1.82477577565));
#31003=CARTESIAN_POINT('Ctrl Pts',(-0.04008326187016,0.4858259304199,1.82941037646));
#31004=CARTESIAN_POINT('Ctrl Pts',(-0.04249896901661,0.5132255431577,1.907411774626));
#31005=CARTESIAN_POINT('Ctrl Pts',(-0.04384834652328,0.5663417760107,2.053551607732));
#31006=CARTESIAN_POINT('Ctrl Pts',(-0.03627411384636,0.6462729463744,2.261605825127));
#31007=CARTESIAN_POINT('Ctrl Pts',(-0.01768977584964,0.730324119387,2.4705330558));
#31008=CARTESIAN_POINT('Ctrl Pts',(0.004566050698213,0.7897246608292,2.612726145468));
#31009=CARTESIAN_POINT('Ctrl Pts',(0.01963083731976,0.8212324290105,2.687391402537));
#31010=CARTESIAN_POINT('Ctrl Pts',(0.02046458526668,0.8229554088081,2.691471916486));
#31011=CARTESIAN_POINT('Ctrl Pts',(-0.3385562814283,0.5122548782035,1.710515139935));
#31012=CARTESIAN_POINT('Ctrl Pts',(-0.3385854937958,0.5146556694714,1.715026264093));
#31013=CARTESIAN_POINT('Ctrl Pts',(-0.3389179244204,0.5551248461428,1.790931560508));
#31014=CARTESIAN_POINT('Ctrl Pts',(-0.3344184843396,0.6329249209683,1.932588547284));
#31015=CARTESIAN_POINT('Ctrl Pts',(-0.312917850693,0.748065379891,2.13267148346));
#31016=CARTESIAN_POINT('Ctrl Pts',(-0.2740805475893,0.8668470835516,2.331716051354));
#31017=CARTESIAN_POINT('Ctrl Pts',(-0.2328066607506,0.9486868685298,2.465517500439));
#31018=CARTESIAN_POINT('Ctrl Pts',(-0.2060460780354,0.9912774222627,2.535169689394));
#31019=CARTESIAN_POINT('Ctrl Pts',(-0.2045679022214,0.993603941535,2.538974208362));
#31020=CARTESIAN_POINT('Ctrl Pts',(-0.592664250327,0.3169298805394,1.727694044175));
#31021=CARTESIAN_POINT('Ctrl Pts',(-0.5932426506397,0.3200449757575,1.732203216897));
#31022=CARTESIAN_POINT('Ctrl Pts',(-0.602784774432,0.3725971593248,1.808070564298));
#31023=CARTESIAN_POINT('Ctrl Pts',(-0.6144625375171,0.4749866408694,1.949492146447));
#31024=CARTESIAN_POINT('Ctrl Pts',(-0.612399990641,0.6307593114652,2.148787406837));
#31025=CARTESIAN_POINT('Ctrl Pts',(-0.5883650519268,0.7965753751741,2.34648704521));
#31026=CARTESIAN_POINT('Ctrl Pts',(-0.5524599168806,0.9156661437381,2.478904894027));
#31027=CARTESIAN_POINT('Ctrl Pts',(-0.5265523235192,0.9795848546602,2.547672988512));
#31028=CARTESIAN_POINT('Ctrl Pts',(-0.5251145852718,0.983082510075,2.551428709617));
#31029=CARTESIAN_POINT('Ctrl Pts',(0.0865773249525696,0.276461408980929,
1.99264087060027));
#31030=CARTESIAN_POINT('Ctrl Pts',(0.0865771947823855,0.27646163218119,
1.9926416609711));
#31031=CARTESIAN_POINT('Ctrl Pts',(0.0865770646123325,0.276461855381553,
1.99264245134172));
#31032=CARTESIAN_POINT('Ctrl Pts',(0.0865769344424107,0.276462078582019,
1.99264324171212));
#31033=CARTESIAN_POINT('Ctrl Pts',(0.078420000105942,0.290448654910433,
2.04217080843749));
#31034=CARTESIAN_POINT('Ctrl Pts',(0.0707810911918314,0.304841755020766,
2.0908545533155));
#31035=CARTESIAN_POINT('Ctrl Pts',(0.0637332814206178,0.319485185859224,
2.13835021057908));
#31036=CARTESIAN_POINT('Ctrl Pts',(0.0597136280289845,0.327836931769758,
2.16543892125728));
#31037=CARTESIAN_POINT('Ctrl Pts',(0.0558856017111063,0.336269535007341,
2.1921414988295));
#31038=CARTESIAN_POINT('Ctrl Pts',(0.0522572081993674,0.344749730813805,
2.21839710659208));
#31039=CARTESIAN_POINT('Ctrl Pts',(0.0471928269709879,0.356586083270145,
2.25504374005737));
#31040=CARTESIAN_POINT('Ctrl Pts',(0.0425107423664863,0.368518464963908,
2.29081396288276));
#31041=CARTESIAN_POINT('Ctrl Pts',(0.0381540197777746,0.380693558702874,
2.32622193849537));
#31042=CARTESIAN_POINT('Ctrl Pts',(0.0339164169991585,0.392535765776565,
2.36066180304628));
#31043=CARTESIAN_POINT('Ctrl Pts',(0.029986260998421,0.404607792760995,
2.3947592227875));
#31044=CARTESIAN_POINT('Ctrl Pts',(0.0263406370667108,0.417078684876168,
2.42897308992216));
#31045=CARTESIAN_POINT('Ctrl Pts',(0.0228702839178175,0.428950013497028,
2.46154205583053));
#31046=CARTESIAN_POINT('Ctrl Pts',(0.0196579772062671,0.441180495440324,
2.49421313164509));
#31047=CARTESIAN_POINT('Ctrl Pts',(0.0167223210422853,0.453948518005868,
2.52735622554626));
#31048=CARTESIAN_POINT('Ctrl Pts',(0.0139677607904214,0.465928901773376,
2.55845477523476));
#31049=CARTESIAN_POINT('Ctrl Pts',(0.0114564603784741,0.478382697242401,
2.58996911427275));
#31050=CARTESIAN_POINT('Ctrl Pts',(0.00923922793228618,0.491480864277342,
2.62218604509979));
#31051=CARTESIAN_POINT('Ctrl Pts',(0.00878499123326938,0.494164240198235,
2.62878621565768));
#31052=CARTESIAN_POINT('Ctrl Pts',(0.00834323197860242,0.496874740632172,
2.63541580115522));
#31053=CARTESIAN_POINT('Ctrl Pts',(0.00791460756900038,0.499613961471066,
2.64207714797975));
#31054=CARTESIAN_POINT('Ctrl Pts',(0.00537502089503349,0.515843762162931,
2.6815454266108));
#31055=CARTESIAN_POINT('Ctrl Pts',(0.00329666449988076,0.533066935814479,
2.72213393305126));
#31056=CARTESIAN_POINT('Ctrl Pts',(0.00190428975338371,0.551309292533906,
2.7635988904245));
#31057=CARTESIAN_POINT('Ctrl Pts',(0.000692060773595733,0.567191448922158,
2.79969910202339));
#31058=CARTESIAN_POINT('Ctrl Pts',(3.33158528145791E-7,0.583845999449411,
2.83646315076817));
#31059=CARTESIAN_POINT('Ctrl Pts',(1.31062334541924E-14,0.6012817622028,
2.873708690212));
#31060=CARTESIAN_POINT('Origin',(-0.5,0.6012817644084,2.87370869249));
#31061=CARTESIAN_POINT('Origin',(0.5,50.,0.));
#31062=CARTESIAN_POINT('',(0.517449748466302,0.145564568504214,3.5677191570162));
#31063=CARTESIAN_POINT('Origin',(0.5,0.6439853496966,3.532050807563));
#31064=CARTESIAN_POINT('Origin',(0.5174497483513,50.,0.));
#31065=CARTESIAN_POINT('Ctrl Pts',(0.001285090917852,0.6712313346096,3.501024393646));
#31066=CARTESIAN_POINT('Ctrl Pts',(0.00100370682231,0.6719071272873,3.510665341527));
#31067=CARTESIAN_POINT('Ctrl Pts',(0.0002345815242706,0.6756478789743,3.563478189283));
#31068=CARTESIAN_POINT('Ctrl Pts',(0.006495759564992,0.6828348068514,3.659504026904));
#31069=CARTESIAN_POINT('Ctrl Pts',(0.03172096583422,0.6932191711605,3.786961238567));
#31070=CARTESIAN_POINT('Ctrl Pts',(0.0735297005907,0.7041454719876,3.91068142931));
#31071=CARTESIAN_POINT('Ctrl Pts',(0.1164371395684,0.7124748329371,3.997808690824));
#31072=CARTESIAN_POINT('Ctrl Pts',(0.1438590078278,0.7170804204961,4.043718664671));
#31073=CARTESIAN_POINT('Ctrl Pts',(0.1489299286299,0.7179117303395,4.051932350288));
#31074=CARTESIAN_POINT('Ctrl Pts',(-0.01806331604683,0.3429577205548,3.52352261367));
#31075=CARTESIAN_POINT('Ctrl Pts',(-0.01835338084308,0.3436566094381,3.533493141926));
#31076=CARTESIAN_POINT('Ctrl Pts',(-0.01914623767077,0.3475252138821,3.588111304264));
#31077=CARTESIAN_POINT('Ctrl Pts',(-0.01269201706095,0.3549578839107,3.687418512264));
#31078=CARTESIAN_POINT('Ctrl Pts',(0.01331034779256,0.3656975079899,3.819229367317));
#31079=CARTESIAN_POINT('Ctrl Pts',(0.05640635123584,0.3769975825921,3.947173799546));
#31080=CARTESIAN_POINT('Ctrl Pts',(0.1006352724421,0.3856118388514,4.037276496891));
#31081=CARTESIAN_POINT('Ctrl Pts',(0.128901400684,0.3903747672857,4.08475381042));
#31082=CARTESIAN_POINT('Ctrl Pts',(0.1341284332036,0.3912344693522,4.093247883936));
#31083=CARTESIAN_POINT('Ctrl Pts',(0.2189431004029,0.1150380520537,3.546425312536));
#31084=CARTESIAN_POINT('Ctrl Pts',(0.2187174988582,0.1155840645799,3.554209879268));
#31085=CARTESIAN_POINT('Ctrl Pts',(0.2181008733428,0.1186055490003,3.596854451109));
#31086=CARTESIAN_POINT('Ctrl Pts',(0.2231215509742,0.1244016054761,3.674400795666));
#31087=CARTESIAN_POINT('Ctrl Pts',(0.2433526981449,0.1327577803046,3.777344386712));
#31088=CARTESIAN_POINT('Ctrl Pts',(0.2768893862856,0.1415339936859,3.877284136683));
#31089=CARTESIAN_POINT('Ctrl Pts',(0.3113049080117,0.1482130428467,3.947661212052));
#31090=CARTESIAN_POINT('Ctrl Pts',(0.333301521837,0.1519035194771,3.984749200474));
#31091=CARTESIAN_POINT('Ctrl Pts',(0.337369261638,0.1525695781223,3.991384739697));
#31092=CARTESIAN_POINT('Ctrl Pts',(0.5469709732897,0.1464668692464,3.553755790656));
#31093=CARTESIAN_POINT('Ctrl Pts',(0.5468380100126,0.14679067791,3.558363759427));
#31094=CARTESIAN_POINT('Ctrl Pts',(0.546474641405,0.1485810122013,3.583608495761));
#31095=CARTESIAN_POINT('Ctrl Pts',(0.5494352161253,0.1519997850887,3.629531909379));
#31096=CARTESIAN_POINT('Ctrl Pts',(0.561372714573,0.1568964726213,3.69052485114));
#31097=CARTESIAN_POINT('Ctrl Pts',(0.5811719886411,0.1620118107838,3.749766788604));
#31098=CARTESIAN_POINT('Ctrl Pts',(0.6014849610443,0.165885532055,3.791477585897));
#31099=CARTESIAN_POINT('Ctrl Pts',(0.6144718382275,0.1680218961319,3.813467076393));
#31100=CARTESIAN_POINT('Ctrl Pts',(0.6168735921791,0.1684073594755,3.817401654546));
#31101=CARTESIAN_POINT('',(0.584439525498375,0.166625640969186,3.82024992016299));
#31102=CARTESIAN_POINT('Origin',(0.5669897777871,0.6648591790704,3.782055102499));
#31103=CARTESIAN_POINT('Origin',(1.02904420412633,0.168033706666644,3.56616160740965));
#31104=CARTESIAN_POINT('Ctrl Pts',(0.1075904147796,0.6897997585045,3.984625378597));
#31105=CARTESIAN_POINT('Ctrl Pts',(0.2296596146426,0.7100892540097,4.196055434799));
#31106=CARTESIAN_POINT('Ctrl Pts',(0.5800094549946,0.7722604608586,4.802879158712));
#31107=CARTESIAN_POINT('Ctrl Pts',(1.173423480477,0.8967762996715,5.830702400772));
#31108=CARTESIAN_POINT('Ctrl Pts',(1.919928591278,1.086197265899,7.123687180788));
#31109=CARTESIAN_POINT('Ctrl Pts',(2.445873995284,1.245360410803,8.034651342534));
#31110=CARTESIAN_POINT('Ctrl Pts',(2.729006765993,1.338703235373,8.52505168669));
#31111=CARTESIAN_POINT('Ctrl Pts',(2.737553647736,1.341527957415,8.539855320115));
#31112=CARTESIAN_POINT('Ctrl Pts',(0.1045498530895,0.3724382569512,4.016835861329));
#31113=CARTESIAN_POINT('Ctrl Pts',(0.2272093052091,0.3928258600432,4.229288264428));
#31114=CARTESIAN_POINT('Ctrl Pts',(0.5792540041567,0.4552978195373,4.839047569541));
#31115=CARTESIAN_POINT('Ctrl Pts',(1.175543046931,0.5804168562544,5.871850487623));
#31116=CARTESIAN_POINT('Ctrl Pts',(1.925673807413,0.7707576941208,7.171115077098));
#31117=CARTESIAN_POINT('Ctrl Pts',(2.454181932341,0.9306962513913,8.086518001686));
#31118=CARTESIAN_POINT('Ctrl Pts',(2.73869719209,1.024494853114,8.5793128871));
#31119=CARTESIAN_POINT('Ctrl Pts',(2.747285809458,1.027333368668,8.594188808748));
#31120=CARTESIAN_POINT('Ctrl Pts',(0.308498647005,0.1467474938082,3.920743969836));
#31121=CARTESIAN_POINT('Ctrl Pts',(0.4315778554011,0.167204865842,4.133923412134));
#31122=CARTESIAN_POINT('Ctrl Pts',(0.7848278483999,0.2298907047566,4.745770347781));
#31123=CARTESIAN_POINT('Ctrl Pts',(1.383161451851,0.3554387040121,5.782114548835));
#31124=CARTESIAN_POINT('Ctrl Pts',(2.135870583181,0.5464337060764,7.085845007618));
#31125=CARTESIAN_POINT('Ctrl Pts',(2.666201180077,0.7069236957289,8.00440454625));
#31126=CARTESIAN_POINT('Ctrl Pts',(2.951699593123,0.8010464221266,8.498902303127));
#31127=CARTESIAN_POINT('Ctrl Pts',(2.960317890666,0.8038947468991,8.513829632345));
#31128=CARTESIAN_POINT('Ctrl Pts',(0.5837390273062,0.1628913043404,3.76028465105));
#31129=CARTESIAN_POINT('Ctrl Pts',(0.7067882102565,0.1833436857553,3.973412087749));
#31130=CARTESIAN_POINT('Ctrl Pts',(1.059951987769,0.2460142257326,4.585109693795));
#31131=CARTESIAN_POINT('Ctrl Pts',(1.658139342435,0.3715315410122,5.62120058452));
#31132=CARTESIAN_POINT('Ctrl Pts',(2.410664041181,0.562479750276,6.924611596699));
#31133=CARTESIAN_POINT('Ctrl Pts',(2.940864275444,0.7229302956031,7.842945340627));
#31134=CARTESIAN_POINT('Ctrl Pts',(3.22629236288,0.817029837147,8.337321289974));
#31135=CARTESIAN_POINT('Ctrl Pts',(3.23490853738,0.8198774602596,8.352244941975));
#31136=CARTESIAN_POINT('',(3.16400873341414,0.811418495172985,8.33346839762618));
#31137=CARTESIAN_POINT('Origin',(-2.23140270727043,50.6145742054134,-1.08622182306733));
#31138=CARTESIAN_POINT('Origin',(3.146558985788,1.304093376118,8.250000032393));
#31139=CARTESIAN_POINT('Ctrl Pts',(2.697976171111,1.328291304826,8.470478725465));
#31140=CARTESIAN_POINT('Ctrl Pts',(2.702496427436,1.32989020433,8.478861959952));
#31141=CARTESIAN_POINT('Ctrl Pts',(2.741672170872,1.343336298271,8.549038004148));
#31142=CARTESIAN_POINT('Ctrl Pts',(2.830553529668,1.36759303881,8.670613831123));
#31143=CARTESIAN_POINT('Ctrl Pts',(2.985965248763,1.397432557112,8.808744119105));
#31144=CARTESIAN_POINT('Ctrl Pts',(3.163320103837,1.421879840356,8.910729967018));
#31145=CARTESIAN_POINT('Ctrl Pts',(3.361331922286,1.440697594273,8.976477330544));
#31146=CARTESIAN_POINT('Ctrl Pts',(3.512953212907,1.449081077376,8.993152567829));
#31147=CARTESIAN_POINT('Ctrl Pts',(3.596210880627,1.45181260013,8.991916516691));
#31148=CARTESIAN_POINT('Ctrl Pts',(3.606094403736,1.452110276979,8.991622099435));
#31149=CARTESIAN_POINT('Ctrl Pts',(2.707229713817,1.02483114282,8.522615032357));
#31150=CARTESIAN_POINT('Ctrl Pts',(2.711757531714,1.026437245798,8.531038853544));
#31151=CARTESIAN_POINT('Ctrl Pts',(2.750998819302,1.039943784245,8.601554659816));
#31152=CARTESIAN_POINT('Ctrl Pts',(2.840029078046,1.064307470111,8.72371926588));
#31153=CARTESIAN_POINT('Ctrl Pts',(2.995702241282,1.094273334906,8.86251873823));
#31154=CARTESIAN_POINT('Ctrl Pts',(3.173356931632,1.118818630411,8.964999159331));
#31155=CARTESIAN_POINT('Ctrl Pts',(3.37170509839,1.13770523227,9.031066488327));
#31156=CARTESIAN_POINT('Ctrl Pts',(3.523584957284,1.146112696876,9.04782465196));
#31157=CARTESIAN_POINT('Ctrl Pts',(3.606984784191,1.148848479805,9.046584219238));
#31158=CARTESIAN_POINT('Ctrl Pts',(3.61688518525,1.149146535858,9.046288572707));
#31159=CARTESIAN_POINT('Ctrl Pts',(2.911986615036,0.8053087593334,8.453506053933));
#31160=CARTESIAN_POINT('Ctrl Pts',(2.915517483284,0.8065606383852,8.46009945291));
#31161=CARTESIAN_POINT('Ctrl Pts',(2.946117152648,0.8170869048461,8.515290469754));
#31162=CARTESIAN_POINT('Ctrl Pts',(3.015515812346,0.8360518603861,8.610867703186));
#31163=CARTESIAN_POINT('Ctrl Pts',(3.136719074313,0.8593273898185,8.719331257004));
#31164=CARTESIAN_POINT('Ctrl Pts',(3.274842213709,0.8783567362483,8.799303634155));
#31165=CARTESIAN_POINT('Ctrl Pts',(3.428844796628,0.8929793997328,8.850790670297));
#31166=CARTESIAN_POINT('Ctrl Pts',(3.546633920865,0.8994873453306,8.863833347941));
#31167=CARTESIAN_POINT('Ctrl Pts',(3.611290879112,0.9016089397426,8.862870550793));
#31168=CARTESIAN_POINT('Ctrl Pts',(3.61896601985,0.9018401752654,8.862640837198));
#31169=CARTESIAN_POINT('Ctrl Pts',(3.182848628904,0.8084535997814,8.306825925367));
#31170=CARTESIAN_POINT('Ctrl Pts',(3.185008068947,0.809213682988,8.310874647509));
#31171=CARTESIAN_POINT('Ctrl Pts',(3.20372011791,0.81560237474,8.344760982929));
#31172=CARTESIAN_POINT('Ctrl Pts',(3.246113072049,0.8270747078833,8.403376857699));
#31173=CARTESIAN_POINT('Ctrl Pts',(3.319898698697,0.8410712468725,8.469670488211));
#31174=CARTESIAN_POINT('Ctrl Pts',(3.403641274247,0.8524565440747,8.518356395924));
#31175=CARTESIAN_POINT('Ctrl Pts',(3.496640992492,0.8611771229168,8.54957704807));
#31176=CARTESIAN_POINT('Ctrl Pts',(3.567534072232,0.8650624697199,8.557453867267));
#31177=CARTESIAN_POINT('Ctrl Pts',(3.606407884075,0.8663395697229,8.556875268173));
#31178=CARTESIAN_POINT('Ctrl Pts',(3.611021902544,0.8664790129072,8.556736982723));
#31179=CARTESIAN_POINT('',(3.579571669199,1.362459037518,9.));
#31180=CARTESIAN_POINT('Ctrl Pts',(2.71354627750015,1.3040933719743,8.50000002131796));
#31181=CARTESIAN_POINT('Ctrl Pts',(2.73240780783335,1.30718564412007,8.53266776695291));
#31182=CARTESIAN_POINT('Ctrl Pts',(2.75295855457772,1.31021121384129,8.56397556110528));
#31183=CARTESIAN_POINT('Ctrl Pts',(2.77500953840381,1.31315034809672,8.59385060141172));
#31184=CARTESIAN_POINT('Ctrl Pts',(2.79564689372688,1.31590106246167,8.62181043426805));
#31185=CARTESIAN_POINT('Ctrl Pts',(2.8175992397998,1.31857622541632,8.64851590702357));
#31186=CARTESIAN_POINT('Ctrl Pts',(2.84075275697417,1.32116110135567,8.67390401044094));
#31187=CARTESIAN_POINT('Ctrl Pts',(2.86139502942833,1.32346562006004,8.69653850453914));
#31188=CARTESIAN_POINT('Ctrl Pts',(2.88300033530865,1.32570076855028,8.71812559348188));
#31189=CARTESIAN_POINT('Ctrl Pts',(2.9053417331799,1.3278487177207,8.73852142578194));
#31190=CARTESIAN_POINT('Ctrl Pts',(2.9276224102888,1.32999082906881,8.75886182509195));
#31191=CARTESIAN_POINT('Ctrl Pts',(2.9506345494046,1.33204612157451,8.77801710890381));
#31192=CARTESIAN_POINT('Ctrl Pts',(2.97412950703109,1.33400408893246,8.79589009824868));
#31193=CARTESIAN_POINT('Ctrl Pts',(2.98173577942302,1.33463796251912,8.80167631108535));
#31194=CARTESIAN_POINT('Ctrl Pts',(2.98939251035384,1.3352616975211,8.80732850506171));
#31195=CARTESIAN_POINT('Ctrl Pts',(2.99709090026803,1.33587512176817,8.81284448333751));
#31196=CARTESIAN_POINT('Ctrl Pts',(3.01817510751269,1.33755515669732,8.82795154214076));
#31197=CARTESIAN_POINT('Ctrl Pts',(3.03956856536244,1.33915243335482,8.84204027731431));
#31198=CARTESIAN_POINT('Ctrl Pts',(3.06130422044454,1.34067812790984,8.85521079188191));
#31199=CARTESIAN_POINT('Ctrl Pts',(3.08331169847731,1.34222290257973,8.8685460149949));
#31200=CARTESIAN_POINT('Ctrl Pts',(3.10567056825425,1.34369438926915,8.88094026547201));
#31201=CARTESIAN_POINT('Ctrl Pts',(3.12844969744608,1.34509853175425,8.89245753558751));
#31202=CARTESIAN_POINT('Ctrl Pts',(3.14220400284712,1.34594636945708,8.89941179837871));
#31203=CARTESIAN_POINT('Ctrl Pts',(3.15611215472,1.34676953926675,8.90604553466176));
#31204=CARTESIAN_POINT('Ctrl Pts',(3.17019402171472,1.34756813901533,8.91236502669045));
#31205=CARTESIAN_POINT('Ctrl Pts',(3.19363757911981,1.34889765157618,8.92288574629397));
#31206=CARTESIAN_POINT('Ctrl Pts',(3.21754745231044,1.3501582134814,8.93253160234711));
#31207=CARTESIAN_POINT('Ctrl Pts',(3.24201675624197,1.35135481993116,8.94130645721643));
#31208=CARTESIAN_POINT('Ctrl Pts',(3.26586440232776,1.35252102585176,8.94985838145439));
#31209=CARTESIAN_POINT('Ctrl Pts',(3.29024397859368,1.35362654202181,8.95758316176405));
#31210=CARTESIAN_POINT('Ctrl Pts',(3.31525278905935,1.35466793937946,8.96443755649156));
#31211=CARTESIAN_POINT('Ctrl Pts',(3.33073613975584,1.35531268497921,8.96868122084033));
#31212=CARTESIAN_POINT('Ctrl Pts',(3.34646086769962,1.35593269322772,8.97259033901732));
#31213=CARTESIAN_POINT('Ctrl Pts',(3.36245086038982,1.35652537029808,8.9761447405435));
#31214=CARTESIAN_POINT('Ctrl Pts',(3.39660962826479,1.35779148210085,8.98373786325591));
#31215=CARTESIAN_POINT('Ctrl Pts',(3.43197070713738,1.35894127328653,8.98970505443759));
#31216=CARTESIAN_POINT('Ctrl Pts',(3.46825922074053,1.35994135206922,8.9937705445444));
#31217=CARTESIAN_POINT('Ctrl Pts',(3.50454773434368,1.36094143085192,8.99783603465122));
#31218=CARTESIAN_POINT('Ctrl Pts',(3.5417633787783,1.36179176414304,8.99999968426863));
#31219=CARTESIAN_POINT('Ctrl Pts',(3.579571669199,1.362459037518,8.99999999999982));
#31220=CARTESIAN_POINT('',(3.597021417327,0.8702239620615,8.586024047651));
#31221=CARTESIAN_POINT('Ctrl Pts',(3.16400873340959,0.811418495170706,8.33346839762921));
#31222=CARTESIAN_POINT('Ctrl Pts',(3.18251475913057,0.81755879068723,8.36584286454173));
#31223=CARTESIAN_POINT('Ctrl Pts',(3.20370582008103,0.823267569144944,8.3949175534773));
#31224=CARTESIAN_POINT('Ctrl Pts',(3.22761204491947,0.828633602007933,8.42130397461794));
#31225=CARTESIAN_POINT('Ctrl Pts',(3.25151827749776,0.833999636608221,8.44769040430141));
#31226=CARTESIAN_POINT('Ctrl Pts',(3.2781396477692,0.839023714446743,8.47138842976006));
#31227=CARTESIAN_POINT('Ctrl Pts',(3.30578098628547,0.843474250546619,8.4914816817855));
#31228=CARTESIAN_POINT('Ctrl Pts',(3.33342232480175,0.847924786646494,8.51157493381093));
#31229=CARTESIAN_POINT('Ctrl Pts',(3.36208365741291,0.851801051595527,8.52806353860089));
#31230=CARTESIAN_POINT('Ctrl Pts',(3.39233262875664,0.855252149752825,8.54175073446735));
#31231=CARTESIAN_POINT('Ctrl Pts',(3.42258160010037,0.858703247910124,8.55543793033381));
#31232=CARTESIAN_POINT('Ctrl Pts',(3.45441819613419,0.861729575415374,8.56632364815803));
#31233=CARTESIAN_POINT('Ctrl Pts',(3.48846097084022,0.864270436217875,8.57396910073167));
#31234=CARTESIAN_POINT('Ctrl Pts',(3.52250374554625,0.866811297020377,8.58161455330531));
#31235=CARTESIAN_POINT('Ctrl Pts',(3.55875270266928,0.868866585502102,8.58601975919096));
#31236=CARTESIAN_POINT('Ctrl Pts',(3.59702141732714,0.870223962057679,8.58602404765169));
#31237=CARTESIAN_POINT('Origin',(3.579571668976,1.362459037517,8.5));
#31238=CARTESIAN_POINT('Origin',(3.579571668976,17.50736,8.));
#31239=CARTESIAN_POINT('',(3.57957168230051,6.23754096186244,9.00000000000025));
#31240=CARTESIAN_POINT('Ctrl Pts',(3.579571669193,6.237540962482,9.));
#31241=CARTESIAN_POINT('Ctrl Pts',(3.53011728241888,6.23841424781783,9.00000000001073));
#31242=CARTESIAN_POINT('Ctrl Pts',(3.48117061949772,6.23960201462633,8.99633236936105));
#31243=CARTESIAN_POINT('Ctrl Pts',(3.43310495241581,6.24107719429828,8.98921559881559));
#31244=CARTESIAN_POINT('Ctrl Pts',(3.41090223035401,6.24175861632436,8.98592818624043));
#31245=CARTESIAN_POINT('Ctrl Pts',(3.3888867000059,6.24250136492367,8.9819046412304));
#31246=CARTESIAN_POINT('Ctrl Pts',(3.36709170786865,6.24330277213392,8.97716542413648));
#31247=CARTESIAN_POINT('Ctrl Pts',(3.33744658181104,6.24439283069516,8.97071923286102));
#31248=CARTESIAN_POINT('Ctrl Pts',(3.30820446262744,6.24559141304431,8.96294344610757));
#31249=CARTESIAN_POINT('Ctrl Pts',(3.27958235305604,6.24688296887885,8.95394256133893));
#31250=CARTESIAN_POINT('Ctrl Pts',(3.25079015911753,6.24818219967028,8.94488818960472));
#31251=CARTESIAN_POINT('Ctrl Pts',(3.22262595615722,6.24957551220371,8.93459447260509));
#31252=CARTESIAN_POINT('Ctrl Pts',(3.19528464198247,6.25104707730712,8.92321367022184));
#31253=CARTESIAN_POINT('Ctrl Pts',(3.18656406822489,6.25151643631237,8.9195837376601));
#31254=CARTESIAN_POINT('Ctrl Pts',(3.1779269748766,6.2519937559938,8.91584353960427));
#31255=CARTESIAN_POINT('Ctrl Pts',(3.16937899398663,6.25247852273933,8.91199888672359));
#31256=CARTESIAN_POINT('Ctrl Pts',(3.14459614848154,6.25388398907288,8.90085222652524));
#31257=CARTESIAN_POINT('Ctrl Pts',(3.12056218077246,6.25535205339036,8.88883262541388));
#31258=CARTESIAN_POINT('Ctrl Pts',(3.09717010751247,6.25688421677726,8.8759501889363));
#31259=CARTESIAN_POINT('Ctrl Pts',(3.07357809068857,6.25842947631876,8.86295763993332));
#31260=CARTESIAN_POINT('Ctrl Pts',(3.05063831677839,6.26003993538532,8.8490870940687));
#31261=CARTESIAN_POINT('Ctrl Pts',(3.02826126562333,6.26171713388391,8.83430020925031));
#31262=CARTESIAN_POINT('Ctrl Pts',(3.01732772911007,6.26253662126396,8.82707526508949));
#31263=CARTESIAN_POINT('Ctrl Pts',(3.00652890218638,6.26337204166456,8.81963085750914));
#31264=CARTESIAN_POINT('Ctrl Pts',(2.99585681279478,6.26422357471117,8.81195872227185));
#31265=CARTESIAN_POINT('Ctrl Pts',(2.97302911160615,6.26604501203492,8.79554795168614));
#31266=CARTESIAN_POINT('Ctrl Pts',(2.95079225545371,6.26794017054501,8.77810692567441));
#31267=CARTESIAN_POINT('Ctrl Pts',(2.92912259389889,6.26991940834275,8.7595498671788));
#31268=CARTESIAN_POINT('Ctrl Pts',(2.90794523902614,6.27185368041776,8.74141440104973));
#31269=CARTESIAN_POINT('Ctrl Pts',(2.88730911650271,6.27386825483174,8.7222124749539));
#31270=CARTESIAN_POINT('Ctrl Pts',(2.8672324480952,6.27597279963524,8.70183533282027));
#31271=CARTESIAN_POINT('Ctrl Pts',(2.85910235513914,6.27682503988423,8.6935835623391));
#31272=CARTESIAN_POINT('Ctrl Pts',(2.85106451293426,6.27769203405006,8.68513878574988));
#31273=CARTESIAN_POINT('Ctrl Pts',(2.84312235741875,6.27857442415559,8.67649272834736));
#31274=CARTESIAN_POINT('Ctrl Pts',(2.82117822934304,6.28101246272719,8.65260372357777));
#31275=CARTESIAN_POINT('Ctrl Pts',(2.79996899724937,6.28356803599439,8.62717678449721));
#31276=CARTESIAN_POINT('Ctrl Pts',(2.77978100812815,6.28622141984332,8.60027901747484));
#31277=CARTESIAN_POINT('Ctrl Pts',(2.75981064432942,6.28884620037211,8.57367120678183));
#31278=CARTESIAN_POINT('Ctrl Pts',(2.74084026265292,6.29156669406441,8.54562420429965));
#31279=CARTESIAN_POINT('Ctrl Pts',(2.72313539509604,6.29436380782913,8.51625275668281));
#31280=CARTESIAN_POINT('Ctrl Pts',(2.71989618577763,6.29487555619111,8.51087907814442));
#31281=CARTESIAN_POINT('Ctrl Pts',(2.716699290052,6.2953898692451,8.50546119925901));
#31282=CARTESIAN_POINT('Ctrl Pts',(2.71354626506509,6.295906630064,8.49999999978095));
#31283=CARTESIAN_POINT('',(3.579571669193,6.237540962482,9.));
#31284=CARTESIAN_POINT('Ctrl Pts',(3.606118543797,6.147888877213,8.991622020187));
#31285=CARTESIAN_POINT('Ctrl Pts',(3.596226611735,6.14818683719,8.991916533163));
#31286=CARTESIAN_POINT('Ctrl Pts',(3.514543691835,6.150866828852,8.9931285392));
#31287=CARTESIAN_POINT('Ctrl Pts',(3.362649869023,6.159198407814,8.976794092479));
#31288=CARTESIAN_POINT('Ctrl Pts',(3.163916181684,6.178009793471,8.911233217637));
#31289=CARTESIAN_POINT('Ctrl Pts',(2.986337602701,6.202539765663,8.808822625203));
#31290=CARTESIAN_POINT('Ctrl Pts',(2.831066145079,6.232302140706,8.671103691814));
#31291=CARTESIAN_POINT('Ctrl Pts',(2.742230088108,6.256472013443,8.550038566438));
#31292=CARTESIAN_POINT('Ctrl Pts',(2.702500721408,6.270108389296,8.478869254392));
#31293=CARTESIAN_POINT('Ctrl Pts',(2.69798283987,6.271706509569,8.47049007187));
#31294=CARTESIAN_POINT('Ctrl Pts',(3.616909366482,6.450852618565,9.046288493852));
#31295=CARTESIAN_POINT('Ctrl Pts',(3.607000542165,6.451150958213,9.046584236403));
#31296=CARTESIAN_POINT('Ctrl Pts',(3.525178152179,6.453835130108,9.047800537919));
#31297=CARTESIAN_POINT('Ctrl Pts',(3.373025288817,6.462190415094,9.031384796543));
#31298=CARTESIAN_POINT('Ctrl Pts',(3.173954011786,6.481070540639,8.965504847357));
#31299=CARTESIAN_POINT('Ctrl Pts',(2.996075229086,6.505698897314,8.862597627541));
#31300=CARTESIAN_POINT('Ctrl Pts',(2.840542553224,6.535587263935,8.724211499603));
#31301=CARTESIAN_POINT('Ctrl Pts',(2.751557670134,6.559863667414,8.602560066809));
#31302=CARTESIAN_POINT('Ctrl Pts',(2.711761832896,6.57356134326,8.531046183576));
#31303=CARTESIAN_POINT('Ctrl Pts',(2.707236393739,6.575166663517,8.522626433943));
#31304=CARTESIAN_POINT('Ctrl Pts',(3.61898478102,6.698159168706,8.862640776355));
#31305=CARTESIAN_POINT('Ctrl Pts',(3.61130310312,6.698390624919,8.862870563926));
#31306=CARTESIAN_POINT('Ctrl Pts',(3.547869039179,6.700472197892,8.863814624792));
#31307=CARTESIAN_POINT('Ctrl Pts',(3.429869177846,6.706939900386,8.851038343534));
#31308=CARTESIAN_POINT('Ctrl Pts',(3.275307153675,6.7215572598,8.799698550945));
#31309=CARTESIAN_POINT('Ctrl Pts',(3.137008498961,6.7406511827,8.719392459593));
#31310=CARTESIAN_POINT('Ctrl Pts',(3.015915940792,6.763866383704,8.611252396668));
#31311=CARTESIAN_POINT('Ctrl Pts',(2.946552922871,6.782763032102,8.516077397137));
#31312=CARTESIAN_POINT('Ctrl Pts',(2.915520842571,6.793438263292,8.460105184664));
#31313=CARTESIAN_POINT('Ctrl Pts',(2.911991831747,6.794689532614,8.453514967436));
#31314=CARTESIAN_POINT('Ctrl Pts',(3.611033207671,6.733520588822,8.556736947109));
#31315=CARTESIAN_POINT('Ctrl Pts',(3.60641524659,6.733660166175,8.55687527608));
#31316=CARTESIAN_POINT('Ctrl Pts',(3.568276611501,6.734913179705,8.557442605468));
#31317=CARTESIAN_POINT('Ctrl Pts',(3.497258450995,6.738774888522,8.54972654454));
#31318=CARTESIAN_POINT('Ctrl Pts',(3.403924438349,6.747491875044,8.51859733675));
#31319=CARTESIAN_POINT('Ctrl Pts',(3.320073171016,6.758916088725,8.469707112214));
#31320=CARTESIAN_POINT('Ctrl Pts',(3.246357276968,6.772876143129,8.403612059442));
#31321=CARTESIAN_POINT('Ctrl Pts',(3.203986574343,6.78430654263,8.345244177306));
#31322=CARTESIAN_POINT('Ctrl Pts',(3.185010131382,6.790785649759,8.310878157544));
#31323=CARTESIAN_POINT('Ctrl Pts',(3.182851831626,6.791545363384,8.306831380263));
#31324=CARTESIAN_POINT('',(3.59702142700201,6.72977603759518,8.58602404765126));
#31325=CARTESIAN_POINT('Origin',(3.57957168907,6.237540961771,8.500000000001));
#31326=CARTESIAN_POINT('',(3.164008715435,6.788581510789,8.333468366184));
#31327=CARTESIAN_POINT('Ctrl Pts',(3.597021417327,6.7297760379381,8.58602404765102));
#31328=CARTESIAN_POINT('Ctrl Pts',(3.58088597603724,6.73034837177699,8.58602214343887));
#31329=CARTESIAN_POINT('Ctrl Pts',(3.56502302749176,6.73104708591087,8.58524234323971));
#31330=CARTESIAN_POINT('Ctrl Pts',(3.54938881284648,6.73186430375203,8.58373710784466));
#31331=CARTESIAN_POINT('Ctrl Pts',(3.53334636737609,6.73270286027384,8.58219256868531));
#31332=CARTESIAN_POINT('Ctrl Pts',(3.5175438291784,6.73366625394346,8.57988406271693));
#31333=CARTESIAN_POINT('Ctrl Pts',(3.50193410093652,6.7347552796972,8.57681507176309));
#31334=CARTESIAN_POINT('Ctrl Pts',(3.49820568216472,6.73501539595293,8.57608203635687));
#31335=CARTESIAN_POINT('Ctrl Pts',(3.49448829989847,6.73528271796873,8.57530538710957));
#31336=CARTESIAN_POINT('Ctrl Pts',(3.49078140477858,6.73555732665343,8.57448474949574));
#31337=CARTESIAN_POINT('Ctrl Pts',(3.47360580500939,6.73682970386104,8.57068239125389));
#31338=CARTESIAN_POINT('Ctrl Pts',(3.45664662919491,6.7382522489223,8.565973303512));
#31339=CARTESIAN_POINT('Ctrl Pts',(3.44010684884663,6.73980100233827,8.56044841819582));
#31340=CARTESIAN_POINT('Ctrl Pts',(3.42356706849835,6.74134975575425,8.55492353287965));
#31341=CARTESIAN_POINT('Ctrl Pts',(3.40744744894976,6.74302460283963,8.54858330475174));
#31342=CARTESIAN_POINT('Ctrl Pts',(3.39192510545283,6.74479444026113,8.54156578324247));
#31343=CARTESIAN_POINT('Ctrl Pts',(3.37807378237151,6.74637375010771,8.5353037160698));
#31344=CARTESIAN_POINT('Ctrl Pts',(3.3647095305328,6.74803262883628,8.52847746681804));
#31345=CARTESIAN_POINT('Ctrl Pts',(3.35174356115493,6.74977086519574,8.5211019478325));
#31346=CARTESIAN_POINT('Ctrl Pts',(3.33862508481612,6.75152954685604,8.51363967729348));
#31347=CARTESIAN_POINT('Ctrl Pts',(3.32591360725994,6.7533695599748,8.50561478592258));
#31348=CARTESIAN_POINT('Ctrl Pts',(3.31353616043678,6.75529834751392,8.49699420783524));
#31349=CARTESIAN_POINT('Ctrl Pts',(3.31072834626721,6.75573589146461,8.49503863641172));
#31350=CARTESIAN_POINT('Ctrl Pts',(3.30793782318856,6.75617803139363,8.49305222690647));
#31351=CARTESIAN_POINT('Ctrl Pts',(3.30516393353998,6.75662490076,8.49103427713288));
#31352=CARTESIAN_POINT('Ctrl Pts',(3.29133031694917,6.75885347516771,8.48097059508209));
#31353=CARTESIAN_POINT('Ctrl Pts',(3.27790939081006,6.76119658123771,8.47014077335627));
#31354=CARTESIAN_POINT('Ctrl Pts',(3.26491581809246,6.76366283998476,8.45848214059525));
#31355=CARTESIAN_POINT('Ctrl Pts',(3.25246674010343,6.7660257503367,8.44731206200011));
#31356=CARTESIAN_POINT('Ctrl Pts',(3.24040961873387,6.76850182512087,8.43538062366922));
#31357=CARTESIAN_POINT('Ctrl Pts',(3.22879686755357,6.77110046653676,8.42261152045667));
#31358=CARTESIAN_POINT('Ctrl Pts',(3.21693015853769,6.77375593732402,8.40956317128735));
#31359=CARTESIAN_POINT('Ctrl Pts',(3.20553108667914,6.77653839520581,8.39564525193401));
#31360=CARTESIAN_POINT('Ctrl Pts',(3.19469271145958,6.7794511503701,8.38080593133939));
#31361=CARTESIAN_POINT('Ctrl Pts',(3.18448743738699,6.78219376299937,8.36683341879471));
#31362=CARTESIAN_POINT('Ctrl Pts',(3.17477900744225,6.78505201880737,8.35204337981397));
#31363=CARTESIAN_POINT('Ctrl Pts',(3.16569253133343,6.78802657658399,8.33639132777214));
#31364=CARTESIAN_POINT('Ctrl Pts',(3.16512883667855,6.78821110822191,8.33542032669666));
#31365=CARTESIAN_POINT('Ctrl Pts',(3.16456755246907,6.7883960863902,8.33444600947876));
#31366=CARTESIAN_POINT('Ctrl Pts',(3.164008715435,6.78858151078889,8.33346836618398));
#31367=CARTESIAN_POINT('Origin',(3.14655896696,6.295906630073,8.249999999787));
#31368=CARTESIAN_POINT('Ctrl Pts',(2.73755431537,6.258471820398,8.539856476492));
#31369=CARTESIAN_POINT('Ctrl Pts',(2.729007207951,6.261296617751,8.525052452183));
#31370=CARTESIAN_POINT('Ctrl Pts',(2.498328684723,6.33734641652,8.125505529738));
#31371=CARTESIAN_POINT('Ctrl Pts',(2.04242243337,6.477595338386,7.335852738906));
#31372=CARTESIAN_POINT('Ctrl Pts',(1.343393624252,6.663026878556,6.12509932556));
#31373=CARTESIAN_POINT('Ctrl Pts',(0.6974672715952,6.805597994089,5.00632206481));
#31374=CARTESIAN_POINT('Ctrl Pts',(0.2768280555865,6.882070724215,4.277753571027));
#31375=CARTESIAN_POINT('Ctrl Pts',(0.107591124226,6.91020011954,3.984626607394));
#31376=CARTESIAN_POINT('Ctrl Pts',(2.747286480821,6.572666423231,8.594189973393));
#31377=CARTESIAN_POINT('Ctrl Pts',(2.738697636674,6.575505014465,8.579313658951));
#31378=CARTESIAN_POINT('Ctrl Pts',(2.506892749498,6.651926151471,8.17781581692));
#31379=CARTESIAN_POINT('Ctrl Pts',(2.048764186804,6.792858642713,7.384313869934));
#31380=CARTESIAN_POINT('Ctrl Pts',(1.346337835851,6.979191351984,6.167675741509));
#31381=CARTESIAN_POINT('Ctrl Pts',(0.6972802940191,7.122453502016,5.043475102021));
#31382=CARTESIAN_POINT('Ctrl Pts',(0.2746058239404,7.199296224689,4.311381444782));
#31383=CARTESIAN_POINT('Ctrl Pts',(0.1045505658565,7.227561636244,4.016837097687));
#31384=CARTESIAN_POINT('Ctrl Pts',(2.960318580227,6.796105048041,8.513830792565));
#31385=CARTESIAN_POINT('Ctrl Pts',(2.951700055121,6.798953448756,8.498903069194));
#31386=CARTESIAN_POINT('Ctrl Pts',(2.719094157332,6.875638661924,8.096017836083));
#31387=CARTESIAN_POINT('Ctrl Pts',(2.259385204058,7.017057271642,7.29977857232));
#31388=CARTESIAN_POINT('Ctrl Pts',(1.554542700605,7.204030844833,6.078955545004));
#31389=CARTESIAN_POINT('Ctrl Pts',(0.9032584222318,7.347784422142,4.950898084692));
#31390=CARTESIAN_POINT('Ctrl Pts',(0.4791365868375,7.424890263994,4.216297517189));
#31391=CARTESIAN_POINT('Ctrl Pts',(0.3084993779623,7.453252403116,3.920745201756));
#31392=CARTESIAN_POINT('Ctrl Pts',(3.234909237514,6.780122314181,8.352246091786));
#31393=CARTESIAN_POINT('Ctrl Pts',(3.226292835509,6.782970013216,8.337322045735));
#31394=CARTESIAN_POINT('Ctrl Pts',(2.993744234615,6.859636336817,7.934536053757));
#31395=CARTESIAN_POINT('Ctrl Pts',(2.534148327875,7.001020174112,7.138492592334));
#31396=CARTESIAN_POINT('Ctrl Pts',(1.829478653638,7.187947905822,5.917968914001));
#31397=CARTESIAN_POINT('Ctrl Pts',(1.178353655414,7.331666330967,4.790187335));
#31398=CARTESIAN_POINT('Ctrl Pts',(0.7543353511557,7.408753351705,4.055766088685));
#31399=CARTESIAN_POINT('Ctrl Pts',(0.5837397696607,7.437108571831,3.760285873989));
#31400=CARTESIAN_POINT('',(0.584436889085312,7.43337480914178,3.82024522397442));
#31401=CARTESIAN_POINT('Origin',(0.5669871034298,6.935141265841,3.782050470377));
#31402=CARTESIAN_POINT('Origin',(-2.20586704229758,-42.6932679752466,-1.0417272484549));
#31403=CARTESIAN_POINT('Ctrl Pts',(0.1488993839097,6.882092998737,4.051886316842));
#31404=CARTESIAN_POINT('Ctrl Pts',(0.1391249419216,6.883695858063,4.036047063007));
#31405=CARTESIAN_POINT('Ctrl Pts',(0.1187380670595,6.887199773797,4.000833626095));
#31406=CARTESIAN_POINT('Ctrl Pts',(0.09068402979308,6.892584054817,3.944687824196));
#31407=CARTESIAN_POINT('Ctrl Pts',(0.06509502960357,6.898211837795,3.883612722829));
#31408=CARTESIAN_POINT('Ctrl Pts',(0.04362719886288,6.903757390935,3.820964525266));
#31409=CARTESIAN_POINT('Ctrl Pts',(0.02637474659593,6.9091924048,3.757016860335));
#31410=CARTESIAN_POINT('Ctrl Pts',(0.0134143459347,6.914489765827,3.692048579365));
#31411=CARTESIAN_POINT('Ctrl Pts',(0.004805063189619,6.919623625663,3.626343926084));
#31412=CARTESIAN_POINT('Ctrl Pts',(0.0007382764448709,6.924391993813,3.562568427967));
#31413=CARTESIAN_POINT('Ctrl Pts',(0.000710719447065,6.927386121703,3.520747207447));
#31414=CARTESIAN_POINT('Ctrl Pts',(0.001283507568449,6.928767604726,3.501041178649));
#31415=CARTESIAN_POINT('Ctrl Pts',(0.1340961482713,7.208770547067,4.09319900537));
#31416=CARTESIAN_POINT('Ctrl Pts',(0.1240204805176,7.210428200377,4.076818539986));
#31417=CARTESIAN_POINT('Ctrl Pts',(0.103007671651,7.214051571443,4.040405692018));
#31418=CARTESIAN_POINT('Ctrl Pts',(0.07408852360614,7.219620173195,3.982340497052));
#31419=CARTESIAN_POINT('Ctrl Pts',(0.04771230919604,7.225440313667,3.919181444569));
#31420=CARTESIAN_POINT('Ctrl Pts',(0.02558314411504,7.231175635589,3.854393383835));
#31421=CARTESIAN_POINT('Ctrl Pts',(0.007799466531112,7.236796549271,3.788262308255));
#31422=CARTESIAN_POINT('Ctrl Pts',(-0.005560285788121,7.24227518205,3.721074180306));
#31423=CARTESIAN_POINT('Ctrl Pts',(-0.01443475371415,7.247584520523,3.653126248775));
#31424=CARTESIAN_POINT('Ctrl Pts',(-0.01862695084338,7.252516147052,3.587168415754));
#31425=CARTESIAN_POINT('Ctrl Pts',(-0.0186554368296,7.255612364638,3.543921256501));
#31426=CARTESIAN_POINT('Ctrl Pts',(-0.01806494151223,7.257041119415,3.523540741356));
#31427=CARTESIAN_POINT('Ctrl Pts',(0.3373468469199,7.447433892025,3.99135077941));
#31428=CARTESIAN_POINT('Ctrl Pts',(0.3295060114974,7.448718119987,3.978555091384));
#31429=CARTESIAN_POINT('Ctrl Pts',(0.3131537888847,7.451525913903,3.950110871236));
#31430=CARTESIAN_POINT('Ctrl Pts',(0.2906487244678,7.455843821799,3.904752830445));
#31431=CARTESIAN_POINT('Ctrl Pts',(0.2701232225468,7.46036004213,3.85541761694));
#31432=CARTESIAN_POINT('Ctrl Pts',(0.2529031715268,7.464814116684,3.804811783341));
#31433=CARTESIAN_POINT('Ctrl Pts',(0.239065347631,7.469183247015,3.753160061754));
#31434=CARTESIAN_POINT('Ctrl Pts',(0.2286704731386,7.473445999966,3.700686137549));
#31435=CARTESIAN_POINT('Ctrl Pts',(0.2217660378869,7.477581471328,3.647623379189));
#31436=CARTESIAN_POINT('Ctrl Pts',(0.2185047232103,7.481427316599,3.596118768688));
#31437=CARTESIAN_POINT('Ctrl Pts',(0.2184826254111,7.483844809718,3.562351628979));
#31438=CARTESIAN_POINT('Ctrl Pts',(0.2189419428023,7.484961027628,3.546439410883));
#31439=CARTESIAN_POINT('Ctrl Pts',(0.6168657783813,7.431593816078,3.817389966263));
#31440=CARTESIAN_POINT('Ctrl Pts',(0.6122368361889,7.432336897234,3.809804338841));
#31441=CARTESIAN_POINT('Ctrl Pts',(0.6025805406548,7.433963020169,3.792937948481));
#31442=CARTESIAN_POINT('Ctrl Pts',(0.5892943522034,7.436467691435,3.766049222514));
#31443=CARTESIAN_POINT('Ctrl Pts',(0.5771760896146,7.439093315939,3.736802263077));
#31444=CARTESIAN_POINT('Ctrl Pts',(0.5670110510533,7.441688912623,3.706807363841));
#31445=CARTESIAN_POINT('Ctrl Pts',(0.5588435708717,7.444241808268,3.676197105016));
#31446=CARTESIAN_POINT('Ctrl Pts',(0.5527095338879,7.446739715699,3.645106950514));
#31447=CARTESIAN_POINT('Ctrl Pts',(0.548636073621,7.449170852428,3.613674065384));
#31448=CARTESIAN_POINT('Ctrl Pts',(0.5467125597304,7.451439307202,3.583175808014));
#31449=CARTESIAN_POINT('Ctrl Pts',(0.5466997109569,7.452870733248,3.563181477118));
#31450=CARTESIAN_POINT('Ctrl Pts',(0.5469704737393,7.453532628332,3.553763299103));
#31451=CARTESIAN_POINT('',(0.517449769067295,7.45443539562573,3.56771964176174));
#31452=CARTESIAN_POINT('Origin',(0.5,6.956014615875,3.532051288651));
#31453=CARTESIAN_POINT('Origin',(1.00128615094072,6.93399420435526,3.53122260992015));
#31454=CARTESIAN_POINT('Origin',(1.02905179608584,7.43196778205744,3.56615971566351));
#31455=CARTESIAN_POINT('Origin',(0.5,-42.4,0.));
#31456=CARTESIAN_POINT('',(0.517453073023311,7.54185093199608,2.00135351550442));
#31457=CARTESIAN_POINT('Origin',(0.5174497483513,-42.4,0.));
#31458=CARTESIAN_POINT('',(0.0865761666724887,7.32353683798742,1.99264208718994));
#31459=CARTESIAN_POINT('Origin',(0.5,7.0425494055,1.981381677743));
#31460=CARTESIAN_POINT('Ctrl Pts',(1.76192394008012E-13,6.99871871675034,
2.87370766691651));
#31461=CARTESIAN_POINT('Ctrl Pts',(1.54231259874596E-8,7.01973080080283,
2.82882528737174));
#31462=CARTESIAN_POINT('Ctrl Pts',(0.00101186006621219,7.03995776878894,
2.78388483535249));
#31463=CARTESIAN_POINT('Ctrl Pts',(0.00280079850515474,7.05927952278183,
2.73936883200046));
#31464=CARTESIAN_POINT('Ctrl Pts',(0.00380243770965784,7.07009790863444,
2.71444400886818));
#31465=CARTESIAN_POINT('Ctrl Pts',(0.00504780239427035,7.08063350065316,
2.68965236124658));
#31466=CARTESIAN_POINT('Ctrl Pts',(0.00649712134266744,7.09087208606895,
2.66507931910599));
#31467=CARTESIAN_POINT('Ctrl Pts',(0.00834719043383405,7.10394173539352,
2.63371160271029));
#31468=CARTESIAN_POINT('Ctrl Pts',(0.0105243960090612,7.11652241623467,
2.60269882830759));
#31469=CARTESIAN_POINT('Ctrl Pts',(0.0130034531449881,7.12880850553544,
2.57159451211062));
#31470=CARTESIAN_POINT('Ctrl Pts',(0.0155308113112305,7.14133397244602,
2.53988417094641));
#31471=CARTESIAN_POINT('Ctrl Pts',(0.0183721278706122,7.15355382103671,
2.50807870852747));
#31472=CARTESIAN_POINT('Ctrl Pts',(0.0215529360858484,7.16566375687849,
2.47570186213225));
#31473=CARTESIAN_POINT('Ctrl Pts',(0.0220616550255212,7.16760054567682,
2.47052370807403));
#31474=CARTESIAN_POINT('Ctrl Pts',(0.0225791610344311,7.16953449172451,
2.4653309317779));
#31475=CARTESIAN_POINT('Ctrl Pts',(0.0231056752009869,7.17146635677458,
2.46012157690981));
#31476=CARTESIAN_POINT('Ctrl Pts',(0.0275243378057489,7.18767913963284,
2.41640313016578));
#31477=CARTESIAN_POINT('Ctrl Pts',(0.0325718997016025,7.20374050194306,
2.37151833744122));
#31478=CARTESIAN_POINT('Ctrl Pts',(0.0383080237529643,7.21973440599729,
2.32497070432694));
#31479=CARTESIAN_POINT('Ctrl Pts',(0.0417209920364785,7.22925070773307,
2.29727506977142));
#31480=CARTESIAN_POINT('Ctrl Pts',(0.0453785461739025,7.23874266445839,
2.2689906890865));
#31481=CARTESIAN_POINT('Ctrl Pts',(0.0493002060250779,7.24822255917105,
2.24001235735313));
#31482=CARTESIAN_POINT('Ctrl Pts',(0.057002047233522,7.26684035023923,2.18310112130363));
#31483=CARTESIAN_POINT('Ctrl Pts',(0.0657293147569602,7.2854118098693,2.12351422610049));
#31484=CARTESIAN_POINT('Ctrl Pts',(0.0754853867527238,7.30367502560143,
2.06149859167507));
#31485=CARTESIAN_POINT('Ctrl Pts',(0.0790459994374604,7.31034043742169,
2.0388651327704));
#31486=CARTESIAN_POINT('Ctrl Pts',(0.0827431515438966,7.31696481318815,
2.01590821646725));
#31487=CARTESIAN_POINT('Ctrl Pts',(0.0865752842352255,7.32353562251123,
1.99264001890475));
#31488=CARTESIAN_POINT('Ctrl Pts',(-0.001081260139012,7.014309618948,2.906543661707));
#31489=CARTESIAN_POINT('Ctrl Pts',(-0.001018369255986,7.016400799091,2.902147314851));
#31490=CARTESIAN_POINT('Ctrl Pts',(0.0001871679450522,7.050992423812,2.829131820991));
#31491=CARTESIAN_POINT('Ctrl Pts',(0.007507857493721,7.113697217666,2.687558940315));
#31492=CARTESIAN_POINT('Ctrl Pts',(0.02870561913676,7.197032885506,2.474508650036));
#31493=CARTESIAN_POINT('Ctrl Pts',(0.05928519434814,7.274597632677,2.249119982873));
#31494=CARTESIAN_POINT('Ctrl Pts',(0.08618036230883,7.322967042458,2.086634502438));
#31495=CARTESIAN_POINT('Ctrl Pts',(0.1018793569146,7.347090408829,1.998560749934));
#31496=CARTESIAN_POINT('Ctrl Pts',(0.1027383636877,7.348399198641,1.993759888543));
#31497=CARTESIAN_POINT('Ctrl Pts',(0.02046330720855,6.777047057716,2.691466056719));
#31498=CARTESIAN_POINT('Ctrl Pts',(0.01962993973341,6.778769180525,2.687387423694));
#31499=CARTESIAN_POINT('Ctrl Pts',(0.005955867276291,6.807367774017,2.619615027721));
#31500=CARTESIAN_POINT('Ctrl Pts',(-0.01530270840099,6.862722393628,2.487237441822));
#31501=CARTESIAN_POINT('Ctrl Pts',(-0.03473413003973,6.944167200619,2.285821170463));
#31502=CARTESIAN_POINT('Ctrl Pts',(-0.04384970159776,7.027302511007,2.070790001253));
#31503=CARTESIAN_POINT('Ctrl Pts',(-0.0427213547525,7.084289791949,1.914480858456));
#31504=CARTESIAN_POINT('Ctrl Pts',(-0.04008670908316,7.114174883662,1.829403670676));
#31505=CARTESIAN_POINT('Ctrl Pts',(-0.03993718883914,7.115800914289,1.824765062074));
#31506=CARTESIAN_POINT('Ctrl Pts',(-0.2045700640878,6.606399527962,2.53896888117));
#31507=CARTESIAN_POINT('Ctrl Pts',(-0.2060475584221,6.608724880767,2.535166077691));
#31508=CARTESIAN_POINT('Ctrl Pts',(-0.2303376413689,6.647382899417,2.471943726365));
#31509=CARTESIAN_POINT('Ctrl Pts',(-0.2695762730753,6.723518668901,2.347474954217));
#31510=CARTESIAN_POINT('Ctrl Pts',(-0.3093746426751,6.838297728139,2.155847204795));
#31511=CARTESIAN_POINT('Ctrl Pts',(-0.3336343557535,6.95779484596,1.949271087601));
#31512=CARTESIAN_POINT('Ctrl Pts',(-0.3389528302416,7.041205966119,1.797815533392));
#31513=CARTESIAN_POINT('Ctrl Pts',(-0.3385904718372,7.085346251581,1.715024763658));
#31514=CARTESIAN_POINT('Ctrl Pts',(-0.3385612404185,7.087749102285,1.710509733302));
#31515=CARTESIAN_POINT('Ctrl Pts',(-0.5251165549145,6.61692265344,2.551423432733));
#31516=CARTESIAN_POINT('Ctrl Pts',(-0.526553642486,6.620418575498,2.547669410243));
#31517=CARTESIAN_POINT('Ctrl Pts',(-0.5500696128295,6.678435587297,2.485249607032));
#31518=CARTESIAN_POINT('Ctrl Pts',(-0.5846190863906,6.789533452527,2.362093983857));
#31519=CARTESIAN_POINT('Ctrl Pts',(-0.6108498439799,6.950494605875,2.171838228225));
#31520=CARTESIAN_POINT('Ctrl Pts',(-0.6155364367152,7.112735107433,1.966138843811));
#31521=CARTESIAN_POINT('Ctrl Pts',(-0.6036539839724,7.222637721349,1.814955916913));
#31522=CARTESIAN_POINT('Ctrl Pts',(-0.5932464655588,7.279957162664,1.732206546957));
#31523=CARTESIAN_POINT('Ctrl Pts',(-0.5926675754179,7.283074933677,1.727693462271));
#31524=CARTESIAN_POINT('Origin',(-0.3268616990873,7.604510051501,2.00392196632));
#31525=CARTESIAN_POINT('Origin',(-0.4999999999811,6.998719488534,2.873707297836));
#31526=CARTESIAN_POINT('Origin',(-0.5,3.8,0.));
#31527=CARTESIAN_POINT('',(-0.0201845395642384,5.74664288092434,3.67572020421874));
#31528=CARTESIAN_POINT('Ctrl Pts',(1.00945995400332E-15,6.252471626846,
3.532050807569));
#31529=CARTESIAN_POINT('Ctrl Pts',(1.06255127647422E-8,6.22355721500666,
3.54358362457381));
#31530=CARTESIAN_POINT('Ctrl Pts',(-0.000148869025013445,6.19495270787919,
3.5545016156147));
#31531=CARTESIAN_POINT('Ctrl Pts',(-0.000440295003910586,6.16703450720138,
3.56471173966722));
#31532=CARTESIAN_POINT('Ctrl Pts',(-0.000483686983627105,6.16287761630882,
3.56623197989243));
#31533=CARTESIAN_POINT('Ctrl Pts',(-0.000530204467916582,6.15873593010086,
3.56773661403369));
#31534=CARTESIAN_POINT('Ctrl Pts',(-0.000579789846082578,6.15461067703008,
3.56922542745825));
#31535=CARTESIAN_POINT('Ctrl Pts',(-0.000834392425583689,6.1334290280892,
3.57686993380889));
#31536=CARTESIAN_POINT('Ctrl Pts',(-0.00116909302387783,6.11268021448515,
3.58408901216498));
#31537=CARTESIAN_POINT('Ctrl Pts',(-0.0015949163214279,6.09188868636396,
3.59105101267837));
#31538=CARTESIAN_POINT('Ctrl Pts',(-0.00180900395429268,6.08143550293149,
3.59455123969387));
#31539=CARTESIAN_POINT('Ctrl Pts',(-0.00204636565207327,6.07097134948497,
3.59798577949579));
#31540=CARTESIAN_POINT('Ctrl Pts',(-0.002310032817556,6.06043519420868,
3.60137127125052));
#31541=CARTESIAN_POINT('Ctrl Pts',(-0.00286123018430172,6.03840931535766,
3.6084486566236));
#31542=CARTESIAN_POINT('Ctrl Pts',(-0.00352621841082366,6.01607131827214,
3.61531684209279));
#31543=CARTESIAN_POINT('Ctrl Pts',(-0.00434184921916814,5.99321851908052,
3.62196888132449));
#31544=CARTESIAN_POINT('Ctrl Pts',(-0.00469241156114277,5.98339626773429,
3.6248279622078));
#31545=CARTESIAN_POINT('Ctrl Pts',(-0.0050709858485351,5.97347906253195,
3.62764657225949));
#31546=CARTESIAN_POINT('Ctrl Pts',(-0.00548143949275076,5.96345175192577,
3.63042137614233));
#31547=CARTESIAN_POINT('Ctrl Pts',(-0.00627128196887642,5.94415603863468,
3.63576097538934));
#31548=CARTESIAN_POINT('Ctrl Pts',(-0.00717855499112012,5.92445507963207,
3.64093636106214));
#31549=CARTESIAN_POINT('Ctrl Pts',(-0.00824695910249482,5.9042812924823,
3.6458748404254));
#31550=CARTESIAN_POINT('Ctrl Pts',(-0.00902554440236525,5.88957991315374,
3.64947369164192));
#31551=CARTESIAN_POINT('Ctrl Pts',(-0.00988991053435746,5.874627728668,
3.65294614153715));
#31552=CARTESIAN_POINT('Ctrl Pts',(-0.0108620715118211,5.85940771717124,
3.6562497499432));
#31553=CARTESIAN_POINT('Ctrl Pts',(-0.0108621699993018,5.8594061752655,
3.65625008462447));
#31554=CARTESIAN_POINT('Ctrl Pts',(-0.010862268487912,5.85940463335719,
3.6562504193038));
#31555=CARTESIAN_POINT('Ctrl Pts',(-0.0108623669776518,5.85940309144632,
3.65625075398118));
#31556=CARTESIAN_POINT('Ctrl Pts',(-0.0118020552639595,5.84469175611481,
3.65944390298656));
#31557=CARTESIAN_POINT('Ctrl Pts',(-0.012843753824908,5.82974410458742,
3.66246313874807));
#31558=CARTESIAN_POINT('Ctrl Pts',(-0.0140227868938516,5.81454018579014,
3.66525725177376));
#31559=CARTESIAN_POINT('Ctrl Pts',(-0.0150765914048981,5.8009511197697,
3.66775459386569));
#31560=CARTESIAN_POINT('Ctrl Pts',(-0.0162400356832888,5.78715707091662,
3.67007226537261));
#31561=CARTESIAN_POINT('Ctrl Pts',(-0.0175467950230611,5.7731696367615,
3.67214302747442));
#31562=CARTESIAN_POINT('Ctrl Pts',(-0.0183660613490072,5.76440028387387,
3.67344128156561));
#31563=CARTESIAN_POINT('Ctrl Pts',(-0.0192418228542866,5.75555543595967,
3.67464188759342));
#31564=CARTESIAN_POINT('Ctrl Pts',(-0.0201846418813895,5.74664479462204,
3.67572037342067));
#31565=CARTESIAN_POINT('Ctrl Pts',(-0.0201846820169889,5.74664441529799,
3.67572041933158));
#31566=CARTESIAN_POINT('Ctrl Pts',(-0.0201847221527103,5.74664403597382,
3.67572046524226));
#31567=CARTESIAN_POINT('Ctrl Pts',(-0.0201847622885535,5.74664365664953,
3.67572051115272));
#31568=CARTESIAN_POINT('Origin',(-0.5,3.8,0.));
#31569=CARTESIAN_POINT('Origin',(-0.5,5.812461179705,3.800000000024));
#31570=CARTESIAN_POINT('Ctrl Pts',(0.1458532199875,6.271988053784,4.052080103981));
#31571=CARTESIAN_POINT('Ctrl Pts',(0.1469209552276,6.265500255559,4.053835336582));
#31572=CARTESIAN_POINT('Ctrl Pts',(0.1548191992219,6.217130452916,4.066727704464));
#31573=CARTESIAN_POINT('Ctrl Pts',(0.1686877140563,6.126928446731,4.08805599936));
#31574=CARTESIAN_POINT('Ctrl Pts',(0.1862467344624,5.996365514295,4.111423817831));
#31575=CARTESIAN_POINT('Ctrl Pts',(0.2017409989679,5.856602279246,4.127313273259));
#31576=CARTESIAN_POINT('Ctrl Pts',(0.214005833747,5.696109622742,4.13198287192));
#31577=CARTESIAN_POINT('Ctrl Pts',(0.2165291553049,5.564635500454,4.119507848871));
#31578=CARTESIAN_POINT('Ctrl Pts',(0.2121000073809,5.485266618107,4.101280410414));
#31579=CARTESIAN_POINT('Ctrl Pts',(0.2114977825543,5.476027053408,4.099020181562));
#31580=CARTESIAN_POINT('Ctrl Pts',(0.04343936334695,6.270350607014,3.883896132752));
#31581=CARTESIAN_POINT('Ctrl Pts',(0.04416828941248,6.264404627156,3.88585256665));
#31582=CARTESIAN_POINT('Ctrl Pts',(0.04955358456158,6.220092655311,3.900265951108));
#31583=CARTESIAN_POINT('Ctrl Pts',(0.05891618512559,6.137723881081,3.924730474888));
#31584=CARTESIAN_POINT('Ctrl Pts',(0.07051173903919,6.01940133794,3.953533205108));
#31585=CARTESIAN_POINT('Ctrl Pts',(0.08040336843717,5.894063634032,3.976422191027));
#31586=CARTESIAN_POINT('Ctrl Pts',(0.08764358238867,5.752421718795,3.991109125861));
#31587=CARTESIAN_POINT('Ctrl Pts',(0.08809976070129,5.639482864577,3.989538930058));
#31588=CARTESIAN_POINT('Ctrl Pts',(0.08415878673266,5.573169980138,3.980095150633));
#31589=CARTESIAN_POINT('Ctrl Pts',(0.08363892228445,5.565474898,3.978885877421));
#31590=CARTESIAN_POINT('Ctrl Pts',(-0.006377890669527,6.268771084875,3.693389188242));
#31591=CARTESIAN_POINT('Ctrl Pts',(-0.00603236671339,6.263346825442,3.695441735005));
#31592=CARTESIAN_POINT('Ctrl Pts',(-0.003495091272066,6.222949053301,3.710593058645));
#31593=CARTESIAN_POINT('Ctrl Pts',(0.0007007410215009,6.148232643904,3.736740844206));
#31594=CARTESIAN_POINT('Ctrl Pts',(0.005295480516823,6.042135280344,3.768916440852));
#31595=CARTESIAN_POINT('Ctrl Pts',(0.008404965977148,5.931514095113,3.796677725173));
#31596=CARTESIAN_POINT('Ctrl Pts',(0.009229009165082,5.809512435811,3.819120678812));
#31597=CARTESIAN_POINT('Ctrl Pts',(0.006530259998911,5.716291958244,3.826913774935));
#31598=CARTESIAN_POINT('Ctrl Pts',(0.002550540157001,5.664026167199,3.825603599923));
#31599=CARTESIAN_POINT('Ctrl Pts',(0.002053792328862,5.657994551734,3.825373242286));
#31600=CARTESIAN_POINT('Ctrl Pts',(0.0005956750778858,6.267382470588,3.496598442174));
#31601=CARTESIAN_POINT('Ctrl Pts',(0.000545483402435,6.262415908922,3.498633921431));
#31602=CARTESIAN_POINT('Ctrl Pts',(0.0001394489138727,6.225459160862,3.513677978239));
#31603=CARTESIAN_POINT('Ctrl Pts',(-0.001057340209199,6.157569980829,3.539914341205));
#31604=CARTESIAN_POINT('Ctrl Pts',(-0.003911350084333,6.062653324111,3.573116790386));
#31605=CARTESIAN_POINT('Ctrl Pts',(-0.008192514736,5.965800631096,3.603212932189));
#31606=CARTESIAN_POINT('Ctrl Pts',(-0.0146360016265,5.862575188833,3.630497592084));
#31607=CARTESIAN_POINT('Ctrl Pts',(-0.0213118426677,5.788596065785,3.645324129995));
#31608=CARTESIAN_POINT('Ctrl Pts',(-0.02585396611666,5.750185809919,3.650812719882));
#31609=CARTESIAN_POINT('Ctrl Pts',(-0.02638878731888,5.745796594557,3.651406820841));
#31610=CARTESIAN_POINT('Origin',(1.,6.252471673428,3.532050807569));
#31611=CARTESIAN_POINT('Origin',(0.9394500501458,5.615008433104,3.427175219049));
#31612=CARTESIAN_POINT('Ctrl Pts',(0.09069279366311,5.616670622145,3.956220996979));
#31613=CARTESIAN_POINT('Ctrl Pts',(0.08945616748986,5.611892456011,3.954079097617));
#31614=CARTESIAN_POINT('Ctrl Pts',(0.08238462062046,5.583998454902,3.941830819151));
#31615=CARTESIAN_POINT('Ctrl Pts',(0.06901185007231,5.525746410592,3.918668501123));
#31616=CARTESIAN_POINT('Ctrl Pts',(0.0509683933199,5.437857521209,3.887416317284));
#31617=CARTESIAN_POINT('Ctrl Pts',(0.03265833413454,5.340814192582,3.855702364485));
#31618=CARTESIAN_POINT('Ctrl Pts',(0.0195624461478,5.266338417057,3.833019621122));
#31619=CARTESIAN_POINT('Ctrl Pts',(0.01244523448206,5.224602654389,3.820692248908));
#31620=CARTESIAN_POINT('Ctrl Pts',(0.01153465633603,5.219243031459,3.819115081295));
#31621=CARTESIAN_POINT('Ctrl Pts',(0.03425063267428,5.671857593246,3.865525883381));
#31622=CARTESIAN_POINT('Ctrl Pts',(0.03286492200821,5.666497275129,3.863125762102));
#31623=CARTESIAN_POINT('Ctrl Pts',(0.02500759929367,5.635488104076,3.849516479949));
#31624=CARTESIAN_POINT('Ctrl Pts',(0.01074391216856,5.57326828928,3.82481104915));
#31625=CARTESIAN_POINT('Ctrl Pts',(-0.008050805571124,5.481693915529,3.792257643109));
#31626=CARTESIAN_POINT('Ctrl Pts',(-0.02689492653263,5.381798763955,3.759618668181));
#31627=CARTESIAN_POINT('Ctrl Pts',(-0.04025534178605,5.305812877369,3.73647775015));
#31628=CARTESIAN_POINT('Ctrl Pts',(-0.04749710773029,5.263345244532,3.723934643602));
#31629=CARTESIAN_POINT('Ctrl Pts',(-0.04842335115087,5.257893246949,3.722330342938));
#31630=CARTESIAN_POINT('Ctrl Pts',(-0.002995698117571,5.726448488071,3.765079625067));
#31631=CARTESIAN_POINT('Ctrl Pts',(-0.004528883010469,5.720512305815,3.762424070936));
#31632=CARTESIAN_POINT('Ctrl Pts',(-0.01316349438033,5.68642161187,3.747468485341));
#31633=CARTESIAN_POINT('Ctrl Pts',(-0.02830847524902,5.620276882606,3.721236608974));
#31634=CARTESIAN_POINT('Ctrl Pts',(-0.04784633958708,5.525056831524,3.687396035277));
#31635=CARTESIAN_POINT('Ctrl Pts',(-0.06721875390343,5.422340659634,3.653842029412));
#31636=CARTESIAN_POINT('Ctrl Pts',(-0.08084083925938,5.344860972747,3.630247885476));
#31637=CARTESIAN_POINT('Ctrl Pts',(-0.08820581416463,5.301669374694,3.617491374745));
#31638=CARTESIAN_POINT('Ctrl Pts',(-0.08914755365818,5.2961260002,3.615860234094));
#31639=CARTESIAN_POINT('Ctrl Pts',(-0.01985090485308,5.778691398179,3.65810570186));
#31640=CARTESIAN_POINT('Ctrl Pts',(-0.02152522102488,5.772204120019,3.655205701185));
#31641=CARTESIAN_POINT('Ctrl Pts',(-0.03090368943386,5.735164441195,3.638961717408));
#31642=CARTESIAN_POINT('Ctrl Pts',(-0.04689205909801,5.665263610215,3.611269048736));
#31643=CARTESIAN_POINT('Ctrl Pts',(-0.06714110689197,5.566554684409,3.576196669184));
#31644=CARTESIAN_POINT('Ctrl Pts',(-0.08701909236977,5.461138825856,3.541766988369));
#31645=CARTESIAN_POINT('Ctrl Pts',(-0.1008915932553,5.382229587848,3.517739112028));
#31646=CARTESIAN_POINT('Ctrl Pts',(-0.108374477833,5.338345162724,3.504778375744));
#31647=CARTESIAN_POINT('Ctrl Pts',(-0.1093310469044,5.33271434149,3.50312154951));
#31648=CARTESIAN_POINT('Ctrl Pts',(-0.0201840365334425,5.74664296949069,
3.67572052170447));
#31649=CARTESIAN_POINT('Ctrl Pts',(-0.0210927252446989,5.7269006225596,
3.68266762453094));
#31650=CARTESIAN_POINT('Ctrl Pts',(-0.0217041190570385,5.70714963688255,
3.68923829806003));
#31651=CARTESIAN_POINT('Ctrl Pts',(-0.0220696690856361,5.68759667513464,
3.69543690080271));
#31652=CARTESIAN_POINT('Ctrl Pts',(-0.0224351127454171,5.66804940296473,
3.70163369985783));
#31653=CARTESIAN_POINT('Ctrl Pts',(-0.0225555467297995,5.64870011852324,
3.70745776399795));
#31654=CARTESIAN_POINT('Ctrl Pts',(-0.0224800830796922,5.62980882412369,
3.71292583377142));
#31655=CARTESIAN_POINT('Ctrl Pts',(-0.0224679836683386,5.62677990170056,
3.71380255289918));
#31656=CARTESIAN_POINT('Ctrl Pts',(-0.0224508333255254,5.62376285473207,
3.71467015812384));
#31657=CARTESIAN_POINT('Ctrl Pts',(-0.0224288160121262,5.62075886263511,
3.71552876206813));
#31658=CARTESIAN_POINT('Ctrl Pts',(-0.0224288112348433,5.6207582108335,
3.7155289483667));
#31659=CARTESIAN_POINT('Ctrl Pts',(-0.0224288064573312,5.62075755903251,
3.71552913466485));
#31660=CARTESIAN_POINT('Ctrl Pts',(-0.02242880167959,5.62075690723214,3.71552932096257));
#31661=CARTESIAN_POINT('Ctrl Pts',(-0.0223037157913754,5.60369214283302,
3.72040677554117));
#31662=CARTESIAN_POINT('Ctrl Pts',(-0.0220235154826046,5.58704134367518,
3.72499898065695));
#31663=CARTESIAN_POINT('Ctrl Pts',(-0.0216232495575363,5.57048317754424,
3.72940007283941));
#31664=CARTESIAN_POINT('Ctrl Pts',(-0.021196012066042,5.55280925398874,
3.73409772873791));
#31665=CARTESIAN_POINT('Ctrl Pts',(-0.0206318069207095,5.53524104924983,
3.73857826340128));
#31666=CARTESIAN_POINT('Ctrl Pts',(-0.0199233159681402,5.51741218968596,
3.74297341795032));
#31667=CARTESIAN_POINT('Ctrl Pts',(-0.0197209598352948,5.5123199876454,
3.74422874305303));
#31668=CARTESIAN_POINT('Ctrl Pts',(-0.0195065456981628,5.50720666188784,
3.74547717429369));
#31669=CARTESIAN_POINT('Ctrl Pts',(-0.019279233338892,5.50206401593398,
3.74672192155617));
#31670=CARTESIAN_POINT('Ctrl Pts',(-0.0192792117831918,5.50206352826435,
3.74672203959374));
#31671=CARTESIAN_POINT('Ctrl Pts',(-0.0192791902273797,5.50206304059445,
3.74672215763127));
#31672=CARTESIAN_POINT('Ctrl Pts',(-0.0192791686714558,5.50206255292428,
3.74672227566876));
#31673=CARTESIAN_POINT('Ctrl Pts',(-0.017975161601807,5.47256136556275,
3.7538628518065));
#31674=CARTESIAN_POINT('Ctrl Pts',(-0.0162581453164372,5.44206985804176,
3.76084820516659));
#31675=CARTESIAN_POINT('Ctrl Pts',(-0.0141475466666794,5.41086175160518,
3.76759619439652));
#31676=CARTESIAN_POINT('Ctrl Pts',(-0.0133952540300333,5.39973806938421,
3.77000141843588));
#31677=CARTESIAN_POINT('Ctrl Pts',(-0.0125933460890804,5.38852361999037,
3.77237640057866));
#31678=CARTESIAN_POINT('Ctrl Pts',(-0.0117438815315688,5.37723190413217,
3.77471733200074));
#31679=CARTESIAN_POINT('Ctrl Pts',(-0.00936709712271081,5.34563791476123,
3.78126721010574));
#31680=CARTESIAN_POINT('Ctrl Pts',(-0.00661723154578303,5.31343729109814,
3.78755503811181));
#31681=CARTESIAN_POINT('Ctrl Pts',(-0.00350446402653477,5.28057655596057,
3.79358521521042));
#31682=CARTESIAN_POINT('Ctrl Pts',(-0.00238348478125948,5.26874264872339,
3.79575682080932));
#31683=CARTESIAN_POINT('Ctrl Pts',(-0.00121532087410187,5.25682357467516,
3.79789500125968));
#31684=CARTESIAN_POINT('Ctrl Pts',(-1.96584511304227E-8,5.24481852186864,
3.79999996595058));
#31685=CARTESIAN_POINT('Ctrl Pts',(0.01313183742357,5.24106019073,3.823805869142));
#31686=CARTESIAN_POINT('Ctrl Pts',(0.01303186504026,5.246042423464,3.82385436109));
#31687=CARTESIAN_POINT('Ctrl Pts',(0.01123027883061,5.335368565326,3.82471367541));
#31688=CARTESIAN_POINT('Ctrl Pts',(0.007608839441613,5.499707692812,3.825952350517));
#31689=CARTESIAN_POINT('Ctrl Pts',(0.002704317645799,5.694405545869,3.826393794893));
#31690=CARTESIAN_POINT('Ctrl Pts',(-0.0002703855975803,5.80461369123,3.826069286647));
#31691=CARTESIAN_POINT('Ctrl Pts',(-0.001263515685967,5.840827121397,3.825885856397));
#31692=CARTESIAN_POINT('Ctrl Pts',(-0.1220155422729,5.119490788538,3.559282264932));
#31693=CARTESIAN_POINT('Ctrl Pts',(-0.1210052566975,5.124318427941,3.558834796486));
#31694=CARTESIAN_POINT('Ctrl Pts',(-0.1028036746347,5.210842870579,3.550915651627));
#31695=CARTESIAN_POINT('Ctrl Pts',(-0.06637047516781,5.369103572629,3.539852558725));
#31696=CARTESIAN_POINT('Ctrl Pts',(-0.01740572866676,5.553685032541,3.537170858724));
#31697=CARTESIAN_POINT('Ctrl Pts',(0.0121187820176,5.65630378412,3.541453508646));
#31698=CARTESIAN_POINT('Ctrl Pts',(0.02195442675914,5.689769064298,3.543633877626));
#31699=CARTESIAN_POINT('Ctrl Pts',(-0.4243708118278,5.033379764573,3.494607553578));
#31700=CARTESIAN_POINT('Ctrl Pts',(-0.4230739478696,5.038097901175,3.492966852937));
#31701=CARTESIAN_POINT('Ctrl Pts',(-0.3995937923544,5.122637821518,3.463646745943));
#31702=CARTESIAN_POINT('Ctrl Pts',(-0.3487237350521,5.276593004014,3.413015804354));
#31703=CARTESIAN_POINT('Ctrl Pts',(-0.2708767291411,5.454008738366,3.365007313026));
#31704=CARTESIAN_POINT('Ctrl Pts',(-0.2195329377535,5.551251709049,3.345376679572));
#31705=CARTESIAN_POINT('Ctrl Pts',(-0.2018836868802,5.582770397361,3.339993364003));
#31706=CARTESIAN_POINT('Ctrl Pts',(-0.690961983047,5.040533704331,3.673198060413));
#31707=CARTESIAN_POINT('Ctrl Pts',(-0.6903946011995,5.045260938217,3.670467876084));
#31708=CARTESIAN_POINT('Ctrl Pts',(-0.6799039890485,5.12996572889,3.621490833281));
#31709=CARTESIAN_POINT('Ctrl Pts',(-0.649906360366,5.284278605745,3.530587976371));
#31710=CARTESIAN_POINT('Ctrl Pts',(-0.587552850239,5.46228965492,3.42547705607));
#31711=CARTESIAN_POINT('Ctrl Pts',(-0.5397170591493,5.559979235235,3.369465755669));
#31712=CARTESIAN_POINT('Ctrl Pts',(-0.5225146677869,5.591659642689,3.351668795617));
#31713=CARTESIAN_POINT('Origin',(-0.4330128001874,5.244818804908,4.049999829751));
#31714=CARTESIAN_POINT('Ctrl Pts',(0.1654598431239,3.783166653544,4.090816155837));
#31715=CARTESIAN_POINT('Ctrl Pts',(0.1654730736086,3.788777525565,4.090839257161));
#31716=CARTESIAN_POINT('Ctrl Pts',(0.1656678333893,3.954021206316,4.091179620988));
#31717=CARTESIAN_POINT('Ctrl Pts',(0.1547815560753,4.279983877015,4.072101699741));
#31718=CARTESIAN_POINT('Ctrl Pts',(0.1051279211205,4.770778970143,3.985157894746));
#31719=CARTESIAN_POINT('Ctrl Pts',(0.04760955067503,5.097085532837,3.884627779379));
#31720=CARTESIAN_POINT('Ctrl Pts',(0.01060629140589,5.266200668492,3.820069159091));
#31721=CARTESIAN_POINT('Ctrl Pts',(0.009485886370904,5.271290271532,3.818114554136));
#31722=CARTESIAN_POINT('Ctrl Pts',(0.07652291896167,3.784112020329,3.897696692716));
#31723=CARTESIAN_POINT('Ctrl Pts',(0.07653599330915,3.789407784645,3.897718314989));
#31724=CARTESIAN_POINT('Ctrl Pts',(0.0767284685246,3.945371305455,3.898036864973));
#31725=CARTESIAN_POINT('Ctrl Pts',(0.06596551784964,4.253028048728,3.880183155471));
#31726=CARTESIAN_POINT('Ctrl Pts',(0.0168611100287,4.716461525162,3.798792241893));
#31727=CARTESIAN_POINT('Ctrl Pts',(-0.04005056496638,5.02485756519,3.704621421695));
#31728=CARTESIAN_POINT('Ctrl Pts',(-0.07668074739283,5.184805550002,3.644109787065));
#31729=CARTESIAN_POINT('Ctrl Pts',(-0.07778986614245,5.189619370843,3.642277679814));
#31730=CARTESIAN_POINT('Ctrl Pts',(-0.1058150099763,3.784941987692,3.788344136719));
#31731=CARTESIAN_POINT('Ctrl Pts',(-0.1058022557404,3.789961110452,3.788364161886));
#31732=CARTESIAN_POINT('Ctrl Pts',(-0.1056144643264,3.937777260311,3.788659124856));
#31733=CARTESIAN_POINT('Ctrl Pts',(-0.1161245714929,4.22936306796,3.772131316596));
#31734=CARTESIAN_POINT('Ctrl Pts',(-0.1641029572589,4.669106290867,3.69671684643));
#31735=CARTESIAN_POINT('Ctrl Pts',(-0.2197707890137,4.962460172974,3.60930175649));
#31736=CARTESIAN_POINT('Ctrl Pts',(-0.2556360916169,5.114903105384,3.553035639076));
#31737=CARTESIAN_POINT('Ctrl Pts',(-0.2567220712945,5.119491329578,3.551331993798));
#31738=CARTESIAN_POINT('Ctrl Pts',(-0.3180638821296,3.785367561021,3.800835044669));
#31739=CARTESIAN_POINT('Ctrl Pts',(-0.3180515005168,3.790244834956,3.800853910787));
#31740=CARTESIAN_POINT('Ctrl Pts',(-0.3178691612411,3.933883317182,3.801131726569));
#31741=CARTESIAN_POINT('Ctrl Pts',(-0.3280849481318,4.217229080328,3.785569830272));
#31742=CARTESIAN_POINT('Ctrl Pts',(-0.3747525977687,4.645202358463,3.714474358092));
#31743=CARTESIAN_POINT('Ctrl Pts',(-0.4289725446736,4.931620126345,3.631859088419));
#31744=CARTESIAN_POINT('Ctrl Pts',(-0.4639474956053,5.080833363824,3.578558730809));
#31745=CARTESIAN_POINT('Ctrl Pts',(-0.4650065404483,5.085324729669,3.576944781319));
#31746=CARTESIAN_POINT('Origin',(-0.2886751345948,3.799999998586,4.3));
#31747=CARTESIAN_POINT('Ctrl Pts',(0.009474644443544,2.328658952906,3.818094956611));
#31748=CARTESIAN_POINT('Ctrl Pts',(0.0105988341721,2.333765482268,3.820056164338));
#31749=CARTESIAN_POINT('Ctrl Pts',(0.04385068457141,2.485729493349,3.878069544614));
#31750=CARTESIAN_POINT('Ctrl Pts',(0.09915489585668,2.792156941505,3.974710259671));
#31751=CARTESIAN_POINT('Ctrl Pts',(0.1527218994168,3.281111771178,4.068490389354));
#31752=CARTESIAN_POINT('Ctrl Pts',(0.1656911157868,3.626085089004,4.091220199701));
#31753=CARTESIAN_POINT('Ctrl Pts',(0.1654730928139,3.811221437351,4.090839298692));
#31754=CARTESIAN_POINT('Ctrl Pts',(0.1654598554814,3.816831728666,4.090816203645));
#31755=CARTESIAN_POINT('Ctrl Pts',(-0.07780099826889,2.410332609439,3.642259301122));
#31756=CARTESIAN_POINT('Ctrl Pts',(-0.07668813260086,2.415162439761,3.644097597749));
#31757=CARTESIAN_POINT('Ctrl Pts',(-0.04377154882854,2.558889003431,3.698474311926));
#31758=CARTESIAN_POINT('Ctrl Pts',(0.01095237427205,2.848518182611,3.789008170026));
#31759=CARTESIAN_POINT('Ctrl Pts',(0.06392943237314,3.310252236621,3.87680411232));
#31760=CARTESIAN_POINT('Ctrl Pts',(0.07675144997308,3.635852231929,3.89807481882));
#31761=CARTESIAN_POINT('Ctrl Pts',(0.07653600950347,3.810591236453,3.897718345495));
#31762=CARTESIAN_POINT('Ctrl Pts',(0.07652293033348,3.815886452588,3.897696729126));
#31763=CARTESIAN_POINT('Ctrl Pts',(-0.2567329809627,2.48046290541,3.551314900382));
#31764=CARTESIAN_POINT('Ctrl Pts',(-0.2556433318135,2.485066389654,3.553024302123));
#31765=CARTESIAN_POINT('Ctrl Pts',(-0.2234141096054,2.622049040122,3.60358597455));
#31766=CARTESIAN_POINT('Ctrl Pts',(-0.1698798897507,2.897605700672,3.68764162277));
#31767=CARTESIAN_POINT('Ctrl Pts',(-0.1181123341796,3.335834773715,3.769004622719));
#31768=CARTESIAN_POINT('Ctrl Pts',(-0.1055921025872,3.644427145636,3.788694227807));
#31769=CARTESIAN_POINT('Ctrl Pts',(-0.1058022484245,3.810037961682,3.788364190593));
#31770=CARTESIAN_POINT('Ctrl Pts',(-0.1058150033307,3.8150565647,3.788344170967));
#31771=CARTESIAN_POINT('Ctrl Pts',(-0.4650171874696,2.514630471845,3.576928594623));
#31772=CARTESIAN_POINT('Ctrl Pts',(-0.4639545633057,2.519136776674,3.57854799889));
#31773=CARTESIAN_POINT('Ctrl Pts',(-0.4325254583033,2.653217278719,3.626444651451));
#31774=CARTESIAN_POINT('Ctrl Pts',(-0.3803761020868,2.922327221957,3.705906449542));
#31775=CARTESIAN_POINT('Ctrl Pts',(-0.3300164573371,3.348951543072,3.782627702705));
#31776=CARTESIAN_POINT('Ctrl Pts',(-0.3178475171024,3.648824045183,3.801164748326));
#31777=CARTESIAN_POINT('Ctrl Pts',(-0.3180514997693,3.809754263313,3.800853950596));
#31778=CARTESIAN_POINT('Ctrl Pts',(-0.318063877219,3.814631031964,3.800835089794));
#31779=CARTESIAN_POINT('Origin',(-0.4330127019009,2.355181672278,4.049999999985));
#31780=CARTESIAN_POINT('Ctrl Pts',(-0.01268225231146,1.827199165611,3.694029057209));
#31781=CARTESIAN_POINT('Ctrl Pts',(-0.01301759300711,1.860931244349,3.712030310352));
#31782=CARTESIAN_POINT('Ctrl Pts',(-0.01039416625468,1.95192169302,3.759169815227));
#31783=CARTESIAN_POINT('Ctrl Pts',(0.007243775571969,2.110691864198,3.834329624173));
#31784=CARTESIAN_POINT('Ctrl Pts',(0.03200461518363,2.243916778438,3.889613928573));
#31785=CARTESIAN_POINT('Ctrl Pts',(0.04752295460543,2.315712820635,3.91708532505));
#31786=CARTESIAN_POINT('Ctrl Pts',(0.0486419497013,2.320840670637,3.919035840936));
#31787=CARTESIAN_POINT('Ctrl Pts',(-0.06997922130649,1.944219997842,3.474398904349));
#31788=CARTESIAN_POINT('Ctrl Pts',(-0.07032634590019,1.976515219533,3.491637536804));
#31789=CARTESIAN_POINT('Ctrl Pts',(-0.06761185180598,2.063452898229,3.53664207313));
#31790=CARTESIAN_POINT('Ctrl Pts',(-0.04957368891527,2.214589162901,3.607995942418));
#31791=CARTESIAN_POINT('Ctrl Pts',(-0.02442010395647,2.341021383202,3.6602310987));
#31792=CARTESIAN_POINT('Ctrl Pts',(-0.008697103908191,2.409075148295,3.686137285925));
#31793=CARTESIAN_POINT('Ctrl Pts',(-0.007563534861443,2.413935321588,3.687976404913));
#31794=CARTESIAN_POINT('Ctrl Pts',(-0.2743702035042,2.014941453006,3.338610219497));
#31795=CARTESIAN_POINT('Ctrl Pts',(-0.2747593638729,2.049740450048,3.357212410043));
#31796=CARTESIAN_POINT('Ctrl Pts',(-0.2717200123951,2.142267225392,3.404879810831));
#31797=CARTESIAN_POINT('Ctrl Pts',(-0.2522541723024,2.299455101574,3.47783355744));
#31798=CARTESIAN_POINT('Ctrl Pts',(-0.22569957768,2.428417376632,3.529601984769));
#31799=CARTESIAN_POINT('Ctrl Pts',(-0.2092465078358,2.497297199027,3.554946751002));
#31800=CARTESIAN_POINT('Ctrl Pts',(-0.2080609502775,2.502213777215,3.556744267749));
#31801=CARTESIAN_POINT('Ctrl Pts',(-0.5292956670928,2.005952905416,3.350813053175));
#31802=CARTESIAN_POINT('Ctrl Pts',(-0.5297372563374,2.046013462642,3.372260800848));
#31803=CARTESIAN_POINT('Ctrl Pts',(-0.5262927283777,2.151130768936,3.426130893777));
#31804=CARTESIAN_POINT('Ctrl Pts',(-0.5050462261996,2.325196838465,3.505334511686));
#31805=CARTESIAN_POINT('Ctrl Pts',(-0.4767442304242,2.464816654345,3.559439123932));
#31806=CARTESIAN_POINT('Ctrl Pts',(-0.4593805852738,2.538700617836,3.585491487078));
#31807=CARTESIAN_POINT('Ctrl Pts',(-0.4581301853469,2.543971035405,3.587336850206));
#31808=CARTESIAN_POINT('',(-0.020178900715945,1.85334863830895,3.67573612706027));
#31809=CARTESIAN_POINT('Ctrl Pts',(5.78773784938718E-13,2.355181672324,
3.80000000000086));
#31810=CARTESIAN_POINT('Ctrl Pts',(-0.00259348412084394,2.32958325346104,
3.79550811878464));
#31811=CARTESIAN_POINT('Ctrl Pts',(-0.0050129340853925,2.30398482576912,
3.79079385831531));
#31812=CARTESIAN_POINT('Ctrl Pts',(-0.00722157512980347,2.27856539847399,
3.78588019449874));
#31813=CARTESIAN_POINT('Ctrl Pts',(-0.0094302161742131,2.25314597117887,
3.78096653068217));
#31814=CARTESIAN_POINT('Ctrl Pts',(-0.0114322186707008,2.22790547510456,
3.77585564649884));
#31815=CARTESIAN_POINT('Ctrl Pts',(-0.0132303451805874,2.20242095353657,
3.77044240629286));
#31816=CARTESIAN_POINT('Ctrl Pts',(-0.0145671608308309,2.18347450728612,
3.76641793738809));
#31817=CARTESIAN_POINT('Ctrl Pts',(-0.0157899159720803,2.16439402966783,
3.76222640653729));
#31818=CARTESIAN_POINT('Ctrl Pts',(-0.0168856972943328,2.14510636267199,
3.75782462812579));
#31819=CARTESIAN_POINT('Ctrl Pts',(-0.0172638315745967,2.13845053825764,
3.75630565415014));
#31820=CARTESIAN_POINT('Ctrl Pts',(-0.0176267490905933,2.13177009729399,
3.75476161339509));
#31821=CARTESIAN_POINT('Ctrl Pts',(-0.0179734794456808,2.12506244269226,
3.75319088822452));
#31822=CARTESIAN_POINT('Ctrl Pts',(-0.0190646827361773,2.1039526244559,
3.74824762193864));
#31823=CARTESIAN_POINT('Ctrl Pts',(-0.0199991533623702,2.08257197318519,
3.74303980220404));
#31824=CARTESIAN_POINT('Ctrl Pts',(-0.020737879582049,2.06065772311987,
3.73745866791453));
#31825=CARTESIAN_POINT('Ctrl Pts',(-0.0209141010770433,2.05543012755698,
3.73612730075569));
#31826=CARTESIAN_POINT('Ctrl Pts',(-0.0210789980621449,2.05017229709023,
3.73477465577134));
#31827=CARTESIAN_POINT('Ctrl Pts',(-0.0212316696078731,2.04488092819401,
3.7333992003443));
#31828=CARTESIAN_POINT('Ctrl Pts',(-0.021644207299719,2.03058298484946,
3.72968254702556));
#31829=CARTESIAN_POINT('Ctrl Pts',(-0.0219699971594484,2.01604450125176,
3.72580198438638));
#31830=CARTESIAN_POINT('Ctrl Pts',(-0.0221928799302953,2.00089825894294,
3.72161269769981));
#31831=CARTESIAN_POINT('Ctrl Pts',(-0.0223982579968669,1.98694156794618,
3.71775242803099));
#31832=CARTESIAN_POINT('Ctrl Pts',(-0.0225164979983158,1.97246858060208,
3.7136298178958));
#31833=CARTESIAN_POINT('Ctrl Pts',(-0.0225031916269554,1.95721439476657,
3.70912669446936));
#31834=CARTESIAN_POINT('Ctrl Pts',(-0.0225017100281382,1.95551591641515,
3.70862529388752));
#31835=CARTESIAN_POINT('Ctrl Pts',(-0.0224985391601981,1.95380776921443,
3.70811923182651));
#31836=CARTESIAN_POINT('Ctrl Pts',(-0.0224936160594434,1.95209019693844,
3.70760844201206));
#31837=CARTESIAN_POINT('Ctrl Pts',(-0.0224399754837185,1.93337606324044,
3.70204303494726));
#31838=CARTESIAN_POINT('Ctrl Pts',(-0.022180408083899,1.91354025838126,
3.69591382635628));
#31839=CARTESIAN_POINT('Ctrl Pts',(-0.0216189713074668,1.89293208130006,
3.68916541028671));
#31840=CARTESIAN_POINT('Ctrl Pts',(-0.0212669316344575,1.88001006367398,
3.68493392726637));
#31841=CARTESIAN_POINT('Ctrl Pts',(-0.0207956678806571,1.86678504453139,
3.68045958413581));
#31842=CARTESIAN_POINT('Ctrl Pts',(-0.020176966977485,1.85334980564532,
3.67573540519852));
#31843=CARTESIAN_POINT('Origin',(-0.5,1.78753882025,3.8));
#31844=CARTESIAN_POINT('Ctrl Pts',(0.01155951010132,2.380682544795,3.819157949804));
#31845=CARTESIAN_POINT('Ctrl Pts',(0.01246241576851,2.375339654434,3.820721864307));
#31846=CARTESIAN_POINT('Ctrl Pts',(0.0169512535827,2.348900772593,3.828496902369));
#31847=CARTESIAN_POINT('Ctrl Pts',(0.02510386697286,2.301991385,3.842617643754));
#31848=CARTESIAN_POINT('Ctrl Pts',(0.03620327875676,2.240589380903,3.861842388624));
#31849=CARTESIAN_POINT('Ctrl Pts',(0.04760543423679,2.180147839132,3.881591501305));
#31850=CARTESIAN_POINT('Ctrl Pts',(0.05961053663961,2.119669925868,3.902384948596));
#31851=CARTESIAN_POINT('Ctrl Pts',(0.07279883802991,2.057561847955,3.925227756676));
#31852=CARTESIAN_POINT('Ctrl Pts',(0.08339615424009,2.012042225791,3.943582846774));
#31853=CARTESIAN_POINT('Ctrl Pts',(0.08936855627525,1.988452335483,3.953927350542));
#31854=CARTESIAN_POINT('Ctrl Pts',(0.09055372500124,1.983862542045,3.955980122991));
#31855=CARTESIAN_POINT('Ctrl Pts',(-0.04842903935518,2.342223142484,3.722320777306));
#31856=CARTESIAN_POINT('Ctrl Pts',(-0.04750543477618,2.336759152394,3.723920396082));
#31857=CARTESIAN_POINT('Ctrl Pts',(-0.04291667013141,2.309736402476,3.731867928017));
#31858=CARTESIAN_POINT('Ctrl Pts',(-0.03459915065528,2.261875354762,3.746274291935));
#31859=CARTESIAN_POINT('Ctrl Pts',(-0.02322915381834,2.198975091133,3.765967704986));
#31860=CARTESIAN_POINT('Ctrl Pts',(-0.01151371840005,2.136868627655,3.786259434136));
#31861=CARTESIAN_POINT('Ctrl Pts',(0.0009395902779249,2.074121416472,3.807829197551));
#31862=CARTESIAN_POINT('Ctrl Pts',(0.01478980849077,2.00888405034,3.831818479172));
#31863=CARTESIAN_POINT('Ctrl Pts',(0.02612878395871,1.960130298146,3.851458160798));
#31864=CARTESIAN_POINT('Ctrl Pts',(0.03276598174019,1.933903035583,3.862954124575));
#31865=CARTESIAN_POINT('Ctrl Pts',(0.03409521153101,1.928749916997,3.865256418107));
#31866=CARTESIAN_POINT('Ctrl Pts',(-0.0891849279982,2.304179010464,3.615799475541));
#31867=CARTESIAN_POINT('Ctrl Pts',(-0.08824084421946,2.298595247152,3.61743441963));
#31868=CARTESIAN_POINT('Ctrl Pts',(-0.08355321678755,2.270995008595,3.625552608771));
#31869=CARTESIAN_POINT('Ctrl Pts',(-0.07507257221585,2.222192578715,3.640241510491));
#31870=CARTESIAN_POINT('Ctrl Pts',(-0.06343491265144,2.157810236795,3.660398530094));
#31871=CARTESIAN_POINT('Ctrl Pts',(-0.05140958072686,2.094056832808,3.681227015441));
#31872=CARTESIAN_POINT('Ctrl Pts',(-0.03851290641217,2.029064832183,3.703564710746));
#31873=CARTESIAN_POINT('Ctrl Pts',(-0.02400792010097,1.96073197423,3.728688083965));
#31874=CARTESIAN_POINT('Ctrl Pts',(-0.01193529529924,1.908779020696,3.749598483488));
#31875=CARTESIAN_POINT('Ctrl Pts',(-0.004640481584497,1.879942869568,3.762233471476));
#31876=CARTESIAN_POINT('Ctrl Pts',(-0.003168746593044,1.87423250976,3.764782591257));
#31877=CARTESIAN_POINT('Ctrl Pts',(-0.1094003325662,2.267770953937,3.503012226299));
#31878=CARTESIAN_POINT('Ctrl Pts',(-0.1084366464606,2.262072587335,3.504680983176));
#31879=CARTESIAN_POINT('Ctrl Pts',(-0.1036543927112,2.233919770715,3.512962516607));
#31880=CARTESIAN_POINT('Ctrl Pts',(-0.09501763858581,2.184216444809,3.527921804991));
#31881=CARTESIAN_POINT('Ctrl Pts',(-0.08312382769833,2.118415764526,3.54852249276));
#31882=CARTESIAN_POINT('Ctrl Pts',(-0.07080192702584,2.053086250209,3.569864649964));
#31883=CARTESIAN_POINT('Ctrl Pts',(-0.05748095495493,1.985946002084,3.592937250614));
#31884=CARTESIAN_POINT('Ctrl Pts',(-0.0423493602444,1.914650780515,3.619145941414));
#31885=CARTESIAN_POINT('Ctrl Pts',(-0.02957463824225,1.859636214095,3.641272408901));
#31886=CARTESIAN_POINT('Ctrl Pts',(-0.02165049076681,1.828303375201,3.654997434942));
#31887=CARTESIAN_POINT('Ctrl Pts',(-0.02004237931471,1.822059739515,3.657782765687));
#31888=CARTESIAN_POINT('Origin',(0.9394619912652,1.984948516829,3.427195899532));
#31889=CARTESIAN_POINT('Ctrl Pts',(0.2115271085781,2.123801978059,4.099083165178));
#31890=CARTESIAN_POINT('Ctrl Pts',(0.2121262002231,2.114600129107,4.101333173451));
#31891=CARTESIAN_POINT('Ctrl Pts',(0.2164404968357,2.037191262064,4.119100527721));
#31892=CARTESIAN_POINT('Ctrl Pts',(0.2139962921771,1.899196368833,4.13258925162));
#31893=CARTESIAN_POINT('Ctrl Pts',(0.199524436147,1.716490317037,4.126202722674));
#31894=CARTESIAN_POINT('Ctrl Pts',(0.1774106709109,1.531708228466,4.100979757227));
#31895=CARTESIAN_POINT('Ctrl Pts',(0.1581803697853,1.403457455766,4.072215873524));
#31896=CARTESIAN_POINT('Ctrl Pts',(0.1469204644944,1.334496569053,4.053834130917));
#31897=CARTESIAN_POINT('Ctrl Pts',(0.1458524770939,1.328006904403,4.052078570375));
#31898=CARTESIAN_POINT('Ctrl Pts',(0.08366135428003,2.034390998194,3.978928836562));
#31899=CARTESIAN_POINT('Ctrl Pts',(0.08417860878662,2.026727285286,3.980132428517));
#31900=CARTESIAN_POINT('Ctrl Pts',(0.08801831539764,1.962051030615,3.989335305632));
#31901=CARTESIAN_POINT('Ctrl Pts',(0.08768495610394,1.843574140367,3.991294021376));
#31902=CARTESIAN_POINT('Ctrl Pts',(0.0790739523643,1.682126401741,3.97369060683));
#31903=CARTESIAN_POINT('Ctrl Pts',(0.06477019106634,1.515735601788,3.939795644756));
#31904=CARTESIAN_POINT('Ctrl Pts',(0.05184529653118,1.398767721864,3.906400952433));
#31905=CARTESIAN_POINT('Ctrl Pts',(0.04416796124159,1.3355924808,3.885851412206));
#31906=CARTESIAN_POINT('Ctrl Pts',(0.0434388747213,1.329644894934,3.883894614747));
#31907=CARTESIAN_POINT('Ctrl Pts',(0.002069708769611,1.941910036321,3.825396483512));
#31908=CARTESIAN_POINT('Ctrl Pts',(0.002564130319744,1.935902935356,3.825625402323));
#31909=CARTESIAN_POINT('Ctrl Pts',(0.006443211256808,1.884925816002,3.826897945044));
#31910=CARTESIAN_POINT('Ctrl Pts',(0.009358963854998,1.787220641492,3.81893556933));
#31911=CARTESIAN_POINT('Ctrl Pts',(0.008197891072037,1.647895242108,3.792711139866));
#31912=CARTESIAN_POINT('Ctrl Pts',(0.003243085717919,1.500137582073,3.75300481842));
#31913=CARTESIAN_POINT('Ctrl Pts',(-0.002415465510452,1.394244822581,3.717041504595));
#31914=CARTESIAN_POINT('Ctrl Pts',(-0.00603250719455,1.336650568951,3.695440705072));
#31915=CARTESIAN_POINT('Ctrl Pts',(-0.006378080860699,1.33122498004,3.693387794139));
#31916=CARTESIAN_POINT('Ctrl Pts',(-0.02637845939937,1.854145254949,3.651412310807));
#31917=CARTESIAN_POINT('Ctrl Pts',(-0.02584594427012,1.849773768258,3.650820359384));
#31918=CARTESIAN_POINT('Ctrl Pts',(-0.021416839685,1.812308948769,3.645464381648));
#31919=CARTESIAN_POINT('Ctrl Pts',(-0.01438725808483,1.734880389255,3.630025108279));
#31920=CARTESIAN_POINT('Ctrl Pts',(-0.007136546264389,1.616678829914,3.598501355566));
#31921=CARTESIAN_POINT('Ctrl Pts',(-0.001990551510268,1.486227398703,3.556333582309));
#31922=CARTESIAN_POINT('Ctrl Pts',(-3.359111288803E-5,1.390269550117,3.520080091633));
#31923=CARTESIAN_POINT('Ctrl Pts',(0.0005455399378233,1.337581750887,3.498633078821));
#31924=CARTESIAN_POINT('Ctrl Pts',(0.0005958023632368,1.332614129104,3.496597269846));
#31925=CARTESIAN_POINT('Ctrl Pts',(-0.0201796772031231,1.8533485682179,
3.67573602729754));
#31926=CARTESIAN_POINT('Ctrl Pts',(-0.0180484169316047,1.8332062091452,
3.67329927372651));
#31927=CARTESIAN_POINT('Ctrl Pts',(-0.0161673154615857,1.81251453951732,
3.67012899402731));
#31928=CARTESIAN_POINT('Ctrl Pts',(-0.0144832545962451,1.79133257575351,
3.66632891140682));
#31929=CARTESIAN_POINT('Ctrl Pts',(-0.0132428308424302,1.77573063906237,
3.66352989573825));
#31930=CARTESIAN_POINT('Ctrl Pts',(-0.0121097653213558,1.75986214367113,
3.66038763081213));
#31931=CARTESIAN_POINT('Ctrl Pts',(-0.0110658077287692,1.74375337710359,
3.65693080646843));
#31932=CARTESIAN_POINT('Ctrl Pts',(-0.0110657287678007,1.74375215869796,
3.65693054500743));
#31933=CARTESIAN_POINT('Ctrl Pts',(-0.0110656498073422,1.74375094029096,
3.65693028354462));
#31934=CARTESIAN_POINT('Ctrl Pts',(-0.0110655708473939,1.74374972188258,
3.65693002208001));
#31935=CARTESIAN_POINT('Ctrl Pts',(-0.00930360226254986,1.71656128866799,
3.65109551441564));
#31936=CARTESIAN_POINT('Ctrl Pts',(-0.00779274517230981,1.68868734172387,
3.64437242260396));
#31937=CARTESIAN_POINT('Ctrl Pts',(-0.00648446807086871,1.6598387869057,
3.63673330275129));
#31938=CARTESIAN_POINT('Ctrl Pts',(-0.00596516871011799,1.64838782131198,
3.63370107811644));
#31939=CARTESIAN_POINT('Ctrl Pts',(-0.00547802320827809,1.63678336231907,
3.6305239294403));
#31940=CARTESIAN_POINT('Ctrl Pts',(-0.00502072425409526,1.62500842706159,
3.62719837418674));
#31941=CARTESIAN_POINT('Ctrl Pts',(-0.0038958181749634,1.59604335698791,
3.61901786713113));
#31942=CARTESIAN_POINT('Ctrl Pts',(-0.00295103873268496,1.56604766064031,
3.60994448283711));
#31943=CARTESIAN_POINT('Ctrl Pts',(-0.00219243495539221,1.53482829685866,
3.59984407614345));
#31944=CARTESIAN_POINT('Ctrl Pts',(-0.00186572146376575,1.52138282288031,
3.59549405939358));
#31945=CARTESIAN_POINT('Ctrl Pts',(-0.00157359566811571,1.50771092696239,
3.59095334765681));
#31946=CARTESIAN_POINT('Ctrl Pts',(-0.00131664102690395,1.49380028354877,
3.58621075218851));
#31947=CARTESIAN_POINT('Ctrl Pts',(-0.000714403889778184,1.46119722946308,
3.57509529965609));
#31948=CARTESIAN_POINT('Ctrl Pts',(-0.000305670842863149,1.42727766026637,
3.56287477923549));
#31949=CARTESIAN_POINT('Ctrl Pts',(-0.000118133862968915,1.39214305106515,
3.54946527329762));
#31950=CARTESIAN_POINT('Ctrl Pts',(-3.98644057114186E-5,1.37747945354596,
3.54386875173457));
#31951=CARTESIAN_POINT('Ctrl Pts',(-4.70921629019157E-9,1.36260469734931,
3.53806544891218));
#31952=CARTESIAN_POINT('Ctrl Pts',(4.91088626388035E-16,1.34752836903785,
3.5320508077706));
#31953=CARTESIAN_POINT('Origin',(-0.5,3.8,0.));
#31954=CARTESIAN_POINT('Origin',(-0.5,3.8,0.));
#31955=CARTESIAN_POINT('Origin',(-0.5,3.8,0.));
#31956=CARTESIAN_POINT('',(-1.,3.76739364408005,3.29983890903081));
#31957=CARTESIAN_POINT('Origin',(-1.,3.8,0.));
#31958=CARTESIAN_POINT('Origin',(-0.5,3.76739364408005,3.29983890903081));
#31959=CARTESIAN_POINT('Origin',(-0.5,3.8,0.));
#31960=CARTESIAN_POINT('Origin',(-0.5,3.8,0.));
#31961=CARTESIAN_POINT('',(-0.0201844691181272,1.85335594570995,-3.67572064370324));
#31962=CARTESIAN_POINT('Ctrl Pts',(-0.0201847187606871,1.85335594052431,
-3.67572046601124));
#31963=CARTESIAN_POINT('Ctrl Pts',(-0.0178286956184653,1.83115373899016,
-3.67305838240737));
#31964=CARTESIAN_POINT('Ctrl Pts',(-0.0158360667308249,1.80880940789044,
-3.66956936811219));
#31965=CARTESIAN_POINT('Ctrl Pts',(-0.014084148622304,1.78626234395626,
-3.6654249360026));
#31966=CARTESIAN_POINT('Ctrl Pts',(-0.0137453719972492,1.7819023124072,
-3.66462350771893));
#31967=CARTESIAN_POINT('Ctrl Pts',(-0.0134157389998275,1.77753464578999,
-3.66379760651892));
#31968=CARTESIAN_POINT('Ctrl Pts',(-0.0130945604005602,1.77315882973048,
-3.66294851672634));
#31969=CARTESIAN_POINT('Ctrl Pts',(-0.0111124584923371,1.74615418688884,
-3.65770849605876));
#31970=CARTESIAN_POINT('Ctrl Pts',(-0.00945014572111559,1.71884148228237,
-3.65158466669008));
#31971=CARTESIAN_POINT('Ctrl Pts',(-0.00803275747314458,1.69159897117484,
-3.64485043816951));
#31972=CARTESIAN_POINT('Ctrl Pts',(-0.0066153692251727,1.6643564600673,
-3.63811620964893));
#31973=CARTESIAN_POINT('Ctrl Pts',(-0.00544334631616801,1.63718405974905,
-3.63077174059948));
#31974=CARTESIAN_POINT('Ctrl Pts',(-0.0044617006739997,1.61012025342433,
-3.62294164204283));
#31975=CARTESIAN_POINT('Ctrl Pts',(-0.00360980208403964,1.58663355164868,
-3.61614647112462));
#31976=CARTESIAN_POINT('Ctrl Pts',(-0.00290086724187045,1.5632287435596,
-3.60898422005949));
#31977=CARTESIAN_POINT('Ctrl Pts',(-0.00230378770602957,1.53931614496347,
-3.6012916794294));
#31978=CARTESIAN_POINT('Ctrl Pts',(-0.00221285046229865,1.53567417488035,
-3.60012007933226));
#31979=CARTESIAN_POINT('Ctrl Pts',(-0.00212456287768805,1.53202042666967,
-3.59893609696379));
#31980=CARTESIAN_POINT('Ctrl Pts',(-0.00203887417552023,1.52835281933648,
-3.59773906580883));
#31981=CARTESIAN_POINT('Ctrl Pts',(-0.00146807360102199,1.5039216829106,
-3.58976524833164));
#31982=CARTESIAN_POINT('Ctrl Pts',(-0.0010109478997301,1.47887566655908,
-3.58121621087756));
#31983=CARTESIAN_POINT('Ctrl Pts',(-0.000671404729556291,1.45271668694635,
-3.57185779465556));
#31984=CARTESIAN_POINT('Ctrl Pts',(-0.000625299613279142,1.44916467087687,
-3.57058705530343));
#31985=CARTESIAN_POINT('Ctrl Pts',(-0.000581394318175335,1.44559214758773,
-3.56930132189872));
#31986=CARTESIAN_POINT('Ctrl Pts',(-0.000539729159247049,1.4419978838711,
-3.56799993917551));
#31987=CARTESIAN_POINT('Ctrl Pts',(-0.000191219093601024,1.41193350595798,
-3.55711446579763));
#31988=CARTESIAN_POINT('Ctrl Pts',(9.14699587802441E-12,1.3803466764801,
-3.54514076878014));
#31989=CARTESIAN_POINT('Ctrl Pts',(0.,1.347528369805,-3.53205080767908));
#31990=CARTESIAN_POINT('Origin',(-0.4999999999811,0.6012805114691,-2.873707297839));
#31991=CARTESIAN_POINT('Origin',(-0.5,1.7875388203,-3.800000000026));
#31992=CARTESIAN_POINT('Ctrl Pts',(-0.02638274264885,1.854145296489,-3.651397889487));
#31993=CARTESIAN_POINT('Ctrl Pts',(-0.02584988028328,1.849776362744,-3.650806899679));
#31994=CARTESIAN_POINT('Ctrl Pts',(-0.02244403090875,1.820986653244,-3.646694311958));
#31995=CARTESIAN_POINT('Ctrl Pts',(-0.01704332156225,1.765138511257,-3.636247413713));
#31996=CARTESIAN_POINT('Ctrl Pts',(-0.011276325478,1.685711356068,-3.617149671255));
#31997=CARTESIAN_POINT('Ctrl Pts',(-0.006856393552252,1.605666931733,-3.594547441496));
#31998=CARTESIAN_POINT('Ctrl Pts',(-0.003478222547858,1.523897199579,-3.568495084708));
#31999=CARTESIAN_POINT('Ctrl Pts',(-0.0009679363545506,1.437662225789,-3.538088485335));
#32000=CARTESIAN_POINT('Ctrl Pts',(0.0001515744128949,1.373436283524,-3.513228241255));
#32001=CARTESIAN_POINT('Ctrl Pts',(0.0005455151103873,1.337581706695,-3.498632990864));
#32002=CARTESIAN_POINT('Ctrl Pts',(0.0005957202757987,1.332613906773,-3.496597029118));
#32003=CARTESIAN_POINT('Ctrl Pts',(0.00205755759891,1.941929047829,-3.825367870495));
#32004=CARTESIAN_POINT('Ctrl Pts',(0.002553460349221,1.935923592207,-3.825601796816));
#32005=CARTESIAN_POINT('Ctrl Pts',(0.005541994612222,1.896743544731,-3.826597574823));
#32006=CARTESIAN_POINT('Ctrl Pts',(0.008399401037005,1.825089858117,-3.822450688835));
#32007=CARTESIAN_POINT('Ctrl Pts',(0.009008797399017,1.729047222386,-3.808392608073));
#32008=CARTESIAN_POINT('Ctrl Pts',(0.007576840272114,1.635755871874,-3.788775319885));
#32009=CARTESIAN_POINT('Ctrl Pts',(0.004676582779189,1.542788345155,-3.764464411949));
#32010=CARTESIAN_POINT('Ctrl Pts',(0.0004113178430084,1.446514215098,-3.734924187794));
#32011=CARTESIAN_POINT('Ctrl Pts',(-0.003570928637939,1.375843575995,-3.710140370327));
#32012=CARTESIAN_POINT('Ctrl Pts',(-0.006032522862356,1.336650553949,-3.695440720027));
#32013=CARTESIAN_POINT('Ctrl Pts',(-0.006378128922918,1.331224937371,-3.693387619733));
#32014=CARTESIAN_POINT('Ctrl Pts',(0.08364112782225,2.034430165208,-3.978886092457));
#32015=CARTESIAN_POINT('Ctrl Pts',(0.08416102368134,2.026767191475,-3.98009867518));
#32016=CARTESIAN_POINT('Ctrl Pts',(0.0871248314785,1.977053136641,-3.987203326034));
#32017=CARTESIAN_POINT('Ctrl Pts',(0.08809270195467,1.889253530143,-3.991157591204));
#32018=CARTESIAN_POINT('Ctrl Pts',(0.08428392479652,1.775987832278,-3.984476044373));
#32019=CARTESIAN_POINT('Ctrl Pts',(0.07759850531386,1.66873570053,-3.970038442414));
#32020=CARTESIAN_POINT('Ctrl Pts',(0.06890748642892,1.563749976296,-3.949586172014));
#32021=CARTESIAN_POINT('Ctrl Pts',(0.05826440232022,1.4564802135,-3.92303550761));
#32022=CARTESIAN_POINT('Ctrl Pts',(0.04939263231509,1.378583011643,-3.899835567345));
#32023=CARTESIAN_POINT('Ctrl Pts',(0.04416795177121,1.335592487269,-3.885851523854));
#32024=CARTESIAN_POINT('Ctrl Pts',(0.04343885083342,1.329645016683,-3.883894494899));
#32025=CARTESIAN_POINT('Ctrl Pts',(0.2114992793448,2.123860789188,-4.099027540324));
#32026=CARTESIAN_POINT('Ctrl Pts',(0.2121021010075,2.114658850969,-4.101290124628));
#32027=CARTESIAN_POINT('Ctrl Pts',(0.2154358527566,2.055153999154,-4.11498983687));
#32028=CARTESIAN_POINT('Ctrl Pts',(0.2153270381774,1.952227455737,-4.128164339508));
#32029=CARTESIAN_POINT('Ctrl Pts',(0.2082114888224,1.822581159193,-4.130575153272));
#32030=CARTESIAN_POINT('Ctrl Pts',(0.1973133334883,1.701829778055,-4.123075893756));
#32031=CARTESIAN_POINT('Ctrl Pts',(0.1838067564356,1.585017290136,-4.108274582941));
#32032=CARTESIAN_POINT('Ctrl Pts',(0.1677205468331,1.466721163078,-4.086584965633));
#32033=CARTESIAN_POINT('Ctrl Pts',(0.1545831460761,1.381423951742,-4.066343003277));
#32034=CARTESIAN_POINT('Ctrl Pts',(0.1469204577389,1.334496587465,-4.053834324906));
#32035=CARTESIAN_POINT('Ctrl Pts',(0.1458524654956,1.328007161482,-4.05207848873));
#32036=CARTESIAN_POINT('Origin',(0.9394505533555,1.984989544106,-3.427176090634));
#32037=CARTESIAN_POINT('Origin',(1.,1.347528370653,-3.532050807569));
#32038=CARTESIAN_POINT('Origin',(1.,7.013523051583,-3.532050807569));
#32039=CARTESIAN_POINT('Origin',(1.00128642976697,0.666005481541297,-3.53122253848802));
#32040=CARTESIAN_POINT('Ctrl Pts',(0.1488993956888,0.7179069965694,-4.051886351638));
#32041=CARTESIAN_POINT('Ctrl Pts',(0.1385570697474,0.7162110101831,-4.035126874871));
#32042=CARTESIAN_POINT('Ctrl Pts',(0.1176862605854,0.7126138946773,-3.998941337807));
#32043=CARTESIAN_POINT('Ctrl Pts',(0.08933527303172,0.7071386038102,-3.94173474656));
#32044=CARTESIAN_POINT('Ctrl Pts',(0.06394561213802,0.7015141325995,-3.880575776974));
#32045=CARTESIAN_POINT('Ctrl Pts',(0.04268217099292,0.6959732845635,-3.817856726743));
#32046=CARTESIAN_POINT('Ctrl Pts',(0.0256383433447,0.6905443235702,-3.753851548948));
#32047=CARTESIAN_POINT('Ctrl Pts',(0.01289006426926,0.6852543476883,-3.688839944825));
#32048=CARTESIAN_POINT('Ctrl Pts',(0.004495469108308,0.6801291657042,-3.623106745103));
#32049=CARTESIAN_POINT('Ctrl Pts',(0.0007024534571773,0.675450952114,-3.560399066502));
#32050=CARTESIAN_POINT('Ctrl Pts',(0.0007422179452603,0.6725379290189,-3.519663636229));
#32051=CARTESIAN_POINT('Ctrl Pts',(0.001283538221875,0.6712323506797,-3.501040402923));
#32052=CARTESIAN_POINT('Ctrl Pts',(0.1340962252224,0.3912294572926,-4.093199135617));
#32053=CARTESIAN_POINT('Ctrl Pts',(0.1234350361148,0.3894754713328,-4.075866781342));
#32054=CARTESIAN_POINT('Ctrl Pts',(0.1019235019593,0.3857557331309,-4.038448847312));
#32055=CARTESIAN_POINT('Ctrl Pts',(0.0726982435266,0.3800930011241,-3.979286595073));
#32056=CARTESIAN_POINT('Ctrl Pts',(0.04652749766874,0.3742762828842,-3.91604080453));
#32057=CARTESIAN_POINT('Ctrl Pts',(0.02460901325779,0.3685458257877,-3.851179458001));
#32058=CARTESIAN_POINT('Ctrl Pts',(0.007040378848643,0.3629311721167,-3.784988888268));
#32059=CARTESIAN_POINT('Ctrl Pts',(-0.006100719778655,0.3574601784024,-3.717755935732));
#32060=CARTESIAN_POINT('Ctrl Pts',(-0.01475389334159,0.3521598165628,-3.649778458152));
#32061=CARTESIAN_POINT('Ctrl Pts',(-0.01866387237992,0.347321433533,-3.584924958567));
#32062=CARTESIAN_POINT('Ctrl Pts',(-0.01862296859118,0.3443090775689,-3.542800463296));
#32063=CARTESIAN_POINT('Ctrl Pts',(-0.01806492014634,0.342958842281,-3.523540054914));
#32064=CARTESIAN_POINT('Ctrl Pts',(0.3373468963971,0.1525661114051,-3.991350865212));
#32065=CARTESIAN_POINT('Ctrl Pts',(0.3290504156986,0.1512072534401,-3.977811610559));
#32066=CARTESIAN_POINT('Ctrl Pts',(0.3123100833698,0.1483247372964,-3.948582265489));
#32067=CARTESIAN_POINT('Ctrl Pts',(0.2895668155851,0.1439336916915,-3.902367297901));
#32068=CARTESIAN_POINT('Ctrl Pts',(0.269201233379,0.1394199538792,-3.85296441848));
#32069=CARTESIAN_POINT('Ctrl Pts',(0.25214516126,0.1349694701275,-3.802301466759));
#32070=CARTESIAN_POINT('Ctrl Pts',(0.2384747042055,0.1306050036345,-3.750603437919));
#32071=CARTESIAN_POINT('Ctrl Pts',(0.2282499930638,0.1263479786245,-3.69809469861));
#32072=CARTESIAN_POINT('Ctrl Pts',(0.2215177543611,0.1222192691329,-3.645009086964));
#32073=CARTESIAN_POINT('Ctrl Pts',(0.2184760069348,0.1184459109448,-3.594367048629));
#32074=CARTESIAN_POINT('Ctrl Pts',(0.2185078803864,0.1160938128734,-3.561476552185));
#32075=CARTESIAN_POINT('Ctrl Pts',(0.2189419602036,0.1150389389891,-3.546438857281));
#32076=CARTESIAN_POINT('Ctrl Pts',(0.6168657267359,0.1684061772862,-3.817389898812));
#32077=CARTESIAN_POINT('Ctrl Pts',(0.6119679285382,0.1676199374555,-3.809363691671));
#32078=CARTESIAN_POINT('Ctrl Pts',(0.6020823810763,0.165950450196,-3.792031641834));
#32079=CARTESIAN_POINT('Ctrl Pts',(0.5886555921188,0.1634031025247,-3.76463500526));
#32080=CARTESIAN_POINT('Ctrl Pts',(0.5766317967327,0.1607786261806,-3.735348089483));
#32081=CARTESIAN_POINT('Ctrl Pts',(0.5665636211538,0.1581848012789,-3.705319562176));
#32082=CARTESIAN_POINT('Ctrl Pts',(0.5584949951317,0.1556342834582,-3.674682152124));
#32083=CARTESIAN_POINT('Ctrl Pts',(0.5524614350958,0.1531393609817,-3.643571720386));
#32084=CARTESIAN_POINT('Ctrl Pts',(0.5484896191243,0.1507118028103,-3.612125698284));
#32085=CARTESIAN_POINT('Ctrl Pts',(0.5466956284192,0.1484857128208,-3.58213862691));
#32086=CARTESIAN_POINT('Ctrl Pts',(0.5467146013709,0.1470928739485,-3.56266364575));
#32087=CARTESIAN_POINT('Ctrl Pts',(0.5469704950681,0.1464673385908,-3.55376282921));
#32088=CARTESIAN_POINT('',(0.51744976844956,0.145564598942594,-3.56771956646391));
#32089=CARTESIAN_POINT('Origin',(0.5,0.6439853787897,-3.532051214103));
#32090=CARTESIAN_POINT('',(0.584436854370166,0.166625187839343,-3.82024516063688));
#32091=CARTESIAN_POINT('Origin',(0.5669870682482,0.6648587286911,-3.78205040944));
#32092=CARTESIAN_POINT('Origin',(1.0290517906493,0.168032215480016,-3.56615971227102));
#32093=CARTESIAN_POINT('Origin',(0.5,50.,0.));
#32094=CARTESIAN_POINT('Origin',(0.5174497483513,50.,0.));
#32095=CARTESIAN_POINT('Ctrl Pts',(1.76192394008012E-13,0.60128128325064,
-2.87370766691881));
#32096=CARTESIAN_POINT('Ctrl Pts',(1.54230945546585E-8,0.580269199198493,
-2.82882528737468));
#32097=CARTESIAN_POINT('Ctrl Pts',(0.00101186006611363,0.560042231212748,
-2.78388483535608));
#32098=CARTESIAN_POINT('Ctrl Pts',(0.00280079850496784,0.540720477220154,
-2.73936883200466));
#32099=CARTESIAN_POINT('Ctrl Pts',(0.00380243770949192,0.529902091366951,
-2.71444400887096));
#32100=CARTESIAN_POINT('Ctrl Pts',(0.0050478023941539,0.519366499347649,
-2.68965236124796));
#32101=CARTESIAN_POINT('Ctrl Pts',(0.00649712134262853,0.509127913931286,
-2.66507931910599));
#32102=CARTESIAN_POINT('Ctrl Pts',(0.00834719043388274,0.496058264606053,
-2.63371160270872));
#32103=CARTESIAN_POINT('Ctrl Pts',(0.01052439600924,0.483477583764246,-2.60269882830449));
#32104=CARTESIAN_POINT('Ctrl Pts',(0.0130034531453356,0.471191494462817,
-2.57159451210596));
#32105=CARTESIAN_POINT('Ctrl Pts',(0.0155308113117525,0.458666027551556,
-2.53988417094012));
#32106=CARTESIAN_POINT('Ctrl Pts',(0.0183721278713497,0.446446178960187,
-2.50807870851953));
#32107=CARTESIAN_POINT('Ctrl Pts',(0.0215529360868368,0.434336243117764,
-2.47570186212255));
#32108=CARTESIAN_POINT('Ctrl Pts',(0.0220616550262061,0.43239945432063,
-2.47052370806755));
#32109=CARTESIAN_POINT('Ctrl Pts',(0.0225791610348015,0.430465508274142,
-2.46533093177464));
#32110=CARTESIAN_POINT('Ctrl Pts',(0.0231056752010314,0.428533643225277,
-2.46012157690981));
#32111=CARTESIAN_POINT('Ctrl Pts',(0.027524337805662,0.412320860367524,
-2.41640313016732));
#32112=CARTESIAN_POINT('Ctrl Pts',(0.0325718997013263,0.396259498057867,
-2.37151833744439));
#32113=CARTESIAN_POINT('Ctrl Pts',(0.0383080237524296,0.380265594004233,
-2.32497070433188));
#32114=CARTESIAN_POINT('Ctrl Pts',(0.0417209920361136,0.370749292267901,
-2.29727506977478));
#32115=CARTESIAN_POINT('Ctrl Pts',(0.0453785461737294,0.36125733554204,
-2.26899068908822));
#32116=CARTESIAN_POINT('Ctrl Pts',(0.0493002060251221,0.351777440828857,
-2.24001235735313));
#32117=CARTESIAN_POINT('Ctrl Pts',(0.0570020472340432,0.333159649759522,
-2.18310112129989));
#32118=CARTESIAN_POINT('Ctrl Pts',(0.0657293147580703,0.314588190128329,
-2.12351422609263));
#32119=CARTESIAN_POINT('Ctrl Pts',(0.0754853867545444,0.296324974395133,
-2.06149859166281));
#32120=CARTESIAN_POINT('Ctrl Pts',(0.0790459994386625,0.289659562576123,
-2.03886513276211));
#32121=CARTESIAN_POINT('Ctrl Pts',(0.0827431515444289,0.283035186810901,
-2.01590821646305));
#32122=CARTESIAN_POINT('Ctrl Pts',(0.0865752842350387,0.276464377489038,
-1.99264001890476));
#32123=CARTESIAN_POINT('Ctrl Pts',(-0.001081260139011,0.5856903810519,-2.906543661707));
#32124=CARTESIAN_POINT('Ctrl Pts',(-0.001018369255986,0.5835992009094,-2.902147314851));
#32125=CARTESIAN_POINT('Ctrl Pts',(0.0001871679450526,0.5490075761878,-2.829131820991));
#32126=CARTESIAN_POINT('Ctrl Pts',(0.007507857493721,0.4863027823338,-2.687558940315));
#32127=CARTESIAN_POINT('Ctrl Pts',(0.02870561913676,0.4029671144941,-2.474508650036));
#32128=CARTESIAN_POINT('Ctrl Pts',(0.05928519434814,0.3254023673231,-2.249119982873));
#32129=CARTESIAN_POINT('Ctrl Pts',(0.08618036230882,0.2770329575424,-2.086634502439));
#32130=CARTESIAN_POINT('Ctrl Pts',(0.1018793569146,0.2529095911706,-1.998560749934));
#32131=CARTESIAN_POINT('Ctrl Pts',(0.1027383636877,0.2516008013594,-1.993759888543));
#32132=CARTESIAN_POINT('Ctrl Pts',(0.02046330720854,0.8229529422841,-2.691466056719));
#32133=CARTESIAN_POINT('Ctrl Pts',(0.01962993973341,0.8212308194753,-2.687387423694));
#32134=CARTESIAN_POINT('Ctrl Pts',(0.005955867276286,0.7926322259833,-2.619615027721));
#32135=CARTESIAN_POINT('Ctrl Pts',(-0.01530270840099,0.7372776063719,-2.487237441822));
#32136=CARTESIAN_POINT('Ctrl Pts',(-0.03473413003973,0.6558327993806,-2.285821170463));
#32137=CARTESIAN_POINT('Ctrl Pts',(-0.04384970159776,0.5726974889928,-2.070790001253));
#32138=CARTESIAN_POINT('Ctrl Pts',(-0.04272135475251,0.5157102080513,-1.914480858456));
#32139=CARTESIAN_POINT('Ctrl Pts',(-0.04008670908317,0.4858251163379,-1.829403670676));
#32140=CARTESIAN_POINT('Ctrl Pts',(-0.03993718883915,0.484199085711,-1.824765062074));
#32141=CARTESIAN_POINT('Ctrl Pts',(-0.2045700640878,0.9936004720384,-2.53896888117));
#32142=CARTESIAN_POINT('Ctrl Pts',(-0.2060475584221,0.9912751192331,-2.535166077691));
#32143=CARTESIAN_POINT('Ctrl Pts',(-0.2303376413689,0.952617100583,-2.471943726365));
#32144=CARTESIAN_POINT('Ctrl Pts',(-0.2695762730753,0.8764813310992,-2.347474954217));
#32145=CARTESIAN_POINT('Ctrl Pts',(-0.3093746426751,0.761702271861,-2.155847204795));
#32146=CARTESIAN_POINT('Ctrl Pts',(-0.3336343557535,0.6422051540402,-1.949271087601));
#32147=CARTESIAN_POINT('Ctrl Pts',(-0.3389528302416,0.5587940338812,-1.797815533392));
#32148=CARTESIAN_POINT('Ctrl Pts',(-0.3385904718372,0.5146537484191,-1.715024763658));
#32149=CARTESIAN_POINT('Ctrl Pts',(-0.3385612404185,0.5122508977145,-1.710509733302));
#32150=CARTESIAN_POINT('Ctrl Pts',(-0.5251165549145,0.9830773465599,-2.551423432733));
#32151=CARTESIAN_POINT('Ctrl Pts',(-0.526553642486,0.9795814245021,-2.547669410243));
#32152=CARTESIAN_POINT('Ctrl Pts',(-0.5500696128295,0.9215644127028,-2.485249607032));
#32153=CARTESIAN_POINT('Ctrl Pts',(-0.5846190863906,0.8104665474727,-2.362093983857));
#32154=CARTESIAN_POINT('Ctrl Pts',(-0.6108498439799,0.6495053941253,-2.171838228225));
#32155=CARTESIAN_POINT('Ctrl Pts',(-0.6155364367152,0.4872648925674,-1.966138843811));
#32156=CARTESIAN_POINT('Ctrl Pts',(-0.6036539839724,0.3773622786505,-1.814955916913));
#32157=CARTESIAN_POINT('Ctrl Pts',(-0.5932464655588,0.320042837336,-1.732206546957));
#32158=CARTESIAN_POINT('Ctrl Pts',(-0.5926675754179,0.3169250663232,-1.727693462271));
#32159=CARTESIAN_POINT('Origin',(6.513074473852,50.,0.));
#32160=CARTESIAN_POINT('',(3.164008715435,0.8114184892106,-8.333468366184));
#32161=CARTESIAN_POINT('Origin',(-2.18195397800361,50.0038044976864,1.00000511325181));
#32162=CARTESIAN_POINT('',(3.59702142554264,0.870223962352941,-8.58602404765116));
#32163=CARTESIAN_POINT('Ctrl Pts',(3.597021417327,0.87022396206158,-8.58602404765099));
#32164=CARTESIAN_POINT('Ctrl Pts',(3.58096741891376,0.869654514666955,-8.58602213943295));
#32165=CARTESIAN_POINT('Ctrl Pts',(3.56518530891056,0.868960131303695,-8.58525072062108));
#32166=CARTESIAN_POINT('Ctrl Pts',(3.54962915365496,0.86814840013051,-8.58376106038573));
#32167=CARTESIAN_POINT('Ctrl Pts',(3.53367433186178,0.867315866255697,-8.58223322377077));
#32168=CARTESIAN_POINT('Ctrl Pts',(3.5179562710213,0.866359828090631,-8.57994970308851));
#32169=CARTESIAN_POINT('Ctrl Pts',(3.50242592358464,0.865279182771811,-8.57691263234756));
#32170=CARTESIAN_POINT('Ctrl Pts',(3.49841119994216,0.864999826992535,-8.57612752436738));
#32171=CARTESIAN_POINT('Ctrl Pts',(3.49440906403718,0.864712099679328,-8.57529179512774));
#32172=CARTESIAN_POINT('Ctrl Pts',(3.49041879141317,0.86441589178025,-8.5744049385936));
#32173=CARTESIAN_POINT('Ctrl Pts',(3.47318074105317,0.863136268265153,-8.57057370222505));
#32174=CARTESIAN_POINT('Ctrl Pts',(3.45615454157413,0.861705014691857,-8.56582824079013));
#32175=CARTESIAN_POINT('Ctrl Pts',(3.43955788599333,0.860147262011866,-8.56026314162774));
#32176=CARTESIAN_POINT('Ctrl Pts',(3.42296123041252,0.858589509331876,-8.55469804246534));
#32177=CARTESIAN_POINT('Ctrl Pts',(3.40679497637281,0.856905386133462,-8.54831381496211));
#32178=CARTESIAN_POINT('Ctrl Pts',(3.3912488155045,0.855128074940696,-8.54125787790699));
#32179=CARTESIAN_POINT('Ctrl Pts',(3.37733685737159,0.853537593592125,-8.53494365655481));
#32180=CARTESIAN_POINT('Ctrl Pts',(3.36393280439972,0.851868343374866,-8.52806545984737));
#32181=CARTESIAN_POINT('Ctrl Pts',(3.35094736280191,0.850121891066415,-8.52064611424454));
#32182=CARTESIAN_POINT('Ctrl Pts',(3.33776993736112,0.848349618255577,-8.51311707699429));
#32183=CARTESIAN_POINT('Ctrl Pts',(3.3250228795613,0.846497749897992,-8.50503043014873));
#32184=CARTESIAN_POINT('Ctrl Pts',(3.31263028034128,0.844560035369382,-8.49636064042773));
#32185=CARTESIAN_POINT('Ctrl Pts',(3.30994179241995,0.844139661724381,-8.49447979004828));
#32186=CARTESIAN_POINT('Ctrl Pts',(3.30727007445323,0.843715221628018,-8.49257132260828));
#32187=CARTESIAN_POINT('Ctrl Pts',(3.30461450965066,0.843286609495757,-8.49063469802249));
#32188=CARTESIAN_POINT('Ctrl Pts',(3.29113505661424,0.841111005608376,-8.48080453303156));
#32189=CARTESIAN_POINT('Ctrl Pts',(3.27807398602321,0.83883055992351,-8.47026397611444));
#32190=CARTESIAN_POINT('Ctrl Pts',(3.26541716603687,0.83643339600023,-8.45893822789531));
#32191=CARTESIAN_POINT('Ctrl Pts',(3.25276034605054,0.83403623207695,-8.44761247967618));
#32192=CARTESIAN_POINT('Ctrl Pts',(3.24050695686514,0.831522216147609,-8.43550102903084));
#32193=CARTESIAN_POINT('Ctrl Pts',(3.22869302733891,0.828876288150112,-8.42249729172191));
#32194=CARTESIAN_POINT('Ctrl Pts',(3.21687909781269,0.826230360152616,-8.40949355441297));
#32195=CARTESIAN_POINT('Ctrl Pts',(3.20550581979188,0.823454018197384,-8.3956060278045));
#32196=CARTESIAN_POINT('Ctrl Pts',(3.19468036961139,0.820544747804952,-8.38078442938157));
#32197=CARTESIAN_POINT('Ctrl Pts',(3.18439707445734,0.817781178103046,-8.36670511917307));
#32198=CARTESIAN_POINT('Ctrl Pts',(3.17460781391463,0.814897544462127,-8.3517823765314));
#32199=CARTESIAN_POINT('Ctrl Pts',(3.1654515788303,0.811894466193472,-8.33597579569462));
#32200=CARTESIAN_POINT('Ctrl Pts',(3.16496884457052,0.811736138152337,-8.33514244246269));
#32201=CARTESIAN_POINT('Ctrl Pts',(3.16448788193827,0.811577479019006,-8.33430663436432));
#32202=CARTESIAN_POINT('Ctrl Pts',(3.164008715435,0.811418489210709,-8.33346836618398));
#32203=CARTESIAN_POINT('',(8.976377188873,1.060990939343,-8.586352585191));
#32204=CARTESIAN_POINT('',(8.976377188873,1.060990939343,-8.586352585191));
#32205=CARTESIAN_POINT('',(9.31255006972063,1.05006965735451,-8.45517202507966));
#32206=CARTESIAN_POINT('Ctrl Pts',(9.31255006975118,1.05006965736242,-8.45517202511191));
#32207=CARTESIAN_POINT('Ctrl Pts',(9.29074436206343,1.05275215314808,-8.4751756322404));
#32208=CARTESIAN_POINT('Ctrl Pts',(9.24411157801294,1.05729799350007,-8.51091803751234));
#32209=CARTESIAN_POINT('Ctrl Pts',(9.165072559821,1.061654875619,-8.551962189244));
#32210=CARTESIAN_POINT('Ctrl Pts',(9.076498905396,1.06329068312,-8.579231767789));
#32211=CARTESIAN_POINT('Ctrl Pts',(9.010839296144,1.062212801702,-8.586352781299));
#32212=CARTESIAN_POINT('Ctrl Pts',(8.976377188873,1.060990939343,-8.586352585191));
#32213=CARTESIAN_POINT('',(9.312550081826,1.050069655877,8.455172014035));
#32214=CARTESIAN_POINT('Ctrl Pts',(9.31255008182614,1.05006965587323,8.45517201403565));
#32215=CARTESIAN_POINT('Ctrl Pts',(9.49007071210251,1.02822813488135,8.29230332198047));
#32216=CARTESIAN_POINT('Ctrl Pts',(9.65651258488126,1.00678323034589,8.12919423308374));
#32217=CARTESIAN_POINT('Ctrl Pts',(9.81265533312651,0.985967919259792,7.96715327562526));
#32218=CARTESIAN_POINT('Ctrl Pts',(9.91037358013901,0.972941148992121,7.86574377383911));
#32219=CARTESIAN_POINT('Ctrl Pts',(10.0040580861799,0.960159921215438,7.76475277538954));
#32220=CARTESIAN_POINT('Ctrl Pts',(10.0938999473117,0.947671072743482,7.66450248813446));
#32221=CARTESIAN_POINT('Ctrl Pts',(10.3272989795294,0.915226451604224,7.40406353762623));
#32222=CARTESIAN_POINT('Ctrl Pts',(10.5347649834303,0.884750855204011,7.14862472245941));
#32223=CARTESIAN_POINT('Ctrl Pts',(10.7224474183718,0.856238063271469,6.89835151627484));
#32224=CARTESIAN_POINT('Ctrl Pts',(10.8811575891838,0.832126749501755,6.68671262041556));
#32225=CARTESIAN_POINT('Ctrl Pts',(11.0257204619308,0.809423428647549,6.47876703586414));
#32226=CARTESIAN_POINT('Ctrl Pts',(11.1579073453267,0.788181410825779,6.27570406781082));
#32227=CARTESIAN_POINT('Ctrl Pts',(11.1820378297224,0.784303717620428,6.23863527810894));
#32228=CARTESIAN_POINT('Ctrl Pts',(11.2057558983319,0.780474581389037,6.20172921156834));
#32229=CARTESIAN_POINT('Ctrl Pts',(11.2290723264035,0.776694143780084,6.16499312259368));
#32230=CARTESIAN_POINT('Ctrl Pts',(11.3801162342959,0.752204454868684,5.92701660138878));
#32231=CARTESIAN_POINT('Ctrl Pts',(11.5143056099425,0.729762942807907,5.6961725140216));
#32232=CARTESIAN_POINT('Ctrl Pts',(11.6344821728398,0.709301052844758,5.4738978660678));
#32233=CARTESIAN_POINT('Ctrl Pts',(11.7107469682605,0.696315810012572,5.3328409898791));
#32234=CARTESIAN_POINT('Ctrl Pts',(11.7813688975902,0.684121567187845,5.19523616882854));
#32235=CARTESIAN_POINT('Ctrl Pts',(11.8476896250997,0.672536043374578,5.05958779379219));
#32236=CARTESIAN_POINT('Ctrl Pts',(11.8858757940816,0.665865326892857,4.98148413049149));
#32237=CARTESIAN_POINT('Ctrl Pts',(11.922636015886,0.659397410760076,4.90402899576009));
#32238=CARTESIAN_POINT('Ctrl Pts',(11.9582263932854,0.653105260710028,4.82693636246589));
#32239=CARTESIAN_POINT('Ctrl Pts',(12.0138665013185,0.643268447106797,4.70641382917198));
#32240=CARTESIAN_POINT('Ctrl Pts',(12.0666476079204,0.633858069994158,4.58677779179511));
#32241=CARTESIAN_POINT('Ctrl Pts',(12.1173228696912,0.62473393238632,4.46626573472694));
#32242=CARTESIAN_POINT('Ctrl Pts',(12.1553590195886,0.617885481019554,4.37581105315446));
#32243=CARTESIAN_POINT('Ctrl Pts',(12.1922087795171,0.611199318424728,4.28486276143975));
#32244=CARTESIAN_POINT('Ctrl Pts',(12.228190632975,0.604635414006047,4.19267444498864));
#32245=CARTESIAN_POINT('Ctrl Pts',(12.3030650772989,0.590976620789059,4.00084027570298));
#32246=CARTESIAN_POINT('Ctrl Pts',(12.3741800556164,0.577857432420985,3.8036351343973));
#32247=CARTESIAN_POINT('Ctrl Pts',(12.4404245679778,0.565505899387503,3.60230507783802));
#32248=CARTESIAN_POINT('Ctrl Pts',(12.4484277147215,0.56401368323476,3.57798194631935));
#32249=CARTESIAN_POINT('Ctrl Pts',(12.4563597741263,0.562532608961203,3.5535986150842));
#32250=CARTESIAN_POINT('Ctrl Pts',(12.464218787137,0.561063026203705,3.52915728605649));
#32251=CARTESIAN_POINT('Ctrl Pts',(12.5124093904619,0.552051706382368,3.37928574489733));
#32252=CARTESIAN_POINT('Ctrl Pts',(12.5578532049559,0.543476675480936,3.22723289499543));
#32253=CARTESIAN_POINT('Ctrl Pts',(12.6001398201956,0.535458492472166,3.0744237536238));
#32254=CARTESIAN_POINT('Ctrl Pts',(12.621831189404,0.531345480185951,2.99603867869846));
#32255=CARTESIAN_POINT('Ctrl Pts',(12.6426918091358,0.527378158798193,2.91745465204444));
#32256=CARTESIAN_POINT('Ctrl Pts',(12.6626662843985,0.523567463387693,2.83886428776322));
#32257=CARTESIAN_POINT('Ctrl Pts',(12.7215803462743,0.512327941835709,2.60706457722144));
#32258=CARTESIAN_POINT('Ctrl Pts',(12.7727864647236,0.502444177432,2.3752102436452));
#32259=CARTESIAN_POINT('Ctrl Pts',(12.8167780306484,0.493907647680068,2.14242044261879));
#32260=CARTESIAN_POINT('Ctrl Pts',(12.8607695965732,0.485371117928113,1.90963064159175));
#32261=CARTESIAN_POINT('Ctrl Pts',(12.8975465474492,0.478183617519471,1.67590541472795));
#32262=CARTESIAN_POINT('Ctrl Pts',(12.9271424461252,0.472377045483412,1.44075450338083));
#32263=CARTESIAN_POINT('Ctrl Pts',(12.9567383448012,0.466570473447369,1.20560359203433));
#32264=CARTESIAN_POINT('Ctrl Pts',(12.9791530291776,0.462149468731758,0.96902683662872));
#32265=CARTESIAN_POINT('Ctrl Pts',(12.9942386480785,0.459169239074605,0.73151377154081));
#32266=CARTESIAN_POINT('Ctrl Pts',(13.0082305889908,0.456405070263105,0.511219941075852));
#32267=CARTESIAN_POINT('Ctrl Pts',(13.0159175203803,0.454882747634876,0.290120603906445));
#32268=CARTESIAN_POINT('Ctrl Pts',(13.0172425512059,0.4546204544462,0.0692015228525397));
#32269=CARTESIAN_POINT('Ctrl Pts',(13.017346122044,0.454599952337965,0.0519334156099304));
#32270=CARTESIAN_POINT('Ctrl Pts',(13.017410823298,0.454587122295236,0.0346664098812243));
#32271=CARTESIAN_POINT('Ctrl Pts',(13.0174366277985,0.454581959570064,0.0174009764857553));
#32272=CARTESIAN_POINT('Ctrl Pts',(13.0177440857389,0.454520446236328,-0.18831486759474));
#32273=CARTESIAN_POINT('Ctrl Pts',(13.0125295252215,0.455551756192601,-0.393807569883898));
#32274=CARTESIAN_POINT('Ctrl Pts',(13.0019394769544,0.45764683830302,-0.598013646668176));
#32275=CARTESIAN_POINT('Ctrl Pts',(13.0002697828882,0.457977162214662,-0.630210069772016));
#32276=CARTESIAN_POINT('Ctrl Pts',(12.9984664613338,0.458333824773382,-0.662374510521939));
#32277=CARTESIAN_POINT('Ctrl Pts',(12.9965300866001,0.458716594295993,-0.694502802839669));
#32278=CARTESIAN_POINT('Ctrl Pts',(12.9823122392856,0.461527082645403,-0.930405051873085));
#32279=CARTESIAN_POINT('Ctrl Pts',(12.9609214508078,0.465744725558995,-1.16435847740544));
#32280=CARTESIAN_POINT('Ctrl Pts',(12.9326414173885,0.471297941890548,-1.39637104020632));
#32281=CARTESIAN_POINT('Ctrl Pts',(12.9043613839692,0.476851158222116,-1.62838360300783));
#32282=CARTESIAN_POINT('Ctrl Pts',(12.869192221051,0.48373663979444,-1.85845528305323));
#32283=CARTESIAN_POINT('Ctrl Pts',(12.82705600053,0.491912777488324,-2.08731283346696));
#32284=CARTESIAN_POINT('Ctrl Pts',(12.7998529196691,0.497191279738091,-2.23506292525406));
#32285=CARTESIAN_POINT('Ctrl Pts',(12.7697455696918,0.503013587051361,-2.38230669762676));
#32286=CARTESIAN_POINT('Ctrl Pts',(12.7371408773064,0.509290643047791,-2.52753835000035));
#32287=CARTESIAN_POINT('Ctrl Pts',(12.7192425213279,0.512736434880241,-2.60726331053068));
#32288=CARTESIAN_POINT('Ctrl Pts',(12.7005916000993,0.516318323710831,-2.68638196014036));
#32289=CARTESIAN_POINT('Ctrl Pts',(12.6812554291551,0.520014935422878,-2.76464550962589));
#32290=CARTESIAN_POINT('Ctrl Pts',(12.648171622478,0.526339765069595,-2.89855289741836));
#32291=CARTESIAN_POINT('Ctrl Pts',(12.6130816730533,0.533003982417723,-3.02995702677085));
#32292=CARTESIAN_POINT('Ctrl Pts',(12.5769266936441,0.539847245472529,-3.15699014733577));
#32293=CARTESIAN_POINT('Ctrl Pts',(12.5534567855764,0.544289531359666,-3.23945335738117));
#32294=CARTESIAN_POINT('Ctrl Pts',(12.5295380821316,0.5488060716748,-3.32007471391683));
#32295=CARTESIAN_POINT('Ctrl Pts',(12.5054280206103,0.55334139293425,-3.39834398359222));
#32296=CARTESIAN_POINT('Ctrl Pts',(12.4687205620638,0.560246398837261,-3.51750858918807));
#32297=CARTESIAN_POINT('Ctrl Pts',(12.4315703607089,0.567188752539699,-3.63122182488701));
#32298=CARTESIAN_POINT('Ctrl Pts',(12.3938089815623,0.574190012215269,-3.74118823375633));
#32299=CARTESIAN_POINT('Ctrl Pts',(12.368560570584,0.578871268187638,-3.81471513207661));
#32300=CARTESIAN_POINT('Ctrl Pts',(12.3430389223144,0.583580059796604,-3.88656691042724));
#32301=CARTESIAN_POINT('Ctrl Pts',(12.3171936877466,0.588335665706033,-3.95725256130275));
#32302=CARTESIAN_POINT('Ctrl Pts',(12.2775531412705,0.595629653175207,-4.06566782143062));
#32303=CARTESIAN_POINT('Ctrl Pts',(12.2371513505869,0.603031170835373,-4.17133971598129));
#32304=CARTESIAN_POINT('Ctrl Pts',(12.1952061173948,0.610646478849638,-4.27627436264688));
#32305=CARTESIAN_POINT('Ctrl Pts',(12.1689021701395,0.615422055121253,-4.34207910852818));
#32306=CARTESIAN_POINT('Ctrl Pts',(12.1419912530875,0.620282768963302,-4.40759387782947));
#32307=CARTESIAN_POINT('Ctrl Pts',(12.1142804664268,0.625265210514748,-4.47331283655918));
#32308=CARTESIAN_POINT('Ctrl Pts',(12.0562410432107,0.635700787006872,-4.61095925222215));
#32309=CARTESIAN_POINT('Ctrl Pts',(11.994691828576,0.646677474596912,-4.7495001552316));
#32310=CARTESIAN_POINT('Ctrl Pts',(11.9300997334008,0.658068155383965,-4.88738150812178));
#32311=CARTESIAN_POINT('Ctrl Pts',(11.9146749410023,0.660788285237967,-4.92030800227241));
#32312=CARTESIAN_POINT('Ctrl Pts',(11.8990766225005,0.663531790474695,-4.95319690039001));
#32313=CARTESIAN_POINT('Ctrl Pts',(11.8833111363837,0.666296501523348,-4.98602707097243));
#32314=CARTESIAN_POINT('Ctrl Pts',(11.8071085671664,0.679659748523099,-5.14471189221277));
#32315=CARTESIAN_POINT('Ctrl Pts',(11.7270006317851,0.693522497860122,-5.30202462303339));
#32316=CARTESIAN_POINT('Ctrl Pts',(11.6438303021589,0.707707201862831,-5.45656047599039));
#32317=CARTESIAN_POINT('Ctrl Pts',(11.637738243609,0.708746202762382,-5.4678799148877));
#32318=CARTESIAN_POINT('Ctrl Pts',(11.6316297544981,0.709786908025164,-5.47918445706611));
#32319=CARTESIAN_POINT('Ctrl Pts',(11.6255051661099,0.71082923706868,-5.49047355140247));
#32320=CARTESIAN_POINT('Ctrl Pts',(11.5427080596109,0.724920278515558,-5.64308859861901));
#32321=CARTESIAN_POINT('Ctrl Pts',(11.456969029483,0.739303729464966,-5.79288102087204));
#32322=CARTESIAN_POINT('Ctrl Pts',(11.3675110472172,0.754054902312731,-5.94123279739961));
#32323=CARTESIAN_POINT('Ctrl Pts',(11.3600106655584,0.755291677650948,-5.95367098251773));
#32324=CARTESIAN_POINT('Ctrl Pts',(11.3524841412791,0.756531068057714,-5.96609903864255));
#32325=CARTESIAN_POINT('Ctrl Pts',(11.344931016417,0.757773134344475,-5.97851777921996));
#32326=CARTESIAN_POINT('Ctrl Pts',(11.2472908345613,0.773829479278541,-6.1390563788767));
#32327=CARTESIAN_POINT('Ctrl Pts',(11.1452052591543,0.790331519802546,-6.29803809444874));
#32328=CARTESIAN_POINT('Ctrl Pts',(11.0381645105898,0.807279061880735,-6.45590173342379));
#32329=CARTESIAN_POINT('Ctrl Pts',(10.9527885590251,0.820796461105002,-6.58181414132203));
#32330=CARTESIAN_POINT('Ctrl Pts',(10.8642604824445,0.834593931277089,-6.70701582823341));
#32331=CARTESIAN_POINT('Ctrl Pts',(10.7709807835768,0.848846921844718,-6.83319338638121));
#32332=CARTESIAN_POINT('Ctrl Pts',(10.7473103505908,0.852463726596192,-6.86521190134991));
#32333=CARTESIAN_POINT('Ctrl Pts',(10.7233339467609,0.856110123852281,-6.89729323502642));
#32334=CARTESIAN_POINT('Ctrl Pts',(10.6990254359918,0.859789513944065,-6.92946490307854));
#32335=CARTESIAN_POINT('Ctrl Pts',(10.5850549505516,0.877040339338839,-7.08030181201762));
#32336=CARTESIAN_POINT('Ctrl Pts',(10.463783904636,0.89501248721515,-7.23312447129108));
#32337=CARTESIAN_POINT('Ctrl Pts',(10.3326853170014,0.913883868715835,-7.38923986896025));
#32338=CARTESIAN_POINT('Ctrl Pts',(10.3256314894953,0.914899253185713,-7.39763973890598));
#32339=CARTESIAN_POINT('Ctrl Pts',(10.3185492109234,0.915917253547585,-7.4060491405237));
#32340=CARTESIAN_POINT('Ctrl Pts',(10.3114380876608,0.916937901851917,-7.41446827707697));
#32341=CARTESIAN_POINT('Ctrl Pts',(10.1793867030325,0.935891028781202,-7.57080906856405));
#32342=CARTESIAN_POINT('Ctrl Pts',(10.0373886982746,0.955753002911298,-7.73050708899526));
#32343=CARTESIAN_POINT('Ctrl Pts',(9.88185937375011,0.976697895521333,-7.89472729852672));
#32344=CARTESIAN_POINT('Ctrl Pts',(9.87335193950286,0.977843578480096,-7.9037101230772));
#32345=CARTESIAN_POINT('Ctrl Pts',(9.86480401851754,0.978992514653285,-7.9127064776283));
#32346=CARTESIAN_POINT('Ctrl Pts',(9.85621502410006,0.980144737119588,-7.92171655257824));
#32347=CARTESIAN_POINT('Ctrl Pts',(9.72378544070834,0.997910302419819,-8.06063857463946));
#32348=CARTESIAN_POINT('Ctrl Pts',(9.58159108396503,1.01646125094447,-8.20282124730524));
#32349=CARTESIAN_POINT('Ctrl Pts',(9.42910813639904,1.03558869639302,-8.34671638294721));
#32350=CARTESIAN_POINT('Ctrl Pts',(9.39090404965467,1.04038101315223,-8.38276882246198));
#32351=CARTESIAN_POINT('Ctrl Pts',(9.35205411094768,1.04520926624713,-8.41892879285433));
#32352=CARTESIAN_POINT('Ctrl Pts',(9.31255008182614,1.05006965587323,-8.45517201403564));
#32353=CARTESIAN_POINT('',(8.97637719778905,1.06099093965794,8.58635258519147));
#32354=CARTESIAN_POINT('Ctrl Pts',(8.97637719778914,1.06099093965548,8.58635258519167));
#32355=CARTESIAN_POINT('Ctrl Pts',(9.00588346338826,1.06203710363627,8.58635283430845));
#32356=CARTESIAN_POINT('Ctrl Pts',(9.03507097655644,1.0626130135361,8.58373842531847));
#32357=CARTESIAN_POINT('Ctrl Pts',(9.0639558049948,1.06272750014265,8.57854965874974));
#32358=CARTESIAN_POINT('Ctrl Pts',(9.09284063634256,1.06284198676072,8.57336089165838));
#32359=CARTESIAN_POINT('Ctrl Pts',(9.12142278435739,1.06249500887076,8.56559777366992));
#32360=CARTESIAN_POINT('Ctrl Pts',(9.14965453611679,1.06165426531512,8.55506327251998));
#32361=CARTESIAN_POINT('Ctrl Pts',(9.1778862878762,1.06081352175948,8.54452877137005));
#32362=CARTESIAN_POINT('Ctrl Pts',(9.20576764744961,1.05947889774048,8.53122290709537));
#32363=CARTESIAN_POINT('Ctrl Pts',(9.23305292402205,1.05757790867323,8.51473702651423));
#32364=CARTESIAN_POINT('Ctrl Pts',(9.26033820059449,1.05567691960598,8.4982511459331));
#32365=CARTESIAN_POINT('Ctrl Pts',(9.28702740061108,1.05320938365932,8.47858528069288));
#32366=CARTESIAN_POINT('Ctrl Pts',(9.31255008182614,1.05006965587323,8.45517201403565));
#32367=CARTESIAN_POINT('',(3.597021417327,0.8702239620615,8.586024047651));
#32368=CARTESIAN_POINT('Ctrl Pts',(3.470944033211,1.387996652244,8.999136656895));
#32369=CARTESIAN_POINT('Ctrl Pts',(3.506806407087,1.389267971531,8.999136656895));
#32370=CARTESIAN_POINT('Ctrl Pts',(4.139999211345,1.41171464956,8.999136656895));
#32371=CARTESIAN_POINT('Ctrl Pts',(5.370898212047,1.455350900996,8.999136656895));
#32372=CARTESIAN_POINT('Ctrl Pts',(7.164016762305,1.518920709268,8.999136656895));
#32373=CARTESIAN_POINT('Ctrl Pts',(8.39566724421,1.562587003558,8.999136656895));
#32374=CARTESIAN_POINT('Ctrl Pts',(9.029611555595,1.585063001874,8.999136656895));
#32375=CARTESIAN_POINT('Ctrl Pts',(9.065473930934,1.586334475758,8.999136656895));
#32376=CARTESIAN_POINT('Ctrl Pts',(3.480853549823,1.108461217464,9.015595309496));
#32377=CARTESIAN_POINT('Ctrl Pts',(3.516715931365,1.109732537023,9.015595309496));
#32378=CARTESIAN_POINT('Ctrl Pts',(4.149908870976,1.13217921985,9.015595309496));
#32379=CARTESIAN_POINT('Ctrl Pts',(5.380808135343,1.175815480634,9.015595309496));
#32380=CARTESIAN_POINT('Ctrl Pts',(7.173927071209,1.239385302576,9.015595309496));
#32381=CARTESIAN_POINT('Ctrl Pts',(8.405577819023,1.283051606293,9.015595309496));
#32382=CARTESIAN_POINT('Ctrl Pts',(9.03952226756,1.305527609472,9.015595309496));
#32383=CARTESIAN_POINT('Ctrl Pts',(9.075384650659,1.306799083631,9.015595309496));
#32384=CARTESIAN_POINT('Ctrl Pts',(3.488452624763,0.8941005377045,8.835315254871));
#32385=CARTESIAN_POINT('Ctrl Pts',(3.524315012182,0.8953718574718,8.835315254871));
#32386=CARTESIAN_POINT('Ctrl Pts',(4.157508055588,0.9178185439784,8.835315254871));
#32387=CARTESIAN_POINT('Ctrl Pts',(5.388407522147,0.9614548119297,8.835315254871));
#32388=CARTESIAN_POINT('Ctrl Pts',(7.181526753714,1.025024644355,8.835315254871));
#32389=CARTESIAN_POINT('Ctrl Pts',(8.413177705439,1.068690955302,8.835315254871));
#32390=CARTESIAN_POINT('Ctrl Pts',(9.047122259151,1.09116696221,8.835315254871));
#32391=CARTESIAN_POINT('Ctrl Pts',(9.0829846482,1.092438436579,8.835315254871));
#32392=CARTESIAN_POINT('Ctrl Pts',(3.489583140862,0.8622100508379,8.556943446236));
#32393=CARTESIAN_POINT('Ctrl Pts',(3.525445529156,0.8634813706362,8.556943446236));
#32394=CARTESIAN_POINT('Ctrl Pts',(4.158638588003,0.8859280576902,8.556943446236));
#32395=CARTESIAN_POINT('Ctrl Pts',(5.389538084642,0.9295643267078,8.556943446236));
#32396=CARTESIAN_POINT('Ctrl Pts',(7.182657360201,0.9931341606926,8.556943446236));
#32397=CARTESIAN_POINT('Ctrl Pts',(8.414308342262,1.036800472715,8.556943446236));
#32398=CARTESIAN_POINT('Ctrl Pts',(9.048252911621,1.059276480178,8.556943446236));
#32399=CARTESIAN_POINT('Ctrl Pts',(9.084115301555,1.060547954579,8.556943446236));
#32400=CARTESIAN_POINT('',(8.95892745008388,1.55316848628071,8.99999999999969));
#32401=CARTESIAN_POINT('',(3.579571669199,1.362459037518,9.));
#32402=CARTESIAN_POINT('Origin',(8.95892745079,1.553168486242,8.499999999999));
#32403=CARTESIAN_POINT('Origin',(3.002221399786,0.,9.));
#32404=CARTESIAN_POINT('',(8.958927440406,6.046831514125,9.));
#32405=CARTESIAN_POINT('',(8.958927440406,6.046831514125,9.));
#32406=CARTESIAN_POINT('',(8.958927440406,6.046831514125,9.));
#32407=CARTESIAN_POINT('Ctrl Pts',(9.065473909596,6.013665524999,8.999136656895));
#32408=CARTESIAN_POINT('Ctrl Pts',(9.02961154137,6.01493699863,8.999136656895));
#32409=CARTESIAN_POINT('Ctrl Pts',(8.3956669983,6.037413005161,8.999136656895));
#32410=CARTESIAN_POINT('Ctrl Pts',(7.164016284709,6.081079307665,8.999136656895));
#32411=CARTESIAN_POINT('Ctrl Pts',(5.370897734451,6.144649115935,8.999136656895));
#32412=CARTESIAN_POINT('Ctrl Pts',(4.139998972687,6.1882853589,8.999136656895));
#32413=CARTESIAN_POINT('Ctrl Pts',(3.506806407366,6.210732028459,8.999136656895));
#32414=CARTESIAN_POINT('Ctrl Pts',(3.470944033629,6.212003347741,8.999136656895));
#32415=CARTESIAN_POINT('Ctrl Pts',(9.07538462932,6.293200917125,9.015595309496));
#32416=CARTESIAN_POINT('Ctrl Pts',(9.039522253334,6.294472391032,9.015595309496));
#32417=CARTESIAN_POINT('Ctrl Pts',(8.405577573112,6.316948402425,9.015595309496));
#32418=CARTESIAN_POINT('Ctrl Pts',(7.173926593613,6.360614714356,9.015595309496));
#32419=CARTESIAN_POINT('Ctrl Pts',(5.380807657748,6.424184536297,9.015595309496));
#32420=CARTESIAN_POINT('Ctrl Pts',(4.149908632317,6.46782078861,9.015595309496));
#32421=CARTESIAN_POINT('Ctrl Pts',(3.516715931643,6.490267462967,9.015595309496));
#32422=CARTESIAN_POINT('Ctrl Pts',(3.480853550242,6.491538782521,9.015595309496));
#32423=CARTESIAN_POINT('Ctrl Pts',(9.082984626861,6.507561564177,8.835315254871));
#32424=CARTESIAN_POINT('Ctrl Pts',(9.047122244925,6.508833038295,8.835315254871));
#32425=CARTESIAN_POINT('Ctrl Pts',(8.413177459528,6.531309053417,8.835315254871));
#32426=CARTESIAN_POINT('Ctrl Pts',(7.181526276118,6.574975372577,8.835315254871));
#32427=CARTESIAN_POINT('Ctrl Pts',(5.388407044551,6.638545205002,8.835315254871));
#32428=CARTESIAN_POINT('Ctrl Pts',(4.157507816929,6.682181464482,8.835315254872));
#32429=CARTESIAN_POINT('Ctrl Pts',(3.524315012461,6.704628142518,8.835315254871));
#32430=CARTESIAN_POINT('Ctrl Pts',(3.488452625181,6.705899462281,8.835315254871));
#32431=CARTESIAN_POINT('Ctrl Pts',(9.084115280216,6.539452046178,8.556943446236));
#32432=CARTESIAN_POINT('Ctrl Pts',(9.048252897395,6.540723520327,8.556943446236));
#32433=CARTESIAN_POINT('Ctrl Pts',(8.414308096351,6.563199536004,8.556943446236));
#32434=CARTESIAN_POINT('Ctrl Pts',(7.182656882606,6.60686585624,8.556943446236));
#32435=CARTESIAN_POINT('Ctrl Pts',(5.389537607047,6.670435690223,8.556943446236));
#32436=CARTESIAN_POINT('Ctrl Pts',(4.158638349345,6.71407195077,8.556943446236));
#32437=CARTESIAN_POINT('Ctrl Pts',(3.525445529435,6.736518629354,8.556943446236));
#32438=CARTESIAN_POINT('Ctrl Pts',(3.489583141281,6.737789949147,8.556943446236));
#32439=CARTESIAN_POINT('',(8.976377188873,6.539009060657,8.586352585191));
#32440=CARTESIAN_POINT('Origin',(8.958927440522,6.046831514122,8.5));
#32441=CARTESIAN_POINT('',(8.976377188873,6.539009060657,8.586352585191));
#32442=CARTESIAN_POINT('Origin',(6.513075547481,-42.4,0.));
#32443=CARTESIAN_POINT('',(0.01744974833006,7.599368653176,-0.04689126965526));
#32444=CARTESIAN_POINT('Ctrl Pts',(0.01744974833006,7.599368653176,-0.04689126965526));
#32445=CARTESIAN_POINT('Ctrl Pts',(0.067537433307,7.597493189218,-0.1814388238612));
#32446=CARTESIAN_POINT('Ctrl Pts',(0.1639979857046,7.592799454319,-0.4404924525001));
#32447=CARTESIAN_POINT('Ctrl Pts',(0.2891401437734,7.583879367514,-0.8017214821274));
#32448=CARTESIAN_POINT('Ctrl Pts',(0.3899548010611,7.573764858792,-1.138584886082));
#32449=CARTESIAN_POINT('Ctrl Pts',(0.4632860851713,7.563044638479,-1.451600247463));
#32450=CARTESIAN_POINT('Ctrl Pts',(0.5076215437038,7.552188980092,-1.74099111528));
#32451=CARTESIAN_POINT('Ctrl Pts',(0.5174627880836,7.545233335246,-1.917359950681));
#32452=CARTESIAN_POINT('Ctrl Pts',(0.5174549507661,7.541860021273,-2.001305923414));
#32453=CARTESIAN_POINT('',(0.0174497466342403,7.59936861534601,0.0468912686245114));
#32454=CARTESIAN_POINT('Ctrl Pts',(0.0174497479590823,7.59936865318618,
0.0468912686587025));
#32455=CARTESIAN_POINT('Ctrl Pts',(0.0157883609905255,7.59943085569528,
0.0424282636034863));
#32456=CARTESIAN_POINT('Ctrl Pts',(0.0143880925278573,7.59948328325758,
0.0380261499363122));
#32457=CARTESIAN_POINT('Ctrl Pts',(0.013231809680605,7.59952657327597,0.0337070287048825));
#32458=CARTESIAN_POINT('Ctrl Pts',(0.0120755267436379,7.59956986329772,
0.0293879071383306));
#32459=CARTESIAN_POINT('Ctrl Pts',(0.0111632296353382,7.59960402079665,
0.0251517780061871));
#32460=CARTESIAN_POINT('Ctrl Pts',(0.0104662607819539,7.59963011599904,
0.0209620713759419));
#32461=CARTESIAN_POINT('Ctrl Pts',(0.00976929192856706,7.59965621120143,
0.0167723647456966));
#32462=CARTESIAN_POINT('Ctrl Pts',(0.00928765138822166,7.59967424577191,
0.0126290806250674));
#32463=CARTESIAN_POINT('Ctrl Pts',(0.00900722076910609,7.59968474284106,
0.00847390165808531));
#32464=CARTESIAN_POINT('Ctrl Pts',(0.00872679014999053,7.59969523991021,
0.00431872269110327));
#32465=CARTESIAN_POINT('Ctrl Pts',(0.00864756965336628,7.59969820524141,
0.000151648877503578));
#32466=CARTESIAN_POINT('Ctrl Pts',(0.00879065645843391,7.59969285107069,
-0.00415254496086243));
#32467=CARTESIAN_POINT('Ctrl Pts',(0.00893374326350403,7.59968749689997,
-0.00845673879921733));
#32468=CARTESIAN_POINT('Ctrl Pts',(0.00929913705893244,7.59967381431182,
-0.0128980526607187));
#32469=CARTESIAN_POINT('Ctrl Pts',(0.00993647955041976,7.59964995114117,
-0.0174909161469611));
#32470=CARTESIAN_POINT('Ctrl Pts',(0.0105738220419093,7.59962608797053,
-0.0220837796332035));
#32471=CARTESIAN_POINT('Ctrl Pts',(0.0114831132109058,7.59959204368608,
-0.0268281927446774));
#32472=CARTESIAN_POINT('Ctrl Pts',(0.012718653611351,7.59954578593001,-0.0317313795031946));
#32473=CARTESIAN_POINT('Ctrl Pts',(0.0139541940117949,7.59949952817393,
-0.0366345662617119));
#32474=CARTESIAN_POINT('Ctrl Pts',(0.0155159835261466,7.59944105358036,
-0.0416965266648994));
#32475=CARTESIAN_POINT('Ctrl Pts',(0.0174497483299296,7.59936865317228,
-0.0468912696552633));
#32476=CARTESIAN_POINT('Ctrl Pts',(0.5174542977566,7.541857836025,2.00131664892));
#32477=CARTESIAN_POINT('Ctrl Pts',(0.5174639416778,7.545246037484,1.917084695768));
#32478=CARTESIAN_POINT('Ctrl Pts',(0.5075557516817,7.552220151835,1.740184484561));
#32479=CARTESIAN_POINT('Ctrl Pts',(0.4629797196809,7.563104735101,1.449958596358));
#32480=CARTESIAN_POINT('Ctrl Pts',(0.3893196154358,7.573844231286,1.1361637114));
#32481=CARTESIAN_POINT('Ctrl Pts',(0.2880099327634,7.583976642822,0.798235513827));
#32482=CARTESIAN_POINT('Ctrl Pts',(0.1627480055576,7.592869536741,0.4370888248364));
#32483=CARTESIAN_POINT('Ctrl Pts',(0.06701238076274,7.597512638594,0.1800461148998));
#32484=CARTESIAN_POINT('Ctrl Pts',(0.01744974438142,7.599368539647,0.04689126959107));
#32485=CARTESIAN_POINT('',(9.31255006808369,6.54993034244276,8.45517202657257));
#32486=CARTESIAN_POINT('Ctrl Pts',(9.31255006811848,6.54993034243673,8.45517202660968));
#32487=CARTESIAN_POINT('Ctrl Pts',(9.29078297542864,6.54725259653745,8.47514021267117));
#32488=CARTESIAN_POINT('Ctrl Pts',(9.24421410184042,6.5427099915477,8.51085124868992));
#32489=CARTESIAN_POINT('Ctrl Pts',(9.165144091791,6.538346690073,8.551938784869));
#32490=CARTESIAN_POINT('Ctrl Pts',(9.076493701984,6.536708784041,8.579235860742));
#32491=CARTESIAN_POINT('Ctrl Pts',(9.010833592703,6.537787400757,8.586352779966));
#32492=CARTESIAN_POINT('Ctrl Pts',(8.976377188873,6.539009060657,8.586352585191));
#32493=CARTESIAN_POINT('',(9.312550081826,6.549930344123,-8.455172014035));
#32494=CARTESIAN_POINT('Ctrl Pts',(9.31255008182585,6.54993034411883,-8.45517201403428));
#32495=CARTESIAN_POINT('Ctrl Pts',(9.49006778755429,6.57177150512728,-8.29230600605519));
#32496=CARTESIAN_POINT('Ctrl Pts',(9.65650776248302,6.59321615075835,-8.12919896342003));
#32497=CARTESIAN_POINT('Ctrl Pts',(9.81264940133939,6.61403129349834,-7.96715940976441));
#32498=CARTESIAN_POINT('Ctrl Pts',(9.91032159555209,6.62705191169574,-7.86579785835051));
#32499=CARTESIAN_POINT('Ctrl Pts',(10.0039641012073,6.63982725131886,-7.76485417052757));
#32500=CARTESIAN_POINT('Ctrl Pts',(10.0937676900692,6.65231053633801,-7.6646501042644));
#32501=CARTESIAN_POINT('Ctrl Pts',(10.327133934128,6.68474996749384,-7.40425687410953));
#32502=CARTESIAN_POINT('Ctrl Pts',(10.5345775074028,6.71522144323954,-7.14885927793018));
#32503=CARTESIAN_POINT('Ctrl Pts',(10.7222455610682,6.74373128167272,-6.89862060649505));
#32504=CARTESIAN_POINT('Ctrl Pts',(10.8809434226423,6.76784007539014,-6.6870111116223));
#32505=CARTESIAN_POINT('Ctrl Pts',(11.0254997683209,6.79054170685715,-6.47909014035725));
#32506=CARTESIAN_POINT('Ctrl Pts',(11.1576842327289,6.81178273634758,-6.27604679436481));
#32507=CARTESIAN_POINT('Ctrl Pts',(11.1818144212986,6.81566027255665,-6.23898136274571));
#32508=CARTESIAN_POINT('Ctrl Pts',(11.2055323259985,6.81948927456683,-6.20207848992696));
#32509=CARTESIAN_POINT('Ctrl Pts',(11.2288487120883,6.82326959994322,-6.16534542921002));
#32510=CARTESIAN_POINT('Ctrl Pts',(11.3798915764977,6.84775843672311,-5.92738974054291));
#32511=CARTESIAN_POINT('Ctrl Pts',(11.5140851958374,6.87019999476148,-5.69655946408425));
#32512=CARTESIAN_POINT('Ctrl Pts',(11.6342642086962,6.89066182319112,-5.47430110068892));
#32513=CARTESIAN_POINT('Ctrl Pts',(11.7106680870889,6.90367044269832,-5.33300021491302));
#32514=CARTESIAN_POINT('Ctrl Pts',(11.7814080028223,6.9158851657,-5.19516484270745));
#32515=CARTESIAN_POINT('Ctrl Pts',(11.8478285723651,6.92748831032456,-5.059302800753));
#32516=CARTESIAN_POINT('Ctrl Pts',(11.8858838311325,6.93413626101579,-4.98146147540998));
#32517=CARTESIAN_POINT('Ctrl Pts',(11.9225212010676,6.94058246134619,-4.90426784694912));
#32518=CARTESIAN_POINT('Ctrl Pts',(11.9579935739301,6.94685356935787,-4.82744073960209));
#32519=CARTESIAN_POINT('Ctrl Pts',(12.0136308210525,6.95668959548248,-4.70693995512574));
#32520=CARTESIAN_POINT('Ctrl Pts',(12.0664022350456,6.96609804028853,-4.58734137006994));
#32521=CARTESIAN_POINT('Ctrl Pts',(12.1170636741229,6.97521944844119,-4.46688154635999));
#32522=CARTESIAN_POINT('Ctrl Pts',(12.1550776589322,6.98206372837619,-4.37649410391776));
#32523=CARTESIAN_POINT('Ctrl Pts',(12.1919036639809,6.98874536971883,-4.28562167942354));
#32524=CARTESIAN_POINT('Ctrl Pts',(12.2278610179747,6.99530451591579,-4.19351816197963));
#32525=CARTESIAN_POINT('Ctrl Pts',(12.3036863575555,7.00913616459135,-3.99929417964824));
#32526=CARTESIAN_POINT('Ctrl Pts',(12.3756475796478,7.02241272830797,-3.79959416133987));
#32527=CARTESIAN_POINT('Ctrl Pts',(12.4426100541845,7.03490158145942,-3.59565695221801));
#32528=CARTESIAN_POINT('Ctrl Pts',(12.4497213980101,7.03622788442778,-3.57399903675229));
#32529=CARTESIAN_POINT('Ctrl Pts',(12.4567763648866,7.03754535193983,-3.55229333798136));
#32530=CARTESIAN_POINT('Ctrl Pts',(12.4637735958284,7.03885374058288,-3.5305413429469));
#32531=CARTESIAN_POINT('Ctrl Pts',(12.5119042445602,7.0478535284571,-3.38091963674243));
#32532=CARTESIAN_POINT('Ctrl Pts',(12.557302921659,7.05641954217032,-3.22910687206369));
#32533=CARTESIAN_POINT('Ctrl Pts',(12.5995564877654,7.06443093497975,-3.07653040949109));
#32534=CARTESIAN_POINT('Ctrl Pts',(12.6212883256478,7.06855135145082,-2.99805734189386));
#32535=CARTESIAN_POINT('Ctrl Pts',(12.6421882040919,7.07252589140287,-2.9193823077654));
#32536=CARTESIAN_POINT('Ctrl Pts',(12.6621999153949,7.07634349842331,-2.84069977527412));
#32537=CARTESIAN_POINT('Ctrl Pts',(12.7211207226989,7.08758374090974,-2.60903351420746));
#32538=CARTESIAN_POINT('Ctrl Pts',(12.7723429523916,7.09747019371598,-2.37730275152345));
#32539=CARTESIAN_POINT('Ctrl Pts',(12.8163549825881,7.10601028713707,-2.14465728986177));
#32540=CARTESIAN_POINT('Ctrl Pts',(12.8603670127847,7.11455038055818,-1.91201182819948));
#32541=CARTESIAN_POINT('Ctrl Pts',(12.897168786403,7.12174247559519,-1.67845171591279));
#32542=CARTESIAN_POINT('Ctrl Pts',(12.9267985558583,7.12755549034134,-1.44348407101859));
#32543=CARTESIAN_POINT('Ctrl Pts',(12.9564283253135,7.13336850508748,-1.20851642612503));
#32544=CARTESIAN_POINT('Ctrl Pts',(12.9788859304009,7.13779785482601,-0.972141090669652));
#32545=CARTESIAN_POINT('Ctrl Pts',(12.9940272207165,7.14078900135936,-0.734834418582472));
#32546=CARTESIAN_POINT('Ctrl Pts',(13.0081495807623,7.14357885925213,-0.513497254138357));
#32547=CARTESIAN_POINT('Ctrl Pts',(13.0159070855893,7.14511512893504,-0.291349846503961));
#32548=CARTESIAN_POINT('Ctrl Pts',(13.0172415248565,7.14537934085419,-0.0693735202517211));
#32549=CARTESIAN_POINT('Ctrl Pts',(13.0173378048379,7.14539840378144,-0.0533578969940196));
#32550=CARTESIAN_POINT('Ctrl Pts',(13.0174006486339,7.14541086733759,-0.0373431644940472));
#32551=CARTESIAN_POINT('Ctrl Pts',(13.0174300343815,7.14541673509063,-0.0213296913672406));
#32552=CARTESIAN_POINT('Ctrl Pts',(13.0178083424561,7.1454922757367,0.18482556027766));
#32553=CARTESIAN_POINT('Ctrl Pts',(13.0126413842003,7.14447031469605,0.390772161360061));
#32554=CARTESIAN_POINT('Ctrl Pts',(13.002072435279,7.14237940736248,0.595449151127796));
#32555=CARTESIAN_POINT('Ctrl Pts',(13.0004419032247,7.14205683115785,0.627025838182427));
#32556=CARTESIAN_POINT('Ctrl Pts',(12.9986827984263,7.14170891390931,0.658572308601473));
#32557=CARTESIAN_POINT('Ctrl Pts',(12.9967956469798,7.14133587053571,0.690084668584461));
#32558=CARTESIAN_POINT('Ctrl Pts',(12.98267616487,7.13854479658696,0.925857056562666));
#32559=CARTESIAN_POINT('Ctrl Pts',(12.96138904957,7.13434741615559,1.15972000730305));
#32560=CARTESIAN_POINT('Ctrl Pts',(12.9332147976316,7.12881461129494,1.39166038958121));
#32561=CARTESIAN_POINT('Ctrl Pts',(12.9050405456931,7.12328180643427,1.62360077185999));
#32562=CARTESIAN_POINT('Ctrl Pts',(12.8699792798543,7.11641709407502,1.85361857379828));
#32563=CARTESIAN_POINT('Ctrl Pts',(12.8279470458181,7.10826026606875,2.0824641655611));
#32564=CARTESIAN_POINT('Ctrl Pts',(12.8007150614312,7.10297559305513,2.23072941304998));
#32565=CARTESIAN_POINT('Ctrl Pts',(12.7705565767191,7.09714263522302,2.37850234504309));
#32566=CARTESIAN_POINT('Ctrl Pts',(12.7378726221699,7.0908498865513,2.5242836001386));
#32567=CARTESIAN_POINT('Ctrl Pts',(12.7201092935788,7.08742985479754,2.60351392499996));
#32568=CARTESIAN_POINT('Ctrl Pts',(12.7015999944259,7.08387493863183,2.68215598443196));
#32569=CARTESIAN_POINT('Ctrl Pts',(12.6824091040699,7.08020576750035,2.75996937505813));
#32570=CARTESIAN_POINT('Ctrl Pts',(12.6495024648307,7.0739142360242,2.89339607521678));
#32571=CARTESIAN_POINT('Ctrl Pts',(12.6145916946915,7.06728319522948,3.0243863246274));
#32572=CARTESIAN_POINT('Ctrl Pts',(12.5786086920348,7.06047129381164,3.15107197859204));
#32573=CARTESIAN_POINT('Ctrl Pts',(12.5549949651851,7.05600100596649,3.2342090212963));
#32574=CARTESIAN_POINT('Ctrl Pts',(12.5309194709636,7.05145403211695,3.31549230343964));
#32575=CARTESIAN_POINT('Ctrl Pts',(12.5066455815884,7.04688726462086,3.39439455486266));
#32576=CARTESIAN_POINT('Ctrl Pts',(12.4698582463404,7.03996628033685,3.51397174869596));
#32577=CARTESIAN_POINT('Ctrl Pts',(12.4326160731218,7.03300607735472,3.62808101585939));
#32578=CARTESIAN_POINT('Ctrl Pts',(12.3947586326729,7.02598632415325,3.73841820624057));
#32579=CARTESIAN_POINT('Ctrl Pts',(12.36957114144,7.02131590877062,3.81182826731294));
#32580=CARTESIAN_POINT('Ctrl Pts',(12.3441112978653,7.01661793652144,3.88356855430558));
#32581=CARTESIAN_POINT('Ctrl Pts',(12.3183318538247,7.01187380074364,3.95413799035498));
#32582=CARTESIAN_POINT('Ctrl Pts',(12.2787528679277,7.00459016488451,4.06248271298572));
#32583=CARTESIAN_POINT('Ctrl Pts',(12.2384205239071,6.99720034784702,4.16806748038133));
#32584=CARTESIAN_POINT('Ctrl Pts',(12.1965545931921,6.98959831045675,4.27289989604193));
#32585=CARTESIAN_POINT('Ctrl Pts',(12.1701654562908,6.9848065573058,4.33897837372818));
#32586=CARTESIAN_POINT('Ctrl Pts',(12.143167010936,6.97992941935173,4.40475788634172));
#32587=CARTESIAN_POINT('Ctrl Pts',(12.1153638613582,6.9749297741696,4.4707406291853));
#32588=CARTESIAN_POINT('Ctrl Pts',(12.057108107269,6.96445405092651,4.6089938306964));
#32589=CARTESIAN_POINT('Ctrl Pts',(11.9953185701516,6.95343331477605,4.74813799939895));
#32590=CARTESIAN_POINT('Ctrl Pts',(11.9304543037742,6.94199424071378,4.88662589555805));
#32591=CARTESIAN_POINT('Ctrl Pts',(11.9152484660004,6.93931263011078,4.91909098921037));
#32592=CARTESIAN_POINT('Ctrl Pts',(11.8998736555181,6.93660825499467,4.95152003275441));
#32593=CARTESIAN_POINT('Ctrl Pts',(11.8843357862834,6.93388316062605,4.98389312313398));
#32594=CARTESIAN_POINT('Ctrl Pts',(11.8086189668404,6.9206036385013,5.14164882322728));
#32595=CARTESIAN_POINT('Ctrl Pts',(11.7290301761305,6.90682801104577,5.29807576163209));
#32596=CARTESIAN_POINT('Ctrl Pts',(11.6464112725892,6.89273303439849,5.4517622729065));
#32597=CARTESIAN_POINT('Ctrl Pts',(11.6397533860299,6.89159718350298,5.46414717894979));
#32598=CARTESIAN_POINT('Ctrl Pts',(11.6330758218434,6.89045928657576,5.47651429096273));
#32599=CARTESIAN_POINT('Ctrl Pts',(11.6263790205946,6.88931945061147,5.48886287145605));
#32600=CARTESIAN_POINT('Ctrl Pts',(11.5435350300419,6.87521890374586,5.64162321893096));
#32601=CARTESIAN_POINT('Ctrl Pts',(11.4577474733856,6.8608259726941,5.79154821698368));
#32602=CARTESIAN_POINT('Ctrl Pts',(11.3682432763548,6.846065870727,5.94001812062533));
#32603=CARTESIAN_POINT('Ctrl Pts',(11.3607295496616,6.84482678501008,5.95248191914141));
#32604=CARTESIAN_POINT('Ctrl Pts',(11.3531896306147,6.84358508150389,5.96493546126059));
#32605=CARTESIAN_POINT('Ctrl Pts',(11.3456230618551,6.84234069947685,5.97737956249348));
#32606=CARTESIAN_POINT('Ctrl Pts',(11.2479228365551,6.82627312535388,6.13805893153611));
#32607=CARTESIAN_POINT('Ctrl Pts',(11.1457793596027,6.80976046367597,6.29716413816969));
#32608=CARTESIAN_POINT('Ctrl Pts',(11.0386838093546,6.79280313264702,6.45513601625609));
#32609=CARTESIAN_POINT('Ctrl Pts',(10.95324778463,6.77927533480954,6.58115889256326));
#32610=CARTESIAN_POINT('Ctrl Pts',(10.8646603995461,6.76546788162356,6.70646106814643));
#32611=CARTESIAN_POINT('Ctrl Pts',(10.7713246513584,6.7512056589261,6.83272795168484));
#32612=CARTESIAN_POINT('Ctrl Pts',(10.7476624078654,6.74758993619637,6.86473881356154));
#32613=CARTESIAN_POINT('Ctrl Pts',(10.723694981797,6.74394472515823,6.89681165784147));
#32614=CARTESIAN_POINT('Ctrl Pts',(10.6993963518299,6.74026664072237,6.92897390289576));
#32615=CARTESIAN_POINT('Ctrl Pts',(10.5856732127626,6.72305236533453,7.07950055694885));
#32616=CARTESIAN_POINT('Ctrl Pts',(10.4646950372019,6.70512194294707,7.23198551458773));
#32617=CARTESIAN_POINT('Ctrl Pts',(10.33394473404,6.68629743059677,7.38773991203805));
#32618=CARTESIAN_POINT('Ctrl Pts',(10.3265618155478,6.68523448973181,7.39653470633959));
#32619=CARTESIAN_POINT('Ctrl Pts',(10.319147739752,6.68416868431552,7.40533992386218));
#32620=CARTESIAN_POINT('Ctrl Pts',(10.3117020534887,6.68309997728696,7.41415580027921));
#32621=CARTESIAN_POINT('Ctrl Pts',(10.1797693680289,6.66416318848558,7.57036735812084));
#32622=CARTESIAN_POINT('Ctrl Pts',(10.0379117757277,6.64431961626695,7.72992583955895));
#32623=CARTESIAN_POINT('Ctrl Pts',(9.88255009909747,6.6233951338071,7.89399787690877));
#32624=CARTESIAN_POINT('Ctrl Pts',(9.87386552973313,6.62222547521898,7.90316934711957));
#32625=CARTESIAN_POINT('Ctrl Pts',(9.86513876411273,6.62105242549219,7.9123549200861));
#32626=CARTESIAN_POINT('Ctrl Pts',(9.85636917706876,6.61987594930949,7.92155479929637));
#32627=CARTESIAN_POINT('Ctrl Pts',(9.72396192532252,6.60211297172393,8.06045879973815));
#32628=CARTESIAN_POINT('Ctrl Pts',(9.58179259770183,6.5835647569172,8.20262298986108));
#32629=CARTESIAN_POINT('Ctrl Pts',(9.42933843780151,6.56444019510331,8.3464990344189));
#32630=CARTESIAN_POINT('Ctrl Pts',(9.39106011623076,6.55963838367691,8.38262355541271));
#32631=CARTESIAN_POINT('Ctrl Pts',(9.35213342239554,6.554800491868,8.41885602797014));
#32632=CARTESIAN_POINT('Ctrl Pts',(9.31255008182585,6.54993034411883,8.45517201403428));
#32633=CARTESIAN_POINT('',(8.9763771992842,6.53900906028642,-8.58635258519104));
#32634=CARTESIAN_POINT('Ctrl Pts',(8.9763771992841,6.53900906028359,-8.58635258519028));
#32635=CARTESIAN_POINT('Ctrl Pts',(9.00583001265153,6.53796479114675,-8.58635283579333));
#32636=CARTESIAN_POINT('Ctrl Pts',(9.03498268830907,6.53738830563828,-8.5837487457709));
#32637=CARTESIAN_POINT('Ctrl Pts',(9.06385871107003,6.53727288613592,-8.57856709206617));
#32638=CARTESIAN_POINT('Ctrl Pts',(9.09273473723344,6.53715746661995,-8.57338543775088));
#32639=CARTESIAN_POINT('Ctrl Pts',(9.12133411192538,6.53750315525565,-8.56562622650716));
#32640=CARTESIAN_POINT('Ctrl Pts',(9.14958717399502,6.53834372961078,-8.55508840261447));
#32641=CARTESIAN_POINT('Ctrl Pts',(9.17784023606467,6.53918430396591,-8.54455057872178));
#32642=CARTESIAN_POINT('Ctrl Pts',(9.20574698943828,6.54051987479979,-8.5312341615105));
#32643=CARTESIAN_POINT('Ctrl Pts',(9.23304466248228,6.54242151574695,-8.51474201807231));
#32644=CARTESIAN_POINT('Ctrl Pts',(9.26034233552627,6.54432315669411,-8.49824987463412));
#32645=CARTESIAN_POINT('Ctrl Pts',(9.2870309347497,6.54679105138876,-8.47858203692904));
#32646=CARTESIAN_POINT('Ctrl Pts',(9.31255008182585,6.54993034411882,-8.45517201403432));
#32647=CARTESIAN_POINT('',(3.597021417327,6.729776037938,-8.586024047651));
#32648=CARTESIAN_POINT('',(3.597021417327,6.729776037938,-8.586024047651));
#32649=CARTESIAN_POINT('Ctrl Pts',(3.16400873497919,6.78858150430047,-8.33346840037428));
#32650=CARTESIAN_POINT('Ctrl Pts',(3.18245003661732,6.78246267353839,-8.3657297019323));
#32651=CARTESIAN_POINT('Ctrl Pts',(3.20356756071657,6.77677099112735,-8.39472009582055));
#32652=CARTESIAN_POINT('Ctrl Pts',(3.22736110799477,6.77142291886836,-8.42102585955313));
#32653=CARTESIAN_POINT('Ctrl Pts',(3.25115466367853,6.76607484472005,-8.44733163257876));
#32654=CARTESIAN_POINT('Ctrl Pts',(3.27762421818746,6.76106964013681,-8.4709526470973));
#32655=CARTESIAN_POINT('Ctrl Pts',(3.30517534476285,6.75662306506702,-8.49104256326221));
#32656=CARTESIAN_POINT('Ctrl Pts',(3.33272647133824,6.75217648999722,-8.51113247942711));
#32657=CARTESIAN_POINT('Ctrl Pts',(3.36135919392955,6.74828922022634,-8.52769141414516));
#32658=CARTESIAN_POINT('Ctrl Pts',(3.39171144247602,6.7448188976879,-8.54146863707291));
#32659=CARTESIAN_POINT('Ctrl Pts',(3.42206369102248,6.74134857514947,-8.55524586000065));
#32660=CARTESIAN_POINT('Ctrl Pts',(3.45413545171913,6.73829481040069,-8.56624130320908));
#32661=CARTESIAN_POINT('Ctrl Pts',(3.48830827981827,6.73574096876752,-8.57393475975479));
#32662=CARTESIAN_POINT('Ctrl Pts',(3.52248110791741,6.73318712713436,-8.5816282163005));
#32663=CARTESIAN_POINT('Ctrl Pts',(3.55875500812843,6.73113334144666,-8.58601970949189));
#32664=CARTESIAN_POINT('Ctrl Pts',(3.59702141732687,6.72977603793439,-8.58602404765039));
#32665=CARTESIAN_POINT('Ctrl Pts',(2.697976245788,6.271708668204,-8.470478867963));
#32666=CARTESIAN_POINT('Ctrl Pts',(2.702496487236,6.270109776492,-8.478862059423));
#32667=CARTESIAN_POINT('Ctrl Pts',(2.741553495773,6.256704437972,-8.548825392175));
#32668=CARTESIAN_POINT('Ctrl Pts',(2.830094460866,6.232525054952,-8.670029259093));
#32669=CARTESIAN_POINT('Ctrl Pts',(2.985002282807,6.202729543589,-8.80802165731));
#32670=CARTESIAN_POINT('Ctrl Pts',(3.162329083555,6.1782271165,-8.910329310933));
#32671=CARTESIAN_POINT('Ctrl Pts',(3.360770749574,6.15933536047,-8.97640494805));
#32672=CARTESIAN_POINT('Ctrl Pts',(3.512848176858,6.150922384735,-8.993154038482));
#32673=CARTESIAN_POINT('Ctrl Pts',(3.596210811008,6.148187398446,-8.991916537819));
#32674=CARTESIAN_POINT('Ctrl Pts',(3.60609432629,6.147889718194,-8.991622140839));
#32675=CARTESIAN_POINT('Ctrl Pts',(2.707229788595,6.575168830057,-8.522615175531));
#32676=CARTESIAN_POINT('Ctrl Pts',(2.711757591597,6.573562734905,-8.531038953485));
#32677=CARTESIAN_POINT('Ctrl Pts',(2.750879945687,6.560097135082,-8.601341018487));
#32678=CARTESIAN_POINT('Ctrl Pts',(2.839569240021,6.535811141223,-8.72313186267));
#32679=CARTESIAN_POINT('Ctrl Pts',(2.99473765246,6.505889438864,-8.861792775667));
#32680=CARTESIAN_POINT('Ctrl Pts',(3.172364230425,6.481288731968,-8.96459655693));
#32681=CARTESIAN_POINT('Ctrl Pts',(3.371142968843,6.462327820356,-9.030993747717));
#32682=CARTESIAN_POINT('Ctrl Pts',(3.523479741901,6.453890770661,-9.047826127655));
#32683=CARTESIAN_POINT('Ctrl Pts',(3.606984714449,6.45115151872,-9.04658424048));
#32684=CARTESIAN_POINT('Ctrl Pts',(3.616885107666,6.450853459245,-9.046288614332));
#32685=CARTESIAN_POINT('Ctrl Pts',(2.911986675828,6.79469121972,-8.453506164382));
#32686=CARTESIAN_POINT('Ctrl Pts',(2.915517531542,6.793439346699,-8.460099530006));
#32687=CARTESIAN_POINT('Ctrl Pts',(2.94602445157,6.782944985081,-8.515123261411));
#32688=CARTESIAN_POINT('Ctrl Pts',(3.01515739146,6.764040432135,-8.610408211832));
#32689=CARTESIAN_POINT('Ctrl Pts',(3.135968450588,6.740798929991,-8.71876429852));
#32690=CARTESIAN_POINT('Ctrl Pts',(3.274071132333,6.721726401897,-8.798989801913));
#32691=CARTESIAN_POINT('Ctrl Pts',(3.428408819964,6.707046179747,-8.850734065253));
#32692=CARTESIAN_POINT('Ctrl Pts',(3.546552349393,6.700515345316,-8.863834484004));
#32693=CARTESIAN_POINT('Ctrl Pts',(3.61129082548,6.69839105866,-8.862870569862));
#32694=CARTESIAN_POINT('Ctrl Pts',(3.618965960468,6.698159820195,-8.862640873848));
#32695=CARTESIAN_POINT('Ctrl Pts',(3.182848670484,6.791546387898,-8.306825990365));
#32696=CARTESIAN_POINT('Ctrl Pts',(3.185008101237,6.790786308233,-8.310874692875));
#32697=CARTESIAN_POINT('Ctrl Pts',(3.203663420435,6.78441697955,-8.3446583261));
#32698=CARTESIAN_POINT('Ctrl Pts',(3.245894163072,6.772981061909,-8.403095186004));
#32699=CARTESIAN_POINT('Ctrl Pts',(3.319442410588,6.759004529431,-8.469324554359));
#32700=CARTESIAN_POINT('Ctrl Pts',(3.403175058521,6.747593048858,-8.518165951076));
#32701=CARTESIAN_POINT('Ctrl Pts',(3.496378554812,6.738838135146,-8.549542875217));
#32702=CARTESIAN_POINT('Ctrl Pts',(3.567485025904,6.734939152711,-8.557454533639));
#32703=CARTESIAN_POINT('Ctrl Pts',(3.606407852607,6.73366042859,-8.556875284136));
#32704=CARTESIAN_POINT('Ctrl Pts',(3.611021868203,6.733520983139,-8.556737012325));
#32705=CARTESIAN_POINT('',(3.579571669165,6.237540962482,-9.));
#32706=CARTESIAN_POINT('Ctrl Pts',(2.71354627856836,6.29590662785209,-8.50000002316856));
#32707=CARTESIAN_POINT('Ctrl Pts',(2.73271290696036,6.29276428740895,-8.53319622314795));
#32708=CARTESIAN_POINT('Ctrl Pts',(2.75362612200078,6.28969051942418,-8.56499171230839));
#32709=CARTESIAN_POINT('Ctrl Pts',(2.77608265061947,6.28670679356586,-8.59530196526257));
#32710=CARTESIAN_POINT('Ctrl Pts',(2.79626205372542,6.28402562196204,-8.62253871333666));
#32711=CARTESIAN_POINT('Ctrl Pts',(2.81768872536269,6.28141700629083,-8.6485766786427));
#32712=CARTESIAN_POINT('Ctrl Pts',(2.84025088394378,6.27889495274492,-8.67335338184266));
#32713=CARTESIAN_POINT('Ctrl Pts',(2.86150654311113,6.27651894291496,-8.6966953487301));
#32714=CARTESIAN_POINT('Ctrl Pts',(2.88377798700089,6.27421759335609,-8.718917609257));
#32715=CARTESIAN_POINT('Ctrl Pts',(2.90682907414929,6.2720086472179,-8.73987654658258));
#32716=CARTESIAN_POINT('Ctrl Pts',(2.92978054743643,6.26980924690515,-8.76074491114422));
#32717=CARTESIAN_POINT('Ctrl Pts',(2.95350429207167,6.26770154421663,-8.78036053410902));
#32718=CARTESIAN_POINT('Ctrl Pts',(2.97774532818122,6.26569567525515,-8.79862777462662));
#32719=CARTESIAN_POINT('Ctrl Pts',(2.98375967268792,6.26519800729594,-8.80315998509664));
#32720=CARTESIAN_POINT('Ctrl Pts',(2.98980578037816,6.26470656868169,-8.80760942851375));
#32721=CARTESIAN_POINT('Ctrl Pts',(2.99587961765459,6.26422143436467,-8.81197511614055));
#32722=CARTESIAN_POINT('Ctrl Pts',(3.01681927685196,6.26254892540517,-8.82702589983905));
#32723=CARTESIAN_POINT('Ctrl Pts',(3.03808451837945,6.2609566002826,-8.84108390682663));
#32724=CARTESIAN_POINT('Ctrl Pts',(3.05971475546151,6.25943353078172,-8.85424559056032));
#32725=CARTESIAN_POINT('Ctrl Pts',(3.08155208208703,6.257895879297,-8.86753328526029));
#32726=CARTESIAN_POINT('Ctrl Pts',(3.10376200877344,6.25642872123841,-8.87990776329837));
#32727=CARTESIAN_POINT('Ctrl Pts',(3.12641871308661,6.25502659177109,-8.89142795734024));
#32728=CARTESIAN_POINT('Ctrl Pts',(3.14041770081031,6.25416025247793,-8.89854598530838));
#32729=CARTESIAN_POINT('Ctrl Pts',(3.15458787574177,6.25331885754533,-8.9053370665679));
#32730=CARTESIAN_POINT('Ctrl Pts',(3.16895165114764,6.25250245441483,-8.91180655896024));
#32731=CARTESIAN_POINT('Ctrl Pts',(3.19352199871603,6.2511059337853,-8.92287312552643));
#32732=CARTESIAN_POINT('Ctrl Pts',(3.21864368964397,6.24978257411292,-8.93299444910136));
#32733=CARTESIAN_POINT('Ctrl Pts',(3.24439464561042,6.24852951272045,-8.94215563455501));
#32734=CARTESIAN_POINT('Ctrl Pts',(3.26942731660678,6.24731140362901,-8.95106128224036));
#32735=CARTESIAN_POINT('Ctrl Pts',(3.2950552167543,6.2461596666439,-8.95905977553184));
#32736=CARTESIAN_POINT('Ctrl Pts',(3.32135908871198,6.24507988147401,-8.96609031402971));
#32737=CARTESIAN_POINT('Ctrl Pts',(3.33477496679961,6.24452915395285,-8.96967613012286));
#32738=CARTESIAN_POINT('Ctrl Pts',(3.34836678575868,6.24399728208548,-8.97300936790168));
#32739=CARTESIAN_POINT('Ctrl Pts',(3.36214547754614,6.24348595006784,-8.97607676506084));
#32740=CARTESIAN_POINT('Ctrl Pts',(3.39643763297189,6.24221335631991,-8.9837108468559));
#32741=CARTESIAN_POINT('Ctrl Pts',(3.43188068992917,6.24106093218739,-8.98969329898011));
#32742=CARTESIAN_POINT('Ctrl Pts',(3.46821448374441,6.24005961143774,-8.99376551635245));
#32743=CARTESIAN_POINT('Ctrl Pts',(3.50454827755965,6.23905829068809,-8.99783773372479));
#32744=CARTESIAN_POINT('Ctrl Pts',(3.54177264129656,6.23820808731495,-8.99999965435044));
#32745=CARTESIAN_POINT('Ctrl Pts',(3.579571669165,6.237540962482,-9.00000000000001));
#32746=CARTESIAN_POINT('Origin',(3.579571668976,6.237540962483,-8.5));
#32747=CARTESIAN_POINT('Origin',(3.579571668976,17.50736,-8.));
#32748=CARTESIAN_POINT('',(3.57957168029041,1.36245903804411,-9.00000000000025));
#32749=CARTESIAN_POINT('',(3.579571669165,6.237540962482,-9.));
#32750=CARTESIAN_POINT('Ctrl Pts',(3.57957166916,1.362459037518,-9.));
#32751=CARTESIAN_POINT('Ctrl Pts',(3.53067956146749,1.36159569723168,-9.000000000009));
#32752=CARTESIAN_POINT('Ctrl Pts',(3.48229116327313,1.36042549044103,-8.99641626892138));
#32753=CARTESIAN_POINT('Ctrl Pts',(3.43474696375249,1.35897335420425,-8.9894573284164));
#32754=CARTESIAN_POINT('Ctrl Pts',(3.41174502962636,1.35827080915359,-8.98609058562344));
#32755=CARTESIAN_POINT('Ctrl Pts',(3.38893988987502,1.35750227471969,-8.98193347499698));
#32756=CARTESIAN_POINT('Ctrl Pts',(3.36636648175544,1.35667057477884,-8.97700744528496));
#32757=CARTESIAN_POINT('Ctrl Pts',(3.3375005477531,1.35560703153914,-8.97070824368423));
#32758=CARTESIAN_POINT('Ctrl Pts',(3.309008416789,1.35444019861569,-8.96314601327225));
#32759=CARTESIAN_POINT('Ctrl Pts',(3.28110543490607,1.35318521002559,-8.95442019421223));
#32760=CARTESIAN_POINT('Ctrl Pts',(3.25302206326135,1.35192210806991,-8.94563796367519));
#32761=CARTESIAN_POINT('Ctrl Pts',(3.22553607665365,1.35056970692941,-8.93567739095572));
#32762=CARTESIAN_POINT('Ctrl Pts',(3.19884192411574,1.34914343604218,-8.92468635838248));
#32763=CARTESIAN_POINT('Ctrl Pts',(3.18844693309194,1.34858803076946,-8.92040633170701));
#32764=CARTESIAN_POINT('Ctrl Pts',(3.17817170134369,1.34802142383197,-8.91597051268099));
#32765=CARTESIAN_POINT('Ctrl Pts',(3.16802641451614,1.3474445263465,-8.91138932599168));
#32766=CARTESIAN_POINT('Ctrl Pts',(3.14307589340737,1.34602575000893,-8.90012271548201));
#32767=CARTESIAN_POINT('Ctrl Pts',(3.11891002670089,1.34454473374312,-8.88798168376388));
#32768=CARTESIAN_POINT('Ctrl Pts',(3.09542161957199,1.3430008971863,-8.87498498824957));
#32769=CARTESIAN_POINT('Ctrl Pts',(3.07167229857546,1.34143991138795,-8.86184392287337));
#32770=CARTESIAN_POINT('Ctrl Pts',(3.04861489058827,1.33981470190665,-8.84782773667852));
#32771=CARTESIAN_POINT('Ctrl Pts',(3.02615772706361,1.3381246688236,-8.83290636262246));
#32772=CARTESIAN_POINT('Ctrl Pts',(3.0155596267221,1.33732709970161,-8.82586459088199));
#32773=CARTESIAN_POINT('Ctrl Pts',(3.0050955469187,1.3365150934981,-8.81862054492759));
#32774=CARTESIAN_POINT('Ctrl Pts',(2.99475796750508,1.33568858715917,-8.81116763654123));
#32775=CARTESIAN_POINT('Ctrl Pts',(2.97315509353913,1.33396140214249,-8.79559298080138));
#32776=CARTESIAN_POINT('Ctrl Pts',(2.9521153696349,1.33217089472038,-8.77911803949023));
#32777=CARTESIAN_POINT('Ctrl Pts',(2.93158843147111,1.33030591798024,-8.76165459620007));
#32778=CARTESIAN_POINT('Ctrl Pts',(2.9114806336299,1.32847902227031,-8.74454773961541));
#32779=CARTESIAN_POINT('Ctrl Pts',(2.89186441996441,1.32658066737695,-8.72649182314979));
#32780=CARTESIAN_POINT('Ctrl Pts',(2.87273094267328,1.32460037536748,-8.70737273600263));
#32781=CARTESIAN_POINT('Ctrl Pts',(2.86265638108103,1.32355767029529,-8.69730575141217));
#32782=CARTESIAN_POINT('Ctrl Pts',(2.85271634578784,1.32249224852657,-8.68694352705419));
#32783=CARTESIAN_POINT('Ctrl Pts',(2.84291467409078,1.32140258048075,-8.67626656865963));
#32784=CARTESIAN_POINT('Ctrl Pts',(2.82156544990445,1.3190291519353,-8.65301086438402));
#32785=CARTESIAN_POINT('Ctrl Pts',(2.80087871271009,1.316540693963,-8.62826131105066));
#32786=CARTESIAN_POINT('Ctrl Pts',(2.7811381471473,1.31395624459894,-8.60208297702246));
#32787=CARTESIAN_POINT('Ctrl Pts',(2.76162204893333,1.3114011826653,-8.57620231335314));
#32788=CARTESIAN_POINT('Ctrl Pts',(2.7430313720079,1.30875229993928,-8.5489252917344));
#32789=CARTESIAN_POINT('Ctrl Pts',(2.72562719938734,1.30602799237575,-8.5203641444786));
#32790=CARTESIAN_POINT('Ctrl Pts',(2.72153358428764,1.30538721117796,-8.51364631041545));
#32791=CARTESIAN_POINT('Ctrl Pts',(2.71750552908601,1.30474225723723,-8.50685764623042));
#32792=CARTESIAN_POINT('Ctrl Pts',(2.71354626504425,1.304093369931,-8.49999999974485));
#32793=CARTESIAN_POINT('Ctrl Pts',(3.606118439109,1.452111117783,-8.991622013561));
#32794=CARTESIAN_POINT('Ctrl Pts',(3.596226549993,1.451813160933,-8.991916534875));
#32795=CARTESIAN_POINT('Ctrl Pts',(3.514295435264,1.449125030121,-8.993132242195));
#32796=CARTESIAN_POINT('Ctrl Pts',(3.361902292376,1.440755734761,-8.976686868883));
#32797=CARTESIAN_POINT('Ctrl Pts',(3.162806797501,1.421866077181,-8.91075977445));
#32798=CARTESIAN_POINT('Ctrl Pts',(2.985508542217,1.397316177247,-8.80817459468));
#32799=CARTESIAN_POINT('Ctrl Pts',(2.83073332976,1.367610099334,-8.670666976124));
#32800=CARTESIAN_POINT('Ctrl Pts',(2.742180934874,1.343511145381,-8.549950688678));
#32801=CARTESIAN_POINT('Ctrl Pts',(2.702500790941,1.329891627237,-8.478869336066));
#32802=CARTESIAN_POINT('Ctrl Pts',(2.697982963143,1.328293519144,-8.470490213466));
#32803=CARTESIAN_POINT('Ctrl Pts',(3.616909261623,1.149147376315,-9.046288487242));
#32804=CARTESIAN_POINT('Ctrl Pts',(3.607000480323,1.148849039803,-9.046584238161));
#32805=CARTESIAN_POINT('Ctrl Pts',(3.524929471719,1.146156716061,-9.047804254029));
#32806=CARTESIAN_POINT('Ctrl Pts',(3.372276437766,1.137763587628,-9.031277044035));
#32807=CARTESIAN_POINT('Ctrl Pts',(3.172842746773,1.118804854858,-8.965029105095));
#32808=CARTESIAN_POINT('Ctrl Pts',(2.995244772122,1.094156444364,-8.861946457188));
#32809=CARTESIAN_POINT('Ctrl Pts',(2.840209180296,1.064324590375,-8.723772668877));
#32810=CARTESIAN_POINT('Ctrl Pts',(2.75150843471,1.040119415609,-8.602471763629));
#32811=CARTESIAN_POINT('Ctrl Pts',(2.711761902532,1.026438673235,-8.531046265659));
#32812=CARTESIAN_POINT('Ctrl Pts',(2.707236517197,1.024833365209,-8.522626576234));
#32813=CARTESIAN_POINT('Ctrl Pts',(3.618984699362,0.9018408279155,-8.862640775326));
#32814=CARTESIAN_POINT('Ctrl Pts',(3.611303055056,0.9016093738728,-8.86287056766));
#32815=CARTESIAN_POINT('Ctrl Pts',(3.547676246624,0.8995214772279,-8.863817500059));
#32816=CARTESIAN_POINT('Ctrl Pts',(3.429288349975,0.8930245062433,-8.850954493995));
#32817=CARTESIAN_POINT('Ctrl Pts',(3.274443865634,0.8783462364203,-8.799327648757));
#32818=CARTESIAN_POINT('Ctrl Pts',(3.136362160075,0.8592365357768,-8.718883846345));
#32819=CARTESIAN_POINT('Ctrl Pts',(3.015656085662,0.8360650174749,-8.610909097964));
#32820=CARTESIAN_POINT('Ctrl Pts',(2.946514523875,0.8172237841081,-8.516008288557));
#32821=CARTESIAN_POINT('Ctrl Pts',(2.915520898728,0.8065617493812,-8.460105247678));
#32822=CARTESIAN_POINT('Ctrl Pts',(2.911991930924,0.8053104895109,-8.453515076827));
#32823=CARTESIAN_POINT('Ctrl Pts',(3.611033157925,0.8664794103834,-8.55673695376));
#32824=CARTESIAN_POINT('Ctrl Pts',(3.606415217474,0.8663398338715,-8.556875282532));
#32825=CARTESIAN_POINT('Ctrl Pts',(3.568160699697,0.8650830103777,-8.557444317374));
#32826=CARTESIAN_POINT('Ctrl Pts',(3.496908759876,0.8612038910007,-8.549675924183));
#32827=CARTESIAN_POINT('Ctrl Pts',(3.403402273431,0.852450539314,-8.518372159072));
#32828=CARTESIAN_POINT('Ctrl Pts',(3.319680109389,0.8410165238057,-8.469396662616));
#32829=CARTESIAN_POINT('Ctrl Pts',(3.24619855465,0.8270823847512,-8.403401567405));
#32830=CARTESIAN_POINT('Ctrl Pts',(3.203963082135,0.8156854566047,-8.345201753149));
#32831=CARTESIAN_POINT('Ctrl Pts',(3.18501016893,0.8092143577992,-8.310878194086));
#32832=CARTESIAN_POINT('Ctrl Pts',(3.182851897331,0.8084546497716,-8.306831443972));
#32833=CARTESIAN_POINT('Origin',(3.579571686039,1.362459038122,-8.500000000001));
#32834=CARTESIAN_POINT('Origin',(3.146558966941,1.304093369921,-8.249999999753));
#32835=CARTESIAN_POINT('Ctrl Pts',(2.737554087051,1.34152810419,-8.539856081031));
#32836=CARTESIAN_POINT('Ctrl Pts',(2.729007055677,1.338703332081,-8.525052188437));
#32837=CARTESIAN_POINT('Ctrl Pts',(2.499808905038,1.26314158189,-8.128069346529));
#32838=CARTESIAN_POINT('Ctrl Pts',(2.046877238873,1.123743738896,-7.343568688376));
#32839=CARTESIAN_POINT('Ctrl Pts',(1.352547748218,0.9392672044454,-6.140954733368));
#32840=CARTESIAN_POINT('Ctrl Pts',(0.7051558095594,0.7959101378268,-5.0196390032));
#32841=CARTESIAN_POINT('Ctrl Pts',(0.2815322151021,0.7187111648313,-4.285901414315));
#32842=CARTESIAN_POINT('Ctrl Pts',(0.1075907271497,0.6897998149103,-3.984625919637));
#32843=CARTESIAN_POINT('Ctrl Pts',(2.747286251397,1.027333500649,-8.594189576059));
#32844=CARTESIAN_POINT('Ctrl Pts',(2.738697483667,1.024494934782,-8.579313393976));
#32845=CARTESIAN_POINT('Ctrl Pts',(2.508380197487,0.9485642294144,-8.18039215245));
#32846=CARTESIAN_POINT('Ctrl Pts',(2.053240695369,0.8084869567693,-7.392067410251));
#32847=CARTESIAN_POINT('Ctrl Pts',(1.355536410545,0.6231138684716,-6.183608140278));
#32848=CARTESIAN_POINT('Ctrl Pts',(0.7050060546966,0.4790619292973,-5.056856512082));
#32849=CARTESIAN_POINT('Ctrl Pts',(0.2793327299031,0.4014894447593,-4.319568686113));
#32850=CARTESIAN_POINT('Ctrl Pts',(0.1045501668528,0.3724382976097,-4.016836406632));
#32851=CARTESIAN_POINT('Ctrl Pts',(2.960318350366,0.8038948754913,-8.513830393669));
#32852=CARTESIAN_POINT('Ctrl Pts',(2.951699901941,0.8010465002312,-8.498902803114));
#32853=CARTESIAN_POINT('Ctrl Pts',(2.720586745609,0.7248534134077,-8.09860307405));
#32854=CARTESIAN_POINT('Ctrl Pts',(2.263877147047,0.5842929662415,-7.307558845036));
#32855=CARTESIAN_POINT('Ctrl Pts',(1.563772886664,0.3982822961497,-6.094942695458));
#32856=CARTESIAN_POINT('Ctrl Pts',(0.9110106540926,0.2537362002753,-4.964325343381));
#32857=CARTESIAN_POINT('Ctrl Pts',(0.4838796692276,0.1758980940347,-4.224512776108));
#32858=CARTESIAN_POINT('Ctrl Pts',(0.3084989779427,0.1467475304718,-3.920744508136));
#32859=CARTESIAN_POINT('Ctrl Pts',(3.23490900795,0.819877609831,-8.352245692761));
#32860=CARTESIAN_POINT('Ctrl Pts',(3.226292682607,0.8170299362443,-8.337321779493));
#32861=CARTESIAN_POINT('Ctrl Pts',(2.995236455471,0.7408556177653,-7.937120654688));
#32862=CARTESIAN_POINT('Ctrl Pts',(2.538639167099,0.6003297324392,-7.146270952629));
#32863=CARTESIAN_POINT('Ctrl Pts',(1.838706578788,0.4143646690566,-5.933952147802));
#32864=CARTESIAN_POINT('Ctrl Pts',(1.186103994052,0.2698539205859,-4.803611313887));
#32865=CARTESIAN_POINT('Ctrl Pts',(0.759077276717,0.1920348144671,-4.063979343274));
#32866=CARTESIAN_POINT('Ctrl Pts',(0.5837393699985,0.1628913622357,-3.760285180345));
#32867=CARTESIAN_POINT('Ctrl Pts',(9.065473909596,1.586334475001,-8.999136656895));
#32868=CARTESIAN_POINT('Ctrl Pts',(9.02961154137,1.58506300137,-8.999136656895));
#32869=CARTESIAN_POINT('Ctrl Pts',(8.395666997776,1.562586994821,-8.999136656895));
#32870=CARTESIAN_POINT('Ctrl Pts',(7.164016283661,1.518920692298,-8.999136656895));
#32871=CARTESIAN_POINT('Ctrl Pts',(5.370897733403,1.455350884028,-8.999136656895));
#32872=CARTESIAN_POINT('Ctrl Pts',(4.139998972163,1.411714641081,-8.999136656895));
#32873=CARTESIAN_POINT('Ctrl Pts',(3.506806407366,1.389267971541,-8.999136656895));
#32874=CARTESIAN_POINT('Ctrl Pts',(3.470944033629,1.387996652259,-8.999136656895));
#32875=CARTESIAN_POINT('Ctrl Pts',(9.07538462932,1.306799082875,-9.015595309496));
#32876=CARTESIAN_POINT('Ctrl Pts',(9.039522253334,1.305527608968,-9.015595309496));
#32877=CARTESIAN_POINT('Ctrl Pts',(8.405577572588,1.283051597556,-9.015595309496));
#32878=CARTESIAN_POINT('Ctrl Pts',(7.173926592565,1.239385285606,-9.015595309496));
#32879=CARTESIAN_POINT('Ctrl Pts',(5.380807656699,1.175815463665,-9.015595309496));
#32880=CARTESIAN_POINT('Ctrl Pts',(4.149908631793,1.132179211371,-9.015595309496));
#32881=CARTESIAN_POINT('Ctrl Pts',(3.516715931643,1.109732537033,-9.015595309496));
#32882=CARTESIAN_POINT('Ctrl Pts',(3.480853550242,1.108461217479,-9.015595309496));
#32883=CARTESIAN_POINT('Ctrl Pts',(9.082984626861,1.092438435823,-8.835315254872));
#32884=CARTESIAN_POINT('Ctrl Pts',(9.047122244925,1.091166961705,-8.835315254872));
#32885=CARTESIAN_POINT('Ctrl Pts',(8.413177459004,1.068690946564,-8.835315254872));
#32886=CARTESIAN_POINT('Ctrl Pts',(7.18152627507,1.025024627385,-8.835315254871));
#32887=CARTESIAN_POINT('Ctrl Pts',(5.388407043503,0.9614547949613,-8.835315254871));
#32888=CARTESIAN_POINT('Ctrl Pts',(4.157507816405,0.9178185354994,-8.835315254872));
#32889=CARTESIAN_POINT('Ctrl Pts',(3.524315012461,0.8953718574817,-8.835315254872));
#32890=CARTESIAN_POINT('Ctrl Pts',(3.488452625181,0.8941005377194,-8.835315254872));
#32891=CARTESIAN_POINT('Ctrl Pts',(9.084115280216,1.060547953822,-8.556943446236));
#32892=CARTESIAN_POINT('Ctrl Pts',(9.048252897395,1.059276479673,-8.556943446236));
#32893=CARTESIAN_POINT('Ctrl Pts',(8.414308095827,1.036800463978,-8.556943446236));
#32894=CARTESIAN_POINT('Ctrl Pts',(7.182656881557,0.9931341437232,-8.556943446236));
#32895=CARTESIAN_POINT('Ctrl Pts',(5.389537605998,0.9295643097394,-8.556943446236));
#32896=CARTESIAN_POINT('Ctrl Pts',(4.158638348821,0.8859280492112,-8.556943446236));
#32897=CARTESIAN_POINT('Ctrl Pts',(3.525445529435,0.8634813706461,-8.556943446236));
#32898=CARTESIAN_POINT('Ctrl Pts',(3.489583141281,0.8622100508528,-8.556943446236));
#32899=CARTESIAN_POINT('',(8.95892744039,1.553168485875,-9.));
#32900=CARTESIAN_POINT('',(8.95892744039,1.553168485875,-9.));
#32901=CARTESIAN_POINT('Origin',(8.958927440522,1.553168485878,-8.5));
#32902=CARTESIAN_POINT('Origin',(9.335521399786,0.,-9.));
#32903=CARTESIAN_POINT('',(8.9589274516891,6.04683151365134,-8.99999999999974));
#32904=CARTESIAN_POINT('',(3.579571669165,6.237540962482,-9.));
#32905=CARTESIAN_POINT('',(8.958927440394,6.046831514125,-9.));
#32906=CARTESIAN_POINT('Ctrl Pts',(3.470944033141,6.212003347758,-8.999136656895));
#32907=CARTESIAN_POINT('Ctrl Pts',(3.50680640704,6.21073202847,-8.999136656895));
#32908=CARTESIAN_POINT('Ctrl Pts',(4.139999211807,6.188285350424,-8.999136656895));
#32909=CARTESIAN_POINT('Ctrl Pts',(5.370898213018,6.144649098969,-8.999136656895));
#32910=CARTESIAN_POINT('Ctrl Pts',(7.164016763276,6.081079290698,-8.999136656895));
#32911=CARTESIAN_POINT('Ctrl Pts',(8.395667245888,6.037412996383,-8.999136656895));
#32912=CARTESIAN_POINT('Ctrl Pts',(9.029611557979,6.014936998041,-8.999136656895));
#32913=CARTESIAN_POINT('Ctrl Pts',(9.06547393451,6.013665524115,-8.999136656895));
#32914=CARTESIAN_POINT('Ctrl Pts',(3.480853549753,6.491538782538,-9.015595309496));
#32915=CARTESIAN_POINT('Ctrl Pts',(3.516715931318,6.490267462978,-9.015595309496));
#32916=CARTESIAN_POINT('Ctrl Pts',(4.149908871438,6.467820780133,-9.015595309496));
#32917=CARTESIAN_POINT('Ctrl Pts',(5.380808136314,6.424184519332,-9.015595309496));
#32918=CARTESIAN_POINT('Ctrl Pts',(7.17392707218,6.36061469739,-9.015595309496));
#32919=CARTESIAN_POINT('Ctrl Pts',(8.4055778207,6.316948393647,-9.015595309496));
#32920=CARTESIAN_POINT('Ctrl Pts',(9.039522269944,6.294472390443,-9.015595309496));
#32921=CARTESIAN_POINT('Ctrl Pts',(9.075384654235,6.293200916242,-9.015595309496));
#32922=CARTESIAN_POINT('Ctrl Pts',(3.488452624693,6.705899462298,-8.835315254871));
#32923=CARTESIAN_POINT('Ctrl Pts',(3.524315012135,6.70462814253,-8.835315254871));
#32924=CARTESIAN_POINT('Ctrl Pts',(4.15750805605,6.682181456005,-8.835315254872));
#32925=CARTESIAN_POINT('Ctrl Pts',(5.388407523118,6.638545188036,-8.835315254871));
#32926=CARTESIAN_POINT('Ctrl Pts',(7.181526754685,6.574975355611,-8.835315254871));
#32927=CARTESIAN_POINT('Ctrl Pts',(8.413177707116,6.531309044639,-8.835315254872));
#32928=CARTESIAN_POINT('Ctrl Pts',(9.047122261535,6.508833037706,-8.835315254871));
#32929=CARTESIAN_POINT('Ctrl Pts',(9.082984651776,6.507561563294,-8.835315254871));
#32930=CARTESIAN_POINT('Ctrl Pts',(3.489583140792,6.737789949165,-8.556943446236));
#32931=CARTESIAN_POINT('Ctrl Pts',(3.525445529109,6.736518629365,-8.556943446236));
#32932=CARTESIAN_POINT('Ctrl Pts',(4.158638588465,6.714071942293,-8.556943446236));
#32933=CARTESIAN_POINT('Ctrl Pts',(5.389538085613,6.670435673258,-8.556943446236));
#32934=CARTESIAN_POINT('Ctrl Pts',(7.182657361173,6.606865839273,-8.556943446236));
#32935=CARTESIAN_POINT('Ctrl Pts',(8.414308343939,6.563199527226,-8.556943446236));
#32936=CARTESIAN_POINT('Ctrl Pts',(9.048252914005,6.540723519738,-8.556943446236));
#32937=CARTESIAN_POINT('Ctrl Pts',(9.084115305131,6.539452045294,-8.556943446236));
#32938=CARTESIAN_POINT('Origin',(8.958927452512,6.046831513697,-8.499999999999));
#32939=CARTESIAN_POINT('Ctrl Pts',(8.927938928541,6.006828531619,-8.997867591216));
#32940=CARTESIAN_POINT('Ctrl Pts',(8.937774429904,6.00642695855,-8.998158451035));
#32941=CARTESIAN_POINT('Ctrl Pts',(9.006435353586,6.003807560836,-8.99917072319));
#32942=CARTESIAN_POINT('Ctrl Pts',(9.134996901011,6.001289846702,-8.987861041925));
#32943=CARTESIAN_POINT('Ctrl Pts',(9.310154709202,6.003639088283,-8.940357378065));
#32944=CARTESIAN_POINT('Ctrl Pts',(9.480463368067,6.012209681015,-8.858861787215));
#32945=CARTESIAN_POINT('Ctrl Pts',(9.591730727664,6.022942085977,-8.776282372617));
#32946=CARTESIAN_POINT('Ctrl Pts',(9.646942429761,6.030093692078,-8.724650169732));
#32947=CARTESIAN_POINT('Ctrl Pts',(9.653937673143,6.031033325521,-8.717912229442));
#32948=CARTESIAN_POINT('Ctrl Pts',(8.938791953801,6.291076248276,-9.02137079219));
#32949=CARTESIAN_POINT('Ctrl Pts',(8.948369630768,6.290685072941,-9.021655027771));
#32950=CARTESIAN_POINT('Ctrl Pts',(9.015230406025,6.28813382963,-9.022644820733));
#32951=CARTESIAN_POINT('Ctrl Pts',(9.140418016028,6.285686148486,-9.011601251901));
#32952=CARTESIAN_POINT('Ctrl Pts',(9.310978373003,6.287991261734,-8.965209492321));
#32953=CARTESIAN_POINT('Ctrl Pts',(9.476823523468,6.29636809076,-8.885616148791));
#32954=CARTESIAN_POINT('Ctrl Pts',(9.585183697085,6.306852394716,-8.804956031936));
#32955=CARTESIAN_POINT('Ctrl Pts',(9.638956172709,6.313838355042,-8.75451988478));
#32956=CARTESIAN_POINT('Ctrl Pts',(9.645769129904,6.31475622189,-8.747937965196));
#32957=CARTESIAN_POINT('Ctrl Pts',(8.953058757155,6.511404577949,-8.840488172299));
#32958=CARTESIAN_POINT('Ctrl Pts',(8.960489665714,6.511101332867,-8.840709539929));
#32959=CARTESIAN_POINT('Ctrl Pts',(9.01236154992,6.509123086244,-8.841480762696));
#32960=CARTESIAN_POINT('Ctrl Pts',(9.109456153971,6.507217777614,-8.83288514462));
#32961=CARTESIAN_POINT('Ctrl Pts',(9.241735947841,6.508976141369,-8.796775018666));
#32962=CARTESIAN_POINT('Ctrl Pts',(9.370415806732,6.515429682801,-8.734796114743));
#32963=CARTESIAN_POINT('Ctrl Pts',(9.454569368652,6.523533628542,-8.671929757642));
#32964=CARTESIAN_POINT('Ctrl Pts',(9.496358160883,6.528943855231,-8.632590750232));
#32965=CARTESIAN_POINT('Ctrl Pts',(9.501653316682,6.529654845007,-8.627456542266));
#32966=CARTESIAN_POINT('Ctrl Pts',(8.962706207688,6.543754453392,-8.557068318775));
#32967=CARTESIAN_POINT('Ctrl Pts',(8.967310172969,6.543567160675,-8.557205973457));
#32968=CARTESIAN_POINT('Ctrl Pts',(8.999444136385,6.542344118915,-8.55768560415));
#32969=CARTESIAN_POINT('Ctrl Pts',(9.059544841125,6.541148131598,-8.552341420912));
#32970=CARTESIAN_POINT('Ctrl Pts',(9.141415387249,6.542164979948,-8.529893434732));
#32971=CARTESIAN_POINT('Ctrl Pts',(9.2211546288,6.546048644919,-8.491323096556));
#32972=CARTESIAN_POINT('Ctrl Pts',(9.273432037729,6.550980270515,-8.45210592626));
#32973=CARTESIAN_POINT('Ctrl Pts',(9.299440276694,6.554291915423,-8.427516736843));
#32974=CARTESIAN_POINT('Ctrl Pts',(9.302736736018,6.554727402792,-8.424306776346));
#32975=CARTESIAN_POINT('',(9.631273226501,6.057526622699,-8.740237221487));
#32976=CARTESIAN_POINT('Ctrl Pts',(8.95892745169395,6.04683151392516,-8.99999999999995));
#32977=CARTESIAN_POINT('Ctrl Pts',(9.00313304379479,6.04604972402664,-8.99999898867999));
#32978=CARTESIAN_POINT('Ctrl Pts',(9.04760587323135,6.0455202798527,-8.99704958523495));
#32979=CARTESIAN_POINT('Ctrl Pts',(9.0917825090689,6.04525525204683,-8.99113201402888));
#32980=CARTESIAN_POINT('Ctrl Pts',(9.10585477641443,6.04517082863913,-8.98924699851176));
#32981=CARTESIAN_POINT('Ctrl Pts',(9.1198968933399,6.04511317331886,-8.98706118387352));
#32982=CARTESIAN_POINT('Ctrl Pts',(9.13389048489755,6.04508249896408,-8.98457500125824));
#32983=CARTESIAN_POINT('Ctrl Pts',(9.1628521082268,6.04501901425359,-8.97942951132918));
#32984=CARTESIAN_POINT('Ctrl Pts',(9.19160465322972,6.04507401878512,-8.97300230786102));
#32985=CARTESIAN_POINT('Ctrl Pts',(9.22017512254227,6.04524499188232,-8.96526941126628));
#32986=CARTESIAN_POINT('Ctrl Pts',(9.24874559185483,6.04541596497953,-8.95753651467154));
#32987=CARTESIAN_POINT('Ctrl Pts',(9.27713482025089,6.04570290954913,-8.94849779093512));
#32988=CARTESIAN_POINT('Ctrl Pts',(9.30534741011489,6.04611300830617,-8.93807953003303));
#32989=CARTESIAN_POINT('Ctrl Pts',(9.33355999997888,6.04652310706321,-8.92766126913094));
#32990=CARTESIAN_POINT('Ctrl Pts',(9.36158834110619,6.0470562702359,-8.91586640524687));
#32991=CARTESIAN_POINT('Ctrl Pts',(9.38941945465935,6.04772000825609,-8.9025928143899));
#32992=CARTESIAN_POINT('Ctrl Pts',(9.41506316740826,6.04833157944233,-8.89036246829066));
#32993=CARTESIAN_POINT('Ctrl Pts',(9.44053971294124,6.04905411615378,-8.87687607922135));
#32994=CARTESIAN_POINT('Ctrl Pts',(9.46580248313527,6.04990050739418,-8.86202001340548));
#32995=CARTESIAN_POINT('Ctrl Pts',(9.46795738965685,6.04997270430647,-8.86075279556414));
#32996=CARTESIAN_POINT('Ctrl Pts',(9.47011071559531,6.05004580639459,-8.85947559313687));
#32997=CARTESIAN_POINT('Ctrl Pts',(9.4722624174361,6.050119823895,-8.85818832518149));
#32998=CARTESIAN_POINT('Ctrl Pts',(9.50110713898193,6.05111206833537,-8.84093180523811));
#32999=CARTESIAN_POINT('Ctrl Pts',(9.52965700600334,6.05226429513786,-8.82186747223183));
#33000=CARTESIAN_POINT('Ctrl Pts',(9.55761457757172,6.05358096894265,-8.8009715755454));
#33001=CARTESIAN_POINT('Ctrl Pts',(9.58272679945829,6.05476363978576,-8.78220233470397));
#33002=CARTESIAN_POINT('Ctrl Pts',(9.60736070239246,6.05607893807379,-8.76195568320717));
#33003=CARTESIAN_POINT('Ctrl Pts',(9.63127322650134,6.057526622699,-8.74023722148736));
#33004=CARTESIAN_POINT('Origin',(9.295100333699,6.057526622722,-8.370118610573));
#33005=CARTESIAN_POINT('Origin',(8.958927440522,17.50736,-8.));
#33006=CARTESIAN_POINT('',(9.63127321029653,1.54247337967211,-8.74023723620533));
#33007=CARTESIAN_POINT('',(9.631273226501,6.057526622699,-8.740237221487));
#33008=CARTESIAN_POINT('Ctrl Pts',(9.63127321025096,1.54247337828569,-8.74023723624765));
#33009=CARTESIAN_POINT('Ctrl Pts',(9.6057200390174,1.54402189862992,-8.76344677737955));
#33010=CARTESIAN_POINT('Ctrl Pts',(9.5788416935493,1.54544836517941,-8.78543940428296));
#33011=CARTESIAN_POINT('Ctrl Pts',(9.55081894029273,1.54673721047252,-8.80601765024047));
#33012=CARTESIAN_POINT('Ctrl Pts',(9.53152029367347,1.54762480954714,-8.82018943033437));
#33013=CARTESIAN_POINT('Ctrl Pts',(9.51167976745598,1.54844713801948,-8.8336910486412));
#33014=CARTESIAN_POINT('Ctrl Pts',(9.49136629635905,1.54919911118225,-8.8464684665095));
#33015=CARTESIAN_POINT('Ctrl Pts',(9.46506696218071,1.55017267170307,-8.86301106431817));
#33016=CARTESIAN_POINT('Ctrl Pts',(9.43797899027672,1.55102830390587,-8.87834410170704));
#33017=CARTESIAN_POINT('Ctrl Pts',(9.41005849198976,1.55176304374565,-8.89245771574993));
#33018=CARTESIAN_POINT('Ctrl Pts',(9.38509876020795,1.55241986975004,-8.9050746833041));
#33019=CARTESIAN_POINT('Ctrl Pts',(9.35947295571484,1.55298008346687,-8.91671676781031));
#33020=CARTESIAN_POINT('Ctrl Pts',(9.33313997277414,1.5534415673395,-8.92734296821911));
#33021=CARTESIAN_POINT('Ctrl Pts',(9.30524515786841,1.55393042221925,-8.93859941775323));
#33022=CARTESIAN_POINT('Ctrl Pts',(9.27656418794365,1.55430848844038,-8.94871368108735));
#33023=CARTESIAN_POINT('Ctrl Pts',(9.2470373763062,1.55456292647825,-8.95759733964878));
#33024=CARTESIAN_POINT('Ctrl Pts',(9.21751056466876,1.55481736451613,-8.96648099821022));
#33025=CARTESIAN_POINT('Ctrl Pts',(9.18713704206229,1.55494817437075,-8.97413435291267));
#33026=CARTESIAN_POINT('Ctrl Pts',(9.15586562026909,1.5549425165175,-8.9804159083562));
#33027=CARTESIAN_POINT('Ctrl Pts',(9.12334173955173,1.55493663206027,-8.98694904782506));
#33028=CARTESIAN_POINT('Ctrl Pts',(9.08984768872008,1.5547831295879,-8.99199043374914));
#33029=CARTESIAN_POINT('Ctrl Pts',(9.05558312753583,1.55446759872465,-8.9953178779505));
#33030=CARTESIAN_POINT('Ctrl Pts',(9.02395754758573,1.55417636935538,-8.99838904970879));
#33031=CARTESIAN_POINT('Ctrl Pts',(8.99167619777338,1.55374710862609,-9.00000000000432));
#33032=CARTESIAN_POINT('Ctrl Pts',(8.95892744039,1.553168485875,-9.));
#33033=CARTESIAN_POINT('Ctrl Pts',(9.6539425342,1.568966285828,-8.717909048124));
#33034=CARTESIAN_POINT('Ctrl Pts',(9.646944923898,1.569906069969,-8.72464832123));
#33035=CARTESIAN_POINT('Ctrl Pts',(9.597148177396,1.576355760916,-8.771213723106));
#33036=CARTESIAN_POINT('Ctrl Pts',(9.494950476551,1.58651869939,-8.848842890954));
#33037=CARTESIAN_POINT('Ctrl Pts',(9.333640806294,1.595561978493,-8.931284233888));
#33038=CARTESIAN_POINT('Ctrl Pts',(9.152534187008,1.598909442216,-8.985523427163));
#33039=CARTESIAN_POINT('Ctrl Pts',(9.013894746136,1.59647733588,-8.999282347838));
#33040=CARTESIAN_POINT('Ctrl Pts',(8.937785978218,1.593573411533,-8.998158240137));
#33041=CARTESIAN_POINT('Ctrl Pts',(8.927957313071,1.593172004412,-8.997866979416));
#33042=CARTESIAN_POINT('Ctrl Pts',(9.645773859302,1.285243398955,-8.747934853163));
#33043=CARTESIAN_POINT('Ctrl Pts',(9.638958599346,1.286161413433,-8.754518076087));
#33044=CARTESIAN_POINT('Ctrl Pts',(9.590459936523,1.29246171878,-8.800004804342));
#33045=CARTESIAN_POINT('Ctrl Pts',(9.490931861646,1.302389666159,-8.875830399956));
#33046=CARTESIAN_POINT('Ctrl Pts',(9.333848365003,1.311227380035,-8.956348467272));
#33047=CARTESIAN_POINT('Ctrl Pts',(9.157494856417,1.314507075387,-9.0093185165));
#33048=CARTESIAN_POINT('Ctrl Pts',(9.022494227322,1.312143653767,-9.022753948681));
#33049=CARTESIAN_POINT('Ctrl Pts',(8.948380876688,1.309315289639,-9.021654826406));
#33050=CARTESIAN_POINT('Ctrl Pts',(8.938809856917,1.308924276241,-9.021370203034));
#33051=CARTESIAN_POINT('Ctrl Pts',(9.501656950695,1.070344855274,-8.627454082903));
#33052=CARTESIAN_POINT('Ctrl Pts',(9.496360026356,1.071055961909,-8.632589318456));
#33053=CARTESIAN_POINT('Ctrl Pts',(9.458669824932,1.075935204229,-8.668067974497));
#33054=CARTESIAN_POINT('Ctrl Pts',(9.381370324166,1.083610835663,-8.727171256311));
#33055=CARTESIAN_POINT('Ctrl Pts',(9.259475956808,1.090423267748,-8.789877060081));
#33056=CARTESIAN_POINT('Ctrl Pts',(9.122699106024,1.092933570735,-8.831108527563));
#33057=CARTESIAN_POINT('Ctrl Pts',(9.017996952515,1.091092054531,-8.8415656694));
#33058=CARTESIAN_POINT('Ctrl Pts',(8.960498394176,1.08889895505,-8.840709420371));
#33059=CARTESIAN_POINT('Ctrl Pts',(8.953072652207,1.088595839625,-8.840487779265));
#33060=CARTESIAN_POINT('Ctrl Pts',(9.302738927017,1.045272401126,-8.424305184978));
#33061=CARTESIAN_POINT('Ctrl Pts',(9.299441402642,1.045707964206,-8.427515806291));
#33062=CARTESIAN_POINT('Ctrl Pts',(9.275984179159,1.048694616249,-8.449692181949));
#33063=CARTESIAN_POINT('Ctrl Pts',(9.227956079129,1.053368806096,-8.486570150069));
#33064=CARTESIAN_POINT('Ctrl Pts',(9.152400046375,1.057476604153,-8.525604156071));
#33065=CARTESIAN_POINT('Ctrl Pts',(9.067739188484,1.058949108328,-8.551237183059));
#33066=CARTESIAN_POINT('Ctrl Pts',(9.002935177616,1.057788851816,-8.557738202339));
#33067=CARTESIAN_POINT('Ctrl Pts',(8.967315586458,1.056433026425,-8.557205961066));
#33068=CARTESIAN_POINT('Ctrl Pts',(8.962714824892,1.056245820989,-8.557068184064));
#33069=CARTESIAN_POINT('Origin',(9.295100309023,1.542473380275,-8.370118632984));
#33070=CARTESIAN_POINT('Ctrl Pts',(9.485442651867,1.647108267952,8.860081856811));
#33071=CARTESIAN_POINT('Ctrl Pts',(9.534636055674,1.64096510107,8.816948883762));
#33072=CARTESIAN_POINT('Ctrl Pts',(9.870608039504,1.598500395072,8.517369852702));
#33073=CARTESIAN_POINT('Ctrl Pts',(10.43190063343,1.521624710073,7.955944056789));
#33074=CARTESIAN_POINT('Ctrl Pts',(11.09326750931,1.42128421097,7.158960123002));
#33075=CARTESIAN_POINT('Ctrl Pts',(11.62445570885,1.33442407676,6.398723949699));
#33076=CARTESIAN_POINT('Ctrl Pts',(12.05012035755,1.260803969321,5.681200837573));
#33077=CARTESIAN_POINT('Ctrl Pts',(12.3950828246,1.198551710967,4.999467721285));
#33078=CARTESIAN_POINT('Ctrl Pts',(12.68374840675,1.144689166094,4.328719065733));
#33079=CARTESIAN_POINT('Ctrl Pts',(12.93020205058,1.097406293304,3.643458045457));
#33080=CARTESIAN_POINT('Ctrl Pts',(13.13571146032,1.057052001434,2.936359424241));
#33081=CARTESIAN_POINT('Ctrl Pts',(13.29688798186,1.024817639632,2.215855271431));
#33082=CARTESIAN_POINT('Ctrl Pts',(13.41249169134,1.00138297161,1.48878756032));
#33083=CARTESIAN_POINT('Ctrl Pts',(13.48260841803,0.9870409655564,0.7555736754422));
#33084=CARTESIAN_POINT('Ctrl Pts',(13.50680269221,0.982069625917,0.01877529667324));
#33085=CARTESIAN_POINT('Ctrl Pts',(13.48500661443,0.9865486686153,-0.7154601880356));
#33086=CARTESIAN_POINT('Ctrl Pts',(13.41819019154,1.000220349609,-1.441614172335));
#33087=CARTESIAN_POINT('Ctrl Pts',(13.30787595815,1.022599136136,-2.155736540013));
#33088=CARTESIAN_POINT('Ctrl Pts',(13.15767129232,1.052680207326,-2.845996704197));
#33089=CARTESIAN_POINT('Ctrl Pts',(12.97703907332,1.088248262002,-3.489954094899));
#33090=CARTESIAN_POINT('Ctrl Pts',(12.77682071924,1.12690535597,-4.077973333215));
#33091=CARTESIAN_POINT('Ctrl Pts',(12.55943682104,1.167989222857,-4.624788445562));
#33092=CARTESIAN_POINT('Ctrl Pts',(12.31876846793,1.2123926264,-5.153155013548));
#33093=CARTESIAN_POINT('Ctrl Pts',(12.05079729047,1.260473276706,-5.671685873951));
#33094=CARTESIAN_POINT('Ctrl Pts',(11.75644670744,1.311635180831,-6.177986581914));
#33095=CARTESIAN_POINT('Ctrl Pts',(11.4341748887,1.365674385277,-6.673870492724));
#33096=CARTESIAN_POINT('Ctrl Pts',(11.07534695527,1.423420589966,-7.169262308066));
#33097=CARTESIAN_POINT('Ctrl Pts',(10.66577646073,1.486219448941,-7.675934257889));
#33098=CARTESIAN_POINT('Ctrl Pts',(10.18588708925,1.555563635995,-8.204530961181));
#33099=CARTESIAN_POINT('Ctrl Pts',(9.78023156014,1.609923272329,-8.597955355053));
#33100=CARTESIAN_POINT('Ctrl Pts',(9.534645036012,1.640963964657,-8.816940683287));
#33101=CARTESIAN_POINT('Ctrl Pts',(9.485454699128,1.647106839676,-8.860071905716));
#33102=CARTESIAN_POINT('Ctrl Pts',(9.501283507643,1.340755486448,8.919478683582));
#33103=CARTESIAN_POINT('Ctrl Pts',(9.550507790226,1.334558254542,8.876058628521));
#33104=CARTESIAN_POINT('Ctrl Pts',(9.886690580984,1.291720690537,8.574485288614));
#33105=CARTESIAN_POINT('Ctrl Pts',(10.44833443549,1.214179980504,8.009317354798));
#33106=CARTESIAN_POINT('Ctrl Pts',(11.11011430115,1.112986469181,7.207011291774));
#33107=CARTESIAN_POINT('Ctrl Pts',(11.64163405682,1.025396523771,6.441690810591));
#33108=CARTESIAN_POINT('Ctrl Pts',(12.06756458097,0.9511628997746,5.719363221124));
#33109=CARTESIAN_POINT('Ctrl Pts',(12.41274280116,0.8883949022656,5.033060755404));
#33110=CARTESIAN_POINT('Ctrl Pts',(12.70158922282,0.8340880943174,4.357812662756));
#33111=CARTESIAN_POINT('Ctrl Pts',(12.94819754771,0.7864166089429,3.667951535326));
#33112=CARTESIAN_POINT('Ctrl Pts',(13.15383619157,0.74573159891,2.956103202327));
#33113=CARTESIAN_POINT('Ctrl Pts',(13.31511425316,0.7132336445999,2.230756755417));
#33114=CARTESIAN_POINT('Ctrl Pts',(13.43079090278,0.6896076458371,1.498800686597));
#33115=CARTESIAN_POINT('Ctrl Pts',(13.50095191817,0.6751486666702,0.7606557814507));
#33116=CARTESIAN_POINT('Ctrl Pts',(13.52516148339,0.6701368018972,0.01890158512833));
#33117=CARTESIAN_POINT('Ctrl Pts',(13.50335163006,0.6746523562059,-0.7202724951362));
#33118=CARTESIAN_POINT('Ctrl Pts',(13.43649300123,0.6884355387342,-1.451310075406));
#33119=CARTESIAN_POINT('Ctrl Pts',(13.32610915903,0.7109970198194,-2.170233874786));
#33120=CARTESIAN_POINT('Ctrl Pts',(13.17580985142,0.7413240355844,-2.86513326537));
#33121=CARTESIAN_POINT('Ctrl Pts',(12.99506401229,0.7771834854259,-3.513416598512));
#33122=CARTESIAN_POINT('Ctrl Pts',(12.79471993203,0.8161580465605,-4.105383881712));
#33123=CARTESIAN_POINT('Ctrl Pts',(12.57719973951,0.8575802200963,-4.655868321512));
#33124=CARTESIAN_POINT('Ctrl Pts',(12.33638070567,0.9023504074507,-5.187778254645));
#33125=CARTESIAN_POINT('Ctrl Pts',(12.068241961,0.9508297021305,-5.709784168435));
#33126=CARTESIAN_POINT('Ctrl Pts',(11.77370749238,1.002417669683,-6.219475482681));
#33127=CARTESIAN_POINT('Ctrl Pts',(11.45123446739,1.056909230048,-6.718677630099));
#33128=CARTESIAN_POINT('Ctrl Pts',(11.09218254538,1.115141808556,-7.217381559891));
#33129=CARTESIAN_POINT('Ctrl Pts',(10.68235630247,1.178473627838,-7.727437814332));
#33130=CARTESIAN_POINT('Ctrl Pts',(10.20216697086,1.248412121368,-8.25956136877));
#33131=CARTESIAN_POINT('Ctrl Pts',(9.796257394007,1.303243865608,-8.655607251179));
#33132=CARTESIAN_POINT('Ctrl Pts',(9.55051677653,1.334557108182,-8.876050373624));
#33133=CARTESIAN_POINT('Ctrl Pts',(9.501295562957,1.340754045595,-8.919468666609));
#33134=CARTESIAN_POINT('Ctrl Pts',(9.359979883938,1.092901517146,8.792071381238));
#33135=CARTESIAN_POINT('Ctrl Pts',(9.40827342587,1.086922770804,8.749258499761));
#33136=CARTESIAN_POINT('Ctrl Pts',(9.73810212497,1.045593549208,8.451901782226));
#33137=CARTESIAN_POINT('Ctrl Pts',(10.28915836763,0.9707608749562,7.89463319151));
#33138=CARTESIAN_POINT('Ctrl Pts',(10.93848999477,0.8730705639218,7.10356490815));
#33139=CARTESIAN_POINT('Ctrl Pts',(11.46001606517,0.7884977051436,6.349006483595));
#33140=CARTESIAN_POINT('Ctrl Pts',(11.87793263586,0.7168140964409,5.636885495828));
#33141=CARTESIAN_POINT('Ctrl Pts',(12.21660767664,0.6561993181206,4.960329573556));
#33142=CARTESIAN_POINT('Ctrl Pts',(12.50000327728,0.6037544207696,4.294718569006));
#33143=CARTESIAN_POINT('Ctrl Pts',(12.74194924295,0.5577172247791,3.614751118391));
#33144=CARTESIAN_POINT('Ctrl Pts',(12.94369254322,0.5184273359704,2.913159732911));
#33145=CARTESIAN_POINT('Ctrl Pts',(13.10191000897,0.487044227227,2.19830818232));
#33146=CARTESIAN_POINT('Ctrl Pts',(13.21538811471,0.4642290789812,1.476977936882));
#33147=CARTESIAN_POINT('Ctrl Pts',(13.28421419066,0.4502665148141,0.7495738144426));
#33148=CARTESIAN_POINT('Ctrl Pts',(13.30796285691,0.4454267556509,0.0186261527622));
#33149=CARTESIAN_POINT('Ctrl Pts',(13.28656822283,0.4497872467096,-0.7097786655537));
#33150=CARTESIAN_POINT('Ctrl Pts',(13.22098175535,0.4630972089924,-1.430177833726));
#33151=CARTESIAN_POINT('Ctrl Pts',(13.11269604486,0.4848843526421,-2.138662949869));
#33152=CARTESIAN_POINT('Ctrl Pts',(12.96524940725,0.5141709553425,-2.823504541799));
#33153=CARTESIAN_POINT('Ctrl Pts',(12.7879282788,0.5488006889822,-3.462440733503));
#33154=CARTESIAN_POINT('Ctrl Pts',(12.59137380672,0.5864390447853,-4.045907115348));
#33155=CARTESIAN_POINT('Ctrl Pts',(12.37796176471,0.6264411523485,-4.588517372372));
#33156=CARTESIAN_POINT('Ctrl Pts',(12.14168451331,0.6696761533601,-5.112848598301));
#33157=CARTESIAN_POINT('Ctrl Pts',(11.87859653892,0.716492108312,-5.627445918905));
#33158=CARTESIAN_POINT('Ctrl Pts',(11.58960470579,0.7663082323814,-6.129930166316));
#33159=CARTESIAN_POINT('Ctrl Pts',(11.27319639095,0.8189252214204,-6.622097308292));
#33160=CARTESIAN_POINT('Ctrl Pts',(10.92089587887,0.8751498914803,-7.113793976026));
#33161=CARTESIAN_POINT('Ctrl Pts',(10.51877834181,0.9362907877084,-7.616701069514));
#33162=CARTESIAN_POINT('Ctrl Pts',(10.04763033621,1.003798345438,-8.141379735601));
#33163=CARTESIAN_POINT('Ctrl Pts',(9.64937820522,1.056710983639,-8.531889495748));
#33164=CARTESIAN_POINT('Ctrl Pts',(9.408282232358,1.086921664791,-8.749250354908));
#33165=CARTESIAN_POINT('Ctrl Pts',(9.359991696511,1.092900125163,-8.792061502863));
#33166=CARTESIAN_POINT('Ctrl Pts',(9.152731006036,1.063514585851,8.560090305693));
#33167=CARTESIAN_POINT('Ctrl Pts',(9.1997329002,1.057885862191,8.518386975545));
#33168=CARTESIAN_POINT('Ctrl Pts',(9.520743623748,1.018972679307,8.228736347825));
#33169=CARTESIAN_POINT('Ctrl Pts',(10.05710676667,0.9484732995852,7.685910240827));
#33170=CARTESIAN_POINT('Ctrl Pts',(10.68916318457,0.8563813896063,6.915386634592));
#33171=CARTESIAN_POINT('Ctrl Pts',(11.19682038478,0.7766252477241,6.180490657665));
#33172=CARTESIAN_POINT('Ctrl Pts',(11.60361548453,0.709009372612,5.486999875077));
#33173=CARTESIAN_POINT('Ctrl Pts',(11.93326565123,0.6518270557176,4.828215841246));
#33174=CARTESIAN_POINT('Ctrl Pts',(12.20909680221,0.6023485409416,4.180158546027));
#33175=CARTESIAN_POINT('Ctrl Pts',(12.44457251662,0.5589137443474,3.51819304649));
#33176=CARTESIAN_POINT('Ctrl Pts',(12.64091000179,0.5218443864833,2.835245298414));
#33177=CARTESIAN_POINT('Ctrl Pts',(12.7948800848,0.4922350253254,2.139452289843));
#33178=CARTESIAN_POINT('Ctrl Pts',(12.90530713191,0.4707095752198,1.43740400211));
#33179=CARTESIAN_POINT('Ctrl Pts',(12.97228062783,0.4575364213677,0.7294802223117));
#33180=CARTESIAN_POINT('Ctrl Pts',(12.99538967536,0.4529703193238,0.01812676726228));
#33181=CARTESIAN_POINT('Ctrl Pts',(12.97457126737,0.4570842521421,-0.6907515555187));
#33182=CARTESIAN_POINT('Ctrl Pts',(12.91075025878,0.4696416949965,-1.39185647522));
#33183=CARTESIAN_POINT('Ctrl Pts',(12.80537625858,0.4901972368263,-2.081400057238));
#33184=CARTESIAN_POINT('Ctrl Pts',(12.66188845186,0.5178285651575,-2.747978261569));
#33185=CARTESIAN_POINT('Ctrl Pts',(12.4893200114,0.5505011463086,-3.369926996511));
#33186=CARTESIAN_POINT('Ctrl Pts',(12.29802461869,0.5860120288538,-3.937930124791));
#33187=CARTESIAN_POINT('Ctrl Pts',(12.0903137174,0.6237522271604,-4.466204790387));
#33188=CARTESIAN_POINT('Ctrl Pts',(11.86033938522,0.6645409012191,-4.976726634499));
#33189=CARTESIAN_POINT('Ctrl Pts',(11.60426068474,0.7087050737737,-5.477813319251));
#33190=CARTESIAN_POINT('Ctrl Pts',(11.32296071804,0.7556950186386,-5.967144362846));
#33191=CARTESIAN_POINT('Ctrl Pts',(11.0149687857,0.8053203822034,-6.446463742772));
#33192=CARTESIAN_POINT('Ctrl Pts',(10.6720376329,0.8583387921827,-6.925356351434));
#33193=CARTESIAN_POINT('Ctrl Pts',(10.28061795534,0.915978932676,-7.415194981312));
#33194=CARTESIAN_POINT('Ctrl Pts',(9.822017170651,0.9795992704055,-7.926262048838));
#33195=CARTESIAN_POINT('Ctrl Pts',(9.434391762418,1.029440205011,-8.306651162358));
#33196=CARTESIAN_POINT('Ctrl Pts',(9.199741457146,1.057884820781,-8.518379034178));
#33197=CARTESIAN_POINT('Ctrl Pts',(9.152742481741,1.063513272641,-8.560080680939));
#33198=CARTESIAN_POINT('',(9.631273226511,1.5424733773,8.740237221479));
#33199=CARTESIAN_POINT('Ctrl Pts',(9.63127322651082,1.5424733773,8.7402372214788));
#33200=CARTESIAN_POINT('Ctrl Pts',(9.76016736551745,1.52748192728802,8.62316346505574));
#33201=CARTESIAN_POINT('Ctrl Pts',(9.88367797190008,1.51265196794207,8.50577017900236));
#33202=CARTESIAN_POINT('Ctrl Pts',(10.0019313763767,1.49808103045733,8.38863411644834));
#33203=CARTESIAN_POINT('Ctrl Pts',(10.1221460058904,1.48326843492024,8.26955535990054));
#33204=CARTESIAN_POINT('Ctrl Pts',(10.2369277857404,1.46872349768402,8.15074250929634));
#33205=CARTESIAN_POINT('Ctrl Pts',(10.3464427733501,1.45452769271862,8.03276472333058));
#33206=CARTESIAN_POINT('Ctrl Pts',(10.380527813305,1.45010944285166,7.9960457532955));
#33207=CARTESIAN_POINT('Ctrl Pts',(10.4141028979157,1.44572486363172,7.95940740548168));
#33208=CARTESIAN_POINT('Ctrl Pts',(10.4471736310341,1.44137601424082,7.92286611309366));
#33209=CARTESIAN_POINT('Ctrl Pts',(10.536440168792,1.42963733499938,7.82423163030186));
#33210=CARTESIAN_POINT('Ctrl Pts',(10.6220293312436,1.41816178692121,7.72631349155243));
#33211=CARTESIAN_POINT('Ctrl Pts',(10.704297540876,1.40695201812211,7.62913681450109));
#33212=CARTESIAN_POINT('Ctrl Pts',(10.789095425202,1.39539755884562,7.52897204056718));
#33213=CARTESIAN_POINT('Ctrl Pts',(10.8703651110396,1.38412536211667,7.42959483382496));
#33214=CARTESIAN_POINT('Ctrl Pts',(10.9484674400921,1.37313074153775,7.33098567275051));
#33215=CARTESIAN_POINT('Ctrl Pts',(11.0015800711469,1.36565397056971,7.26392759581079));
#33216=CARTESIAN_POINT('Ctrl Pts',(11.053227327317,1.35830540981071,7.19722372438596));
#33217=CARTESIAN_POINT('Ctrl Pts',(11.1035148709274,1.35108206939083,7.1308567988699));
#33218=CARTESIAN_POINT('Ctrl Pts',(11.2015036679035,1.33700688521846,7.00153620129411));
#33219=CARTESIAN_POINT('Ctrl Pts',(11.2943246180977,1.32340992308326,6.87350257018018));
#33220=CARTESIAN_POINT('Ctrl Pts',(11.3823679190261,1.31031122879814,6.74706040500975));
#33221=CARTESIAN_POINT('Ctrl Pts',(11.4704112199545,1.29721253451303,6.62061823983932));
#33222=CARTESIAN_POINT('Ctrl Pts',(11.5536769978988,1.28461192973242,6.4957671084551));
#33223=CARTESIAN_POINT('Ctrl Pts',(11.6325422446539,1.27251585364215,6.37275783163964));
#33224=CARTESIAN_POINT('Ctrl Pts',(11.7130560730598,1.26016692385639,6.24717719614634));
#33225=CARTESIAN_POINT('Ctrl Pts',(11.788983030893,1.24834526068386,6.12351749166098));
#33226=CARTESIAN_POINT('Ctrl Pts',(11.8607187737643,1.23704304155025,6.0019887645426));
#33227=CARTESIAN_POINT('Ctrl Pts',(11.9295168292409,1.22620366542002,5.88543682299102));
#33228=CARTESIAN_POINT('Ctrl Pts',(11.9944598344691,1.21584188353946,5.77084425224909));
#33229=CARTESIAN_POINT('Ctrl Pts',(12.0558789256988,1.20594334387555,5.65835573107204));
#33230=CARTESIAN_POINT('Ctrl Pts',(12.1038310837798,1.19821518754449,5.57053177858779));
#33231=CARTESIAN_POINT('Ctrl Pts',(12.1496367114629,1.19077219983256,5.48399330909393));
#33232=CARTESIAN_POINT('Ctrl Pts',(12.1936278131294,1.18357376049498,5.39842189093468));
#33233=CARTESIAN_POINT('Ctrl Pts',(12.2386454394624,1.17620734683392,5.31085367869266));
#33234=CARTESIAN_POINT('Ctrl Pts',(12.2817628927706,1.16909695753592,5.22429795088912));
#33235=CARTESIAN_POINT('Ctrl Pts',(12.3232908005036,1.16220259249432,5.13838260493158));
#33236=CARTESIAN_POINT('Ctrl Pts',(12.3473569046407,1.15820719479413,5.08859325180347));
#33237=CARTESIAN_POINT('Ctrl Pts',(12.3708883419127,1.15428441754086,5.03901841395892));
#33238=CARTESIAN_POINT('Ctrl Pts',(12.3939388048181,1.15042713724629,4.98958152163347));
#33239=CARTESIAN_POINT('Ctrl Pts',(12.4317412300487,1.14410125344399,4.90850573441675));
#33240=CARTESIAN_POINT('Ctrl Pts',(12.4682510143418,1.13795307997892,4.82780619813583));
#33241=CARTESIAN_POINT('Ctrl Pts',(12.5037313437523,1.13194537250749,4.74700117092273));
#33242=CARTESIAN_POINT('Ctrl Pts',(12.5392814814001,1.12592584475489,4.66603715824885));
#33243=CARTESIAN_POINT('Ctrl Pts',(12.5737981464946,1.12004727777973,4.58496704665721));
#33244=CARTESIAN_POINT('Ctrl Pts',(12.6074992630549,1.11427866384779,4.50328422139707));
#33245=CARTESIAN_POINT('Ctrl Pts',(12.6306462071191,1.11031660568355,4.4471819915516));
#33246=CARTESIAN_POINT('Ctrl Pts',(12.653407468017,1.10640654850001,4.39079027065877));
#33247=CARTESIAN_POINT('Ctrl Pts',(12.6758406044922,1.1025404436147,4.33393955596147));
#33248=CARTESIAN_POINT('Ctrl Pts',(12.7274812603864,1.09364074328731,4.20307028593055));
#33249=CARTESIAN_POINT('Ctrl Pts',(12.7773728839536,1.08496340147549,4.06976945161404));
#33250=CARTESIAN_POINT('Ctrl Pts',(12.8252096589171,1.07658322740027,3.93441410555896));
#33251=CARTESIAN_POINT('Ctrl Pts',(12.8586060667958,1.07073275542085,3.83991813778412));
#33252=CARTESIAN_POINT('Ctrl Pts',(12.8910018140696,1.06502704983544,3.74442145063781));
#33253=CARTESIAN_POINT('Ctrl Pts',(12.9223056969685,1.0594901363143,3.64806012546232));
#33254=CARTESIAN_POINT('Ctrl Pts',(12.9568881477048,1.05337332199786,3.54160653337837));
#33255=CARTESIAN_POINT('Ctrl Pts',(12.9901360722762,1.04746035389728,3.43409399001926));
#33256=CARTESIAN_POINT('Ctrl Pts',(13.0218729325533,1.04178927772019,3.32598947361619));
#33257=CARTESIAN_POINT('Ctrl Pts',(13.0535488749454,1.03612908699186,3.21809246036381));
#33258=CARTESIAN_POINT('Ctrl Pts',(13.0837194710999,1.03070992177902,3.10960598071963));
#33259=CARTESIAN_POINT('Ctrl Pts',(13.1122581627635,1.02556110406422,3.00100968818389));
#33260=CARTESIAN_POINT('Ctrl Pts',(13.1180829828847,1.02451021717076,2.97884490651453));
#33261=CARTESIAN_POINT('Ctrl Pts',(13.1238399864087,1.02347056232403,2.95667559452744));
#33262=CARTESIAN_POINT('Ctrl Pts',(13.1295283518426,1.02244234182423,2.93450589513787));
#33263=CARTESIAN_POINT('Ctrl Pts',(13.1668836820405,1.0156900477369,2.78891812467845));
#33264=CARTESIAN_POINT('Ctrl Pts',(13.2012838387308,1.00943843149588,2.64331335810838));
#33265=CARTESIAN_POINT('Ctrl Pts',(13.2328430798278,1.00367908012121,2.49748776573468));
#33266=CARTESIAN_POINT('Ctrl Pts',(13.2532264254349,0.999959255262895,2.40330256531842));
#33267=CARTESIAN_POINT('Ctrl Pts',(13.2724236824129,0.996444944216602,2.30902485890701));
#33268=CARTESIAN_POINT('Ctrl Pts',(13.2904547716062,0.993135801902423,2.21459634085511));
#33269=CARTESIAN_POINT('Ctrl Pts',(13.3214594197414,0.98744569677451,2.05222550763766));
#33270=CARTESIAN_POINT('Ctrl Pts',(13.3490176029642,0.982361156275227,1.88941172405413));
#33271=CARTESIAN_POINT('Ctrl Pts',(13.3731643781013,0.977892034139776,1.72600340806214));
#33272=CARTESIAN_POINT('Ctrl Pts',(13.3848027163602,0.975737992664778,1.6472433564596));
#33273=CARTESIAN_POINT('Ctrl Pts',(13.3956478126217,0.97372706051493,1.56834503918377));
#33274=CARTESIAN_POINT('Ctrl Pts',(13.4056993955901,0.971861166161085,1.48929083180983));
#33275=CARTESIAN_POINT('Ctrl Pts',(13.4366056150463,0.96612398620019,1.2462180054005));
#33276=CARTESIAN_POINT('Ctrl Pts',(13.4600071666758,0.961754442251598,1.00167097719576));
#33277=CARTESIAN_POINT('Ctrl Pts',(13.4757625271622,0.958810186936582,0.75615674000873));
#33278=CARTESIAN_POINT('Ctrl Pts',(13.4870314438372,0.956704327927927,0.580554316707783));
#33279=CARTESIAN_POINT('Ctrl Pts',(13.4943847641842,0.955326771075483,0.404456792494881));
#33280=CARTESIAN_POINT('Ctrl Pts',(13.4977916921877,0.954688412324058,0.228331189878502));
#33281=CARTESIAN_POINT('Ctrl Pts',(13.499148077322,0.95443426538586,0.158211084932178));
#33282=CARTESIAN_POINT('Ctrl Pts',(13.4998795101869,0.954297167785211,0.0880865669065382));
#33283=CARTESIAN_POINT('Ctrl Pts',(13.4999862992676,0.954277342264801,0.0179871712228238));
#33284=CARTESIAN_POINT('Ctrl Pts',(13.5002265334807,0.95423274249614,-0.13970941207456));
#33285=CARTESIAN_POINT('Ctrl Pts',(13.4973018794775,0.954781650237799,-0.29727994041566));
#33286=CARTESIAN_POINT('Ctrl Pts',(13.4912574586599,0.955912892086901,-0.454274314967719));
#33287=CARTESIAN_POINT('Ctrl Pts',(13.4878662083785,0.956547580563249,-0.542356735591353));
#33288=CARTESIAN_POINT('Ctrl Pts',(13.4834938311073,0.957365388509113,-0.630257845020122));
#33289=CARTESIAN_POINT('Ctrl Pts',(13.4781552909154,0.95836291423459,-0.717898947514517));
#33290=CARTESIAN_POINT('Ctrl Pts',(13.4661608904116,0.960604111759422,-0.914807174507933));
#33291=CARTESIAN_POINT('Ctrl Pts',(13.4492956345586,0.963755902347615,-1.11040352667427));
#33292=CARTESIAN_POINT('Ctrl Pts',(13.4276955991877,0.967773971019727,-1.30468906634728));
#33293=CARTESIAN_POINT('Ctrl Pts',(13.4225463984485,0.968731832514913,-1.35100451108217));
#33294=CARTESIAN_POINT('Ctrl Pts',(13.4171278995042,0.969738972562947,-1.39724550214024));
#33295=CARTESIAN_POINT('Ctrl Pts',(13.4114415260978,0.970794881126638,-1.44341211566292));
#33296=CARTESIAN_POINT('Ctrl Pts',(13.3924576987589,0.974320007674985,-1.59753829720194));
#33297=CARTESIAN_POINT('Ctrl Pts',(13.3704926452548,0.978389043240586,-1.75083401852059));
#33298=CARTESIAN_POINT('Ctrl Pts',(13.3455542466026,0.98299168568862,-1.90350363273298));
#33299=CARTESIAN_POINT('Ctrl Pts',(13.3316872845961,0.985550978642689,-1.98839536011907));
#33300=CARTESIAN_POINT('Ctrl Pts',(13.3169000816878,0.988275444713513,-2.07309342852308));
#33301=CARTESIAN_POINT('Ctrl Pts',(13.3011872234493,0.991164664440456,-2.15763205493448));
#33302=CARTESIAN_POINT('Ctrl Pts',(13.2817749696322,0.994734114748057,-2.2620742416032));
#33303=CARTESIAN_POINT('Ctrl Pts',(13.2609449552185,0.998551087536764,-2.3662727735945));
#33304=CARTESIAN_POINT('Ctrl Pts',(13.2388164250053,1.00259155889224,-2.46972511079396));
#33305=CARTESIAN_POINT('Ctrl Pts',(13.2165454097734,1.00665804673552,-2.57384357484662));
#33306=CARTESIAN_POINT('Ctrl Pts',(13.1929591758184,1.01095087186728,-2.67720597429563));
#33307=CARTESIAN_POINT('Ctrl Pts',(13.168229649725,1.01543629733027,-2.77931309282663));
#33308=CARTESIAN_POINT('Ctrl Pts',(13.1618737206253,1.01658913164328,-2.8055564427198));
#33309=CARTESIAN_POINT('Ctrl Pts',(13.1554425213489,1.01775464375683,-2.83171694779066));
#33310=CARTESIAN_POINT('Ctrl Pts',(13.1489394909979,1.01893216973745,-2.85778629807699));
#33311=CARTESIAN_POINT('Ctrl Pts',(13.1263239080982,1.02302725079878,-2.94844765451032));
#33312=CARTESIAN_POINT('Ctrl Pts',(13.1028347601488,1.02726732550112,-3.03800882211687));
#33313=CARTESIAN_POINT('Ctrl Pts',(13.0787022721279,1.03160637240792,-3.12591046701909));
#33314=CARTESIAN_POINT('Ctrl Pts',(13.0539550821271,1.0360559433818,-3.21605113987043));
#33315=CARTESIAN_POINT('Ctrl Pts',(13.0285314995321,1.04060952686829,-3.30444647936617));
#33316=CARTESIAN_POINT('Ctrl Pts',(13.0027308146993,1.0452092509767,-3.39051297959414));
#33317=CARTESIAN_POINT('Ctrl Pts',(12.9903401839258,1.04741824207352,-3.43184592223512));
#33318=CARTESIAN_POINT('Ctrl Pts',(12.9778633112975,1.04963776091173,-3.47264205963787));
#33319=CARTESIAN_POINT('Ctrl Pts',(12.9653371636099,1.0518608243978,-3.51283847920185));
#33320=CARTESIAN_POINT('Ctrl Pts',(12.9397525056021,1.05640143180874,-3.59493967051231));
#33321=CARTESIAN_POINT('Ctrl Pts',(12.9139675330497,1.06096428172172,-3.67453971736313));
#33322=CARTESIAN_POINT('Ctrl Pts',(12.8879510802549,1.06555104034565,-3.7521646067085));
#33323=CARTESIAN_POINT('Ctrl Pts',(12.8611841832938,1.07027010394901,-3.83202858475043));
#33324=CARTESIAN_POINT('Ctrl Pts',(12.8341721013302,1.07501454269927,-3.90980195282997));
#33325=CARTESIAN_POINT('Ctrl Pts',(12.8068280574077,1.07979620072513,-3.98604480334464));
#33326=CARTESIAN_POINT('Ctrl Pts',(12.7942204177638,1.08200090100504,-4.02119843268463));
#33327=CARTESIAN_POINT('Ctrl Pts',(12.7815414973675,1.08421364481377,-4.05602650238246));
#33328=CARTESIAN_POINT('Ctrl Pts',(12.768779288753,1.0864362255717,-4.09058291631843));
#33329=CARTESIAN_POINT('Ctrl Pts',(12.7416044788988,1.09116880841115,-4.1641645357952));
#33330=CARTESIAN_POINT('Ctrl Pts',(12.714056646962,1.09594489502114,-4.23651208758985));
#33331=CARTESIAN_POINT('Ctrl Pts',(12.6859506057501,1.10079561217221,-4.30823009812429));
#33332=CARTESIAN_POINT('Ctrl Pts',(12.6576888991591,1.10567319503226,-4.38034531903806));
#33333=CARTESIAN_POINT('Ctrl Pts',(12.6288626839948,1.11062629594105,-4.45182414645006));
#33334=CARTESIAN_POINT('Ctrl Pts',(12.5992351970053,1.1156943322581,-4.52326269754378));
#33335=CARTESIAN_POINT('Ctrl Pts',(12.5853084146409,1.11807662809128,-4.55684330982678));
#33336=CARTESIAN_POINT('Ctrl Pts',(12.5712039002858,1.12048442557025,-4.59041474515251));
#33337=CARTESIAN_POINT('Ctrl Pts',(12.5568934393279,1.12292235830783,-4.62403736370218));
#33338=CARTESIAN_POINT('Ctrl Pts',(12.5157966851936,1.12992360883407,-4.72059473470175));
#33339=CARTESIAN_POINT('Ctrl Pts',(12.4729962079317,1.13716536282956,-4.81757125875771));
#33340=CARTESIAN_POINT('Ctrl Pts',(12.4286427289522,1.14461307353984,-4.91446457153812));
#33341=CARTESIAN_POINT('Ctrl Pts',(12.392020208736,1.15076262352617,-4.99446905794523));
#33342=CARTESIAN_POINT('Ctrl Pts',(12.3543397615075,1.15705242076176,-5.07441703357359));
#33343=CARTESIAN_POINT('Ctrl Pts',(12.3157108673077,1.1634592045548,-5.15403561069008));
#33344=CARTESIAN_POINT('Ctrl Pts',(12.263417077726,1.1721323755194,-5.26181910293787));
#33345=CARTESIAN_POINT('Ctrl Pts',(12.2093834549275,1.18102122084978,-5.36900096619964));
#33346=CARTESIAN_POINT('Ctrl Pts',(12.1538263915905,1.19007320817802,-5.47515194145451));
#33347=CARTESIAN_POINT('Ctrl Pts',(12.1186412076037,1.19580597770291,-5.54237906561095));
#33348=CARTESIAN_POINT('Ctrl Pts',(12.0828459295794,1.20160405362024,-5.60919316153846));
#33349=CARTESIAN_POINT('Ctrl Pts',(12.0465049645459,1.20745299121237,-5.67549034442851));
#33350=CARTESIAN_POINT('Ctrl Pts',(11.9921789271359,1.21619655655648,-5.77459787320605));
#33351=CARTESIAN_POINT('Ctrl Pts',(11.9366389356514,1.2250554615878,-5.87255244596524));
#33352=CARTESIAN_POINT('Ctrl Pts',(11.8796989992141,1.23404685830823,-5.96971786588508));
#33353=CARTESIAN_POINT('Ctrl Pts',(11.8384064553275,1.24056737214985,-6.04018171985728));
#33354=CARTESIAN_POINT('Ctrl Pts',(11.7963766993591,1.24715769405327,-6.11023007401325));
#33355=CARTESIAN_POINT('Ctrl Pts',(11.7535240951848,1.25382589389963,-6.17999300576206));
#33356=CARTESIAN_POINT('Ctrl Pts',(11.6791717591893,1.26539569799939,-6.30103668656892));
#33357=CARTESIAN_POINT('Ctrl Pts',(11.6023431512998,1.27719852979548,-6.42122091795169));
#33358=CARTESIAN_POINT('Ctrl Pts',(11.522831796062,1.28923292277853,-6.54072032768313));
#33359=CARTESIAN_POINT('Ctrl Pts',(11.4933258998355,1.29369876981941,-6.58506540483728));
#33360=CARTESIAN_POINT('Ctrl Pts',(11.4634501712187,1.29819651733763,-6.6293158522582));
#33361=CARTESIAN_POINT('Ctrl Pts',(11.4331926690046,1.30272611517905,-6.67347939649423));
#33362=CARTESIAN_POINT('Ctrl Pts',(11.3801106222787,1.31067258486998,-6.75095741507395));
#33363=CARTESIAN_POINT('Ctrl Pts',(11.3258574716049,1.3187173628309,-6.82816947322432));
#33364=CARTESIAN_POINT('Ctrl Pts',(11.270099910585,1.32689750593474,-6.90550130181125));
#33365=CARTESIAN_POINT('Ctrl Pts',(11.2151048678493,1.33496578064673,-6.98177557098961));
#33366=CARTESIAN_POINT('Ctrl Pts',(11.1586462082761,1.34316582874487,-7.05816654327559));
#33367=CARTESIAN_POINT('Ctrl Pts',(11.1003648662286,1.35153426861603,-7.13501209334715));
#33368=CARTESIAN_POINT('Ctrl Pts',(11.0932894453453,1.35255020668719,-7.14434123009419));
#33369=CARTESIAN_POINT('Ctrl Pts',(11.0861871138464,1.35356862693456,-7.15367702482475));
#33370=CARTESIAN_POINT('Ctrl Pts',(11.0790571897794,1.35458959500383,-7.16302004684974));
#33371=CARTESIAN_POINT('Ctrl Pts',(11.0163547803249,1.36356825414787,-7.24518501621748));
#33372=CARTESIAN_POINT('Ctrl Pts',(10.9515226474709,1.37274293502362,-7.32791024198651));
#33373=CARTESIAN_POINT('Ctrl Pts',(10.8841959067605,1.38214071339441,-7.41140804188175));
#33374=CARTESIAN_POINT('Ctrl Pts',(10.8168691660501,1.3915384917652,-7.494905841777));
#33375=CARTESIAN_POINT('Ctrl Pts',(10.7470478932044,1.40115948398462,-7.5791766228846));
#33376=CARTESIAN_POINT('Ctrl Pts',(10.6743311014899,1.41102779561278,-7.66439154289842));
#33377=CARTESIAN_POINT('Ctrl Pts',(10.609071748101,1.41988406691836,-7.74086728458169));
#33378=CARTESIAN_POINT('Ctrl Pts',(10.5414820399865,1.42893856155155,-7.81810198386333));
#33379=CARTESIAN_POINT('Ctrl Pts',(10.4711762902307,1.43821456689777,-7.89626316965109));
#33380=CARTESIAN_POINT('Ctrl Pts',(10.402894830669,1.44722349129075,-7.97217388627369));
#33381=CARTESIAN_POINT('Ctrl Pts',(10.3320514165358,1.45644144668458,-8.04895869510814));
#33382=CARTESIAN_POINT('Ctrl Pts',(10.2582624312653,1.46588546680312,-8.12673235594464));
#33383=CARTESIAN_POINT('Ctrl Pts',(10.2387105952778,1.46838784479006,-8.14734000971909));
#33384=CARTESIAN_POINT('Ctrl Pts',(10.2189517878589,1.4709060662173,-8.16801686462112));
#33385=CARTESIAN_POINT('Ctrl Pts',(10.1989785098382,1.47344038183622,-8.18876455273126));
#33386=CARTESIAN_POINT('Ctrl Pts',(10.0991791609495,1.48610345338535,-8.29243335272441));
#33387=CARTESIAN_POINT('Ctrl Pts',(9.99402608080279,1.49916870374078,-8.39786818195577));
#33388=CARTESIAN_POINT('Ctrl Pts',(9.88340877548464,1.51255465483016,-8.50440623974693));
#33389=CARTESIAN_POINT('Ctrl Pts',(9.80230993319642,1.52236853642087,-8.58251439038075));
#33390=CARTESIAN_POINT('Ctrl Pts',(9.71827471455824,1.53235440715854,-8.66121489978216));
#33391=CARTESIAN_POINT('Ctrl Pts',(9.63127322649984,1.542473377301,-8.74023722148882));
#33392=CARTESIAN_POINT('Origin',(9.295100333713,1.542473377277,8.37011861056));
#33393=CARTESIAN_POINT('Origin',(1.692653696601,0.,0.));
#33394=CARTESIAN_POINT('',(9.63127320811535,6.05752662000828,8.74023723818668));
#33395=CARTESIAN_POINT('Ctrl Pts',(9.63127322650206,6.057526622699,-8.74023722148816));
#33396=CARTESIAN_POINT('Ctrl Pts',(9.76588086213937,6.0731825242371,-8.61797523041577));
#33397=CARTESIAN_POINT('Ctrl Pts',(9.89461857444399,6.08865437321686,-8.49536863500099));
#33398=CARTESIAN_POINT('Ctrl Pts',(10.0176281064609,6.10384611849948,-8.37306561562682));
#33399=CARTESIAN_POINT('Ctrl Pts',(10.1431176997746,6.11934415272484,-8.24829677933693));
#33400=CARTESIAN_POINT('Ctrl Pts',(10.2626461575767,6.13455067475198,-8.12384421773691));
#33401=CARTESIAN_POINT('Ctrl Pts',(10.37640803786,6.14936370590824,-8.00036482099906));
#33402=CARTESIAN_POINT('Ctrl Pts',(10.400201994996,6.15246193729742,-7.97453838893019));
#33403=CARTESIAN_POINT('Ctrl Pts',(10.4237438262894,6.15554295497639,-7.94875441217995));
#33404=CARTESIAN_POINT('Ctrl Pts',(10.447035525501,6.15860582586468,-7.92301871272803));
#33405=CARTESIAN_POINT('Ctrl Pts',(10.5370129321437,6.1704379029023,-7.82359996814539));
#33406=CARTESIAN_POINT('Ctrl Pts',(10.6232564765674,6.18199917010837,-7.72490907933849));
#33407=CARTESIAN_POINT('Ctrl Pts',(10.7061287125036,6.19329278823122,-7.62697153961611));
#33408=CARTESIAN_POINT('Ctrl Pts',(10.7912441069049,6.20489209830034,-7.52638305873346));
#33409=CARTESIAN_POINT('Ctrl Pts',(10.872803393278,6.21620907391581,-7.42658905138719));
#33410=CARTESIAN_POINT('Ctrl Pts',(10.951172069922,6.22724713949817,-7.32756878229688));
#33411=CARTESIAN_POINT('Ctrl Pts',(11.0032593022312,6.23458351814911,-7.2617556030995));
#33412=CARTESIAN_POINT('Ctrl Pts',(11.0539365063572,6.24179668801535,-7.19628323082759));
#33413=CARTESIAN_POINT('Ctrl Pts',(11.103304087683,6.24888765453051,-7.13113496894025));
#33414=CARTESIAN_POINT('Ctrl Pts',(11.2012859035996,6.26296137977892,-7.0018326042689));
#33415=CARTESIAN_POINT('Ctrl Pts',(11.2941025393094,6.27655372243322,-6.87381566679909));
#33416=CARTESIAN_POINT('Ctrl Pts',(11.3821420721327,6.28965154729957,-6.7473877722308));
#33417=CARTESIAN_POINT('Ctrl Pts',(11.470181604956,6.30274937216593,-6.6209598776625));
#33418=CARTESIAN_POINT('Ctrl Pts',(11.5534442861599,6.31535267924435,-6.49612068475505));
#33419=CARTESIAN_POINT('Ctrl Pts',(11.6323087423303,6.32744833334101,-6.37312202145236));
#33420=CARTESIAN_POINT('Ctrl Pts',(11.7139317330224,6.3399670713085,-6.24582108973488));
#33421=CARTESIAN_POINT('Ctrl Pts',(11.7908429946487,6.35194202164803,-6.12049296792028));
#33422=CARTESIAN_POINT('Ctrl Pts',(11.8634519252431,6.36338559571308,-5.99735692790288));
#33423=CARTESIAN_POINT('Ctrl Pts',(11.9311530660119,6.37405567461845,-5.88254391095459));
#33424=CARTESIAN_POINT('Ctrl Pts',(11.9951137821112,6.38426378322768,-5.769635897331));
#33425=CARTESIAN_POINT('Ctrl Pts',(12.0556513233948,6.39401998244428,-5.65877256262166));
#33426=CARTESIAN_POINT('Ctrl Pts',(12.1038652840376,6.40179011970257,-5.57047759154957));
#33427=CARTESIAN_POINT('Ctrl Pts',(12.1499093874645,6.40927360994193,-5.48348278526444));
#33428=CARTESIAN_POINT('Ctrl Pts',(12.1941193727415,6.41650884040827,-5.39746657064736));
#33429=CARTESIAN_POINT('Ctrl Pts',(12.239347841141,6.4239107517742,-5.30946876607293));
#33430=CARTESIAN_POINT('Ctrl Pts',(12.2826567466982,6.43105283309077,-5.22249493248192));
#33431=CARTESIAN_POINT('Ctrl Pts',(12.3243602954384,6.4379761862191,-5.13616992754827));
#33432=CARTESIAN_POINT('Ctrl Pts',(12.3479705506366,6.44189580790898,-5.08729745846498));
#33433=CARTESIAN_POINT('Ctrl Pts',(12.371065438676,6.44574532280715,-5.03863241735876));
#33434=CARTESIAN_POINT('Ctrl Pts',(12.3936956904151,6.44953218929337,-4.99010290224972));
#33435=CARTESIAN_POINT('Ctrl Pts',(12.4316423719943,6.45588205311251,-4.908728020597));
#33436=CARTESIAN_POINT('Ctrl Pts',(12.4682836359117,6.46205576845061,-4.82773956322418));
#33437=CARTESIAN_POINT('Ctrl Pts',(12.5038861066545,6.46808556494792,-4.74664939765116));
#33438=CARTESIAN_POINT('Ctrl Pts',(12.5395883311841,6.47413225620062,-4.6653320273106));
#33439=CARTESIAN_POINT('Ctrl Pts',(12.574245978718,6.48003422099657,-4.58391218210168));
#33440=CARTESIAN_POINT('Ctrl Pts',(12.6080804843132,6.48582396064637,-4.50187569469749));
#33441=CARTESIAN_POINT('Ctrl Pts',(12.6309096503538,6.48973047340522,-4.44652319111007));
#33442=CARTESIAN_POINT('Ctrl Pts',(12.6533631014863,6.49358589443462,-4.39088950817029));
#33443=CARTESIAN_POINT('Ctrl Pts',(12.6754964142268,6.4974002074343,-4.33481171082529));
#33444=CARTESIAN_POINT('Ctrl Pts',(12.7269620283516,6.50626946091183,-4.20441648653281));
#33445=CARTESIAN_POINT('Ctrl Pts',(12.7766868579223,6.5149164508941,-4.07162023955325));
#33446=CARTESIAN_POINT('Ctrl Pts',(12.8243735059259,6.52326975856373,-3.93678051396021));
#33447=CARTESIAN_POINT('Ctrl Pts',(12.8578991816006,6.52914247756301,-3.84198263871521));
#33448=CARTESIAN_POINT('Ctrl Pts',(12.8904183033638,6.53487003912974,-3.74617535806888));
#33449=CARTESIAN_POINT('Ctrl Pts',(12.9218408197293,6.5404276259437,-3.64949082505811));
#33450=CARTESIAN_POINT('Ctrl Pts',(12.9562541218577,6.54651418221784,-3.5436038869485));
#33451=CARTESIAN_POINT('Ctrl Pts',(12.989350143959,6.5523968676152,-3.4366610057836));
#33452=CARTESIAN_POINT('Ctrl Pts',(13.0209525658403,6.5580429985623,-3.32912472845405));
#33453=CARTESIAN_POINT('Ctrl Pts',(13.0525173160842,6.56368239904426,-3.22171663964358));
#33454=CARTESIAN_POINT('Ctrl Pts',(13.0825919425141,6.56908580870885,-3.11371679794506));
#33455=CARTESIAN_POINT('Ctrl Pts',(13.1110505414873,6.57422066072457,-3.00560147409868));
#33456=CARTESIAN_POINT('Ctrl Pts',(13.1171211402712,6.57531599315578,-2.98253903331994));
#33457=CARTESIAN_POINT('Ctrl Pts',(13.1231183881254,6.57639910552087,-2.95947138618505));
#33458=CARTESIAN_POINT('Ctrl Pts',(13.1290413604535,6.57746968171617,-2.93640323022847));
#33459=CARTESIAN_POINT('Ctrl Pts',(13.1676212352864,6.58444298723336,-2.786146480723));
#33460=CARTESIAN_POINT('Ctrl Pts',(13.2030547578354,6.59088442080034,-2.63586799647866));
#33461=CARTESIAN_POINT('Ctrl Pts',(13.2354636382202,6.59679996185767,-2.48535015240714));
#33462=CARTESIAN_POINT('Ctrl Pts',(13.2547085157596,6.60031269854823,-2.39597040703327));
#33463=CARTESIAN_POINT('Ctrl Pts',(13.2728859159242,6.60363999702594,-2.30650590690212));
#33464=CARTESIAN_POINT('Ctrl Pts',(13.2900130167678,6.60678310931848,-2.21690855187006));
#33465=CARTESIAN_POINT('Ctrl Pts',(13.3222777813736,6.61270423859626,-2.04812122494202));
#33466=CARTESIAN_POINT('Ctrl Pts',(13.3508170882143,6.61797171624897,-1.87886546720217));
#33467=CARTESIAN_POINT('Ctrl Pts',(13.3756691945126,6.62257209353774,-1.70896916413712));
#33468=CARTESIAN_POINT('Ctrl Pts',(13.386225408693,6.62452615599781,-1.63680378136887));
#33469=CARTESIAN_POINT('Ctrl Pts',(13.3961157384593,6.62635985874055,-1.5645227116085));
#33470=CARTESIAN_POINT('Ctrl Pts',(13.4053402988285,6.62807217110335,-1.49211235716791));
#33471=CARTESIAN_POINT('Ctrl Pts',(13.4362819019681,6.63381571740367,-1.2492289718761));
#33472=CARTESIAN_POINT('Ctrl Pts',(13.4597283165912,6.63819349065334,-1.00489014817131));
#33473=CARTESIAN_POINT('Ctrl Pts',(13.4755417506912,6.64114854912334,-0.759589252947098));
#33474=CARTESIAN_POINT('Ctrl Pts',(13.4865389940783,6.64320360541361,-0.588997992957664));
#33475=CARTESIAN_POINT('Ctrl Pts',(13.4938417996689,6.64457059089948,-0.417941196048216));
#33476=CARTESIAN_POINT('Ctrl Pts',(13.4974195660371,6.64524136211976,-0.24683900869035));
#33477=CARTESIAN_POINT('Ctrl Pts',(13.4989864318914,6.64553512320223,-0.171905615231797));
#33478=CARTESIAN_POINT('Ctrl Pts',(13.4998395222726,6.64569535313262,-0.0969635614458784));
#33479=CARTESIAN_POINT('Ctrl Pts',(13.4999794142971,6.64572136789133,-0.0220482345393076));
#33480=CARTESIAN_POINT('Ctrl Pts',(13.5002684457918,6.64577511709272,0.132734634566845));
#33481=CARTESIAN_POINT('Ctrl Pts',(13.4975093177643,6.64525593039062,0.287404480942835));
#33482=CARTESIAN_POINT('Ctrl Pts',(13.4917413597792,6.64417678722204,0.441539403733856));
#33483=CARTESIAN_POINT('Ctrl Pts',(13.4883430531217,6.64354098865631,0.532351045500931));
#33484=CARTESIAN_POINT('Ctrl Pts',(13.4839013085648,6.6427108174116,0.622977047436292));
#33485=CARTESIAN_POINT('Ctrl Pts',(13.4784325941184,6.64168892795466,0.713331975483202));
#33486=CARTESIAN_POINT('Ctrl Pts',(13.4653273546151,6.63924006977958,0.929858726693208));
#33487=CARTESIAN_POINT('Ctrl Pts',(13.4463315506767,6.63569022305755,1.14482941200399));
#33488=CARTESIAN_POINT('Ctrl Pts',(13.4216193971161,6.6310961576815,1.35823058592934));
#33489=CARTESIAN_POINT('Ctrl Pts',(13.4185164456516,6.63051930945774,1.38502604442876));
#33490=CARTESIAN_POINT('Ctrl Pts',(13.4153233038083,6.62992599780766,1.41179677541527));
#33491=CARTESIAN_POINT('Ctrl Pts',(13.4120402606657,6.62931633511701,1.43854276628595));
#33492=CARTESIAN_POINT('Ctrl Pts',(13.3926244347943,6.6257108069141,1.59671781271477));
#33493=CARTESIAN_POINT('Ctrl Pts',(13.3700688387817,6.6215333999691,1.75402610638057));
#33494=CARTESIAN_POINT('Ctrl Pts',(13.3443776216534,6.61679181905033,1.91069524068469));
#33495=CARTESIAN_POINT('Ctrl Pts',(13.3311274780926,6.61434636745629,1.99149672668338));
#33496=CARTESIAN_POINT('Ctrl Pts',(13.3170424290057,6.61175084898136,2.07212813769992));
#33497=CARTESIAN_POINT('Ctrl Pts',(13.3021176699024,6.60900632060681,2.15262002709032));
#33498=CARTESIAN_POINT('Ctrl Pts',(13.282699452721,6.60543548588387,2.2573459378208));
#33499=CARTESIAN_POINT('Ctrl Pts',(13.2618549081864,6.60161240813343,2.36183523166039));
#33500=CARTESIAN_POINT('Ctrl Pts',(13.2397008743149,6.59756647754478,2.46558881488019));
#33501=CARTESIAN_POINT('Ctrl Pts',(13.2174151238934,6.59349649192299,2.56995926381932));
#33502=CARTESIAN_POINT('Ctrl Pts',(13.1938043422287,6.58920099564749,2.67358500413981));
#33503=CARTESIAN_POINT('Ctrl Pts',(13.1690386693525,6.58470990624757,2.77597094466383));
#33504=CARTESIAN_POINT('Ctrl Pts',(13.1628121938078,6.58358077648569,2.80171236335964));
#33505=CARTESIAN_POINT('Ctrl Pts',(13.1565129652826,6.58243928332459,2.82737548734641));
#33506=CARTESIAN_POINT('Ctrl Pts',(13.1501441803073,6.58128590221134,2.85295260111209));
#33507=CARTESIAN_POINT('Ctrl Pts',(13.1276352530914,6.57720955615299,2.94334871189015));
#33508=CARTESIAN_POINT('Ctrl Pts',(13.1042526433213,6.57298471795363,3.03267264726758));
#33509=CARTESIAN_POINT('Ctrl Pts',(13.0802238691335,6.56866270647682,3.12036412844092));
#33510=CARTESIAN_POINT('Ctrl Pts',(13.0555891306266,6.56423170131094,3.21026703780761));
#33511=CARTESIAN_POINT('Ctrl Pts',(13.0302753666322,6.55969855998359,3.29845393225428));
#33512=CARTESIAN_POINT('Ctrl Pts',(13.0045795814911,6.55511858261199,3.38434033500869));
#33513=CARTESIAN_POINT('Ctrl Pts',(12.99200037201,6.55287648358838,3.42638548155284));
#33514=CARTESIAN_POINT('Ctrl Pts',(12.9793303739806,6.5506231601651,3.46787961563997));
#33515=CARTESIAN_POINT('Ctrl Pts',(12.9666085639724,6.54836510018653,3.50875595858229));
#33516=CARTESIAN_POINT('Ctrl Pts',(12.940792431796,6.5437828611159,3.5917055602194));
#33517=CARTESIAN_POINT('Ctrl Pts',(12.9147681836767,6.53918111699148,3.67211234175013));
#33518=CARTESIAN_POINT('Ctrl Pts',(12.8885057287866,6.53455169676247,3.75050983225192));
#33519=CARTESIAN_POINT('Ctrl Pts',(12.8615210754612,6.52979497083945,3.83106319680337));
#33520=CARTESIAN_POINT('Ctrl Pts',(12.8342847721211,6.52500902573734,3.90949538777508));
#33521=CARTESIAN_POINT('Ctrl Pts',(12.8067104903906,6.52018499760443,3.98637282662223));
#33522=CARTESIAN_POINT('Ctrl Pts',(12.7945330216198,6.51805459027371,4.02032376031806));
#33523=CARTESIAN_POINT('Ctrl Pts',(12.7822889612338,6.51591675553747,4.05397129591668));
#33524=CARTESIAN_POINT('Ctrl Pts',(12.7699677834507,6.51377072994513,4.08736337382604));
#33525=CARTESIAN_POINT('Ctrl Pts',(12.7427108058986,6.50902328027543,4.16123351303019));
#33526=CARTESIAN_POINT('Ctrl Pts',(12.7150811577462,6.50423574575775,4.23385109131939));
#33527=CARTESIAN_POINT('Ctrl Pts',(12.6868914513244,6.49937095059352,4.30582894702377));
#33528=CARTESIAN_POINT('Ctrl Pts',(12.6585644801614,6.494482467178,4.37815728604268));
#33529=CARTESIAN_POINT('Ctrl Pts',(12.6296718796146,6.48951596887022,4.44983980209247));
#33530=CARTESIAN_POINT('Ctrl Pts',(12.5999743835185,6.48443373416024,4.52148008523258));
#33531=CARTESIAN_POINT('Ctrl Pts',(12.5861748224671,6.48207216778673,4.5547692372113));
#33532=CARTESIAN_POINT('Ctrl Pts',(12.5722007878739,6.47968561172406,4.58804900037526));
#33533=CARTESIAN_POINT('Ctrl Pts',(12.5580247409487,6.47727028132517,4.62137845204915));
#33534=CARTESIAN_POINT('Ctrl Pts',(12.5168376484799,6.47025277940755,4.71821385441987));
#33535=CARTESIAN_POINT('Ctrl Pts',(12.4739402348053,6.46299238320348,4.81546529168791));
#33536=CARTESIAN_POINT('Ctrl Pts',(12.4294801907888,6.45552630928657,4.91263509352366));
#33537=CARTESIAN_POINT('Ctrl Pts',(12.3929332080852,6.44938905773091,4.9925104770408));
#33538=CARTESIAN_POINT('Ctrl Pts',(12.355331219531,6.44311282674947,5.07233092004027));
#33539=CARTESIAN_POINT('Ctrl Pts',(12.3167808262493,6.43671828828554,5.15182971976806));
#33540=CARTESIAN_POINT('Ctrl Pts',(12.2651233822605,6.42814962051294,5.25835794022213));
#33541=CARTESIAN_POINT('Ctrl Pts',(12.211761199467,6.41936852050751,5.36431060995521));
#33542=CARTESIAN_POINT('Ctrl Pts',(12.1569061803181,6.41042804776098,5.46926381567329));
#33543=CARTESIAN_POINT('Ctrl Pts',(12.1210244044939,6.40457990398431,5.53791582706711));
#33544=CARTESIAN_POINT('Ctrl Pts',(12.0845048538408,6.3986635688782,5.606140646506));
#33545=CARTESIAN_POINT('Ctrl Pts',(12.0474174600384,6.3926938927608,5.67382535260096));
#33546=CARTESIAN_POINT('Ctrl Pts',(11.9926822297006,6.3838835784241,5.77371746144518));
#33547=CARTESIAN_POINT('Ctrl Pts',(11.9367157922521,6.37495708110681,5.8724355292054));
#33548=CARTESIAN_POINT('Ctrl Pts',(11.8793286684131,6.36589527473159,5.97035005230608));
#33549=CARTESIAN_POINT('Ctrl Pts',(11.8383864053749,6.35943022063242,6.04020617841705));
#33550=CARTESIAN_POINT('Ctrl Pts',(11.796720037908,6.35289629470045,6.10965282806653));
#33551=CARTESIAN_POINT('Ctrl Pts',(11.7542467422086,6.34628655152287,6.17881640065429));
#33552=CARTESIAN_POINT('Ctrl Pts',(11.6787939476812,6.33454450076735,6.30168383406892));
#33553=CARTESIAN_POINT('Ctrl Pts',(11.6007955847598,6.32256318084416,6.42365766571776));
#33554=CARTESIAN_POINT('Ctrl Pts',(11.5200360405655,6.31034401507871,6.54492039630344));
#33555=CARTESIAN_POINT('Ctrl Pts',(11.4916148586905,6.30604380343135,6.58759560150689));
#33556=CARTESIAN_POINT('Ctrl Pts',(11.462851342409,6.3017141345399,6.63018243833174));
#33557=CARTESIAN_POINT('Ctrl Pts',(11.4337349306691,6.29735507044112,6.67268784821382));
#33558=CARTESIAN_POINT('Ctrl Pts',(11.3778091956261,6.28898234010605,6.75433067948669));
#33559=CARTESIAN_POINT('Ctrl Pts',(11.3205862334272,6.28050116110226,6.8356750631076));
#33560=CARTESIAN_POINT('Ctrl Pts',(11.2616761282475,6.27186760351598,6.91716968355268));
#33561=CARTESIAN_POINT('Ctrl Pts',(11.2063472398295,6.26375889036932,6.99371014715426));
#33562=CARTESIAN_POINT('Ctrl Pts',(11.1495296754629,6.25551576207198,7.07038306740363));
#33563=CARTESIAN_POINT('Ctrl Pts',(11.0908602382651,6.24710182319922,7.14752688198067));
#33564=CARTESIAN_POINT('Ctrl Pts',(11.0870628011956,6.24655722272405,7.15252009130992));
#33565=CARTESIAN_POINT('Ctrl Pts',(11.0832575922087,6.24601190664599,7.15751526131866));
#33566=CARTESIAN_POINT('Ctrl Pts',(11.0794445071668,6.24546586509583,7.16251247866907));
#33567=CARTESIAN_POINT('Ctrl Pts',(11.0167202277328,6.23648362043076,7.24471543350426));
#33568=CARTESIAN_POINT('Ctrl Pts',(10.9518690113909,6.22730506726939,7.32747369271627));
#33569=CARTESIAN_POINT('Ctrl Pts',(10.8845241565944,6.21790432002736,7.41100156356173));
#33570=CARTESIAN_POINT('Ctrl Pts',(10.8171793017979,6.20850357278533,7.49452943440719));
#33571=CARTESIAN_POINT('Ctrl Pts',(10.7473408580157,6.19888063146263,7.57882731379565));
#33572=CARTESIAN_POINT('Ctrl Pts',(10.6746067396372,6.18900961047489,7.66406851881595));
#33573=CARTESIAN_POINT('Ctrl Pts',(10.6092476574337,6.18013948340723,7.74066650405669));
#33574=CARTESIAN_POINT('Ctrl Pts',(10.5415523622487,6.17106903523843,7.81802449638722));
#33575=CARTESIAN_POINT('Ctrl Pts',(10.4711322854565,6.1617777234388,7.8963118222002));
#33576=CARTESIAN_POINT('Ctrl Pts',(10.4026106648622,6.15273689629178,7.97248859849848));
#33577=CARTESIAN_POINT('Ctrl Pts',(10.3315091069494,6.14348695352644,8.04954548082737));
#33578=CARTESIAN_POINT('Ctrl Pts',(10.2574401066208,6.13400896964473,8.12759869082826));
#33579=CARTESIAN_POINT('Ctrl Pts',(10.2382091260077,6.13154814361128,8.14786411579227));
#33580=CARTESIAN_POINT('Ctrl Pts',(10.2187779530672,6.12907194512913,8.16819648124987));
#33581=CARTESIAN_POINT('Ctrl Pts',(10.199139479305,6.12658004295878,8.18859733758286));
#33582=CARTESIAN_POINT('Ctrl Pts',(10.0955471544311,6.11343533821694,8.29621120628442));
#33583=CARTESIAN_POINT('Ctrl Pts',(9.98618552590945,6.09985367380175,8.40572955822586));
#33584=CARTESIAN_POINT('Ctrl Pts',(9.87093205162319,6.0859343295064,8.51640709901712));
#33585=CARTESIAN_POINT('Ctrl Pts',(9.79369900175001,6.07660677197443,8.59057374848871));
#33586=CARTESIAN_POINT('Ctrl Pts',(9.71382101063564,6.06712757802916,8.66526037192818));
#33587=CARTESIAN_POINT('Ctrl Pts',(9.63127322650993,6.0575266227,8.74023722148102));
#33588=CARTESIAN_POINT('',(9.631273226509,6.0575266227,8.74023722148));
#33589=CARTESIAN_POINT('',(13.3,5.241201401137,2.164009824691));
#33590=CARTESIAN_POINT('',(13.3,5.241201401137,-2.164009824691));
#33591=CARTESIAN_POINT('Ctrl Pts',(13.300000000001,5.24120140113708,2.16400982469131));
#33592=CARTESIAN_POINT('Ctrl Pts',(13.3180935597627,5.38692580429823,2.06695933461524));
#33593=CARTESIAN_POINT('Ctrl Pts',(13.3374024258682,5.52055417312555,1.95640108904449));
#33594=CARTESIAN_POINT('Ctrl Pts',(13.3922809876029,5.86870480663107,1.60825045553898));
#33595=CARTESIAN_POINT('Ctrl Pts',(13.4307628143448,6.06863168929127,1.3166037527462));
#33596=CARTESIAN_POINT('Ctrl Pts',(13.4849916924495,6.33430849895895,0.676325134116298));
#33597=CARTESIAN_POINT('Ctrl Pts',(13.500000000001,6.4,0.327606623932291));
#33598=CARTESIAN_POINT('Ctrl Pts',(13.500000000001,6.4,-0.327606623932292));
#33599=CARTESIAN_POINT('Ctrl Pts',(13.4849916924495,6.33430849895895,-0.676325134116299));
#33600=CARTESIAN_POINT('Ctrl Pts',(13.4307628143448,6.06863168929127,-1.31660375274621));
#33601=CARTESIAN_POINT('Ctrl Pts',(13.3922809876029,5.86870480663107,-1.60825045553898));
#33602=CARTESIAN_POINT('Ctrl Pts',(13.3374024258682,5.52055417312555,-1.95640108904449));
#33603=CARTESIAN_POINT('Ctrl Pts',(13.3180935597627,5.38692580429823,-2.06695933461524));
#33604=CARTESIAN_POINT('Ctrl Pts',(13.300000000001,5.24120140113708,-2.16400982469131));
#33605=CARTESIAN_POINT('',(13.3,2.358798598863,-2.164009824691));
#33606=CARTESIAN_POINT('Ctrl Pts',(13.3000000000008,5.24120140113749,-2.16400982469205));
#33607=CARTESIAN_POINT('Ctrl Pts',(13.2864350300733,5.10747808862643,-2.23676980098582));
#33608=CARTESIAN_POINT('Ctrl Pts',(13.2739820406732,4.96621350744257,-2.29979178340204));
#33609=CARTESIAN_POINT('Ctrl Pts',(13.2394248960124,4.48771447089005,-2.46983579880371));
#33610=CARTESIAN_POINT('Ctrl Pts',(13.2265218318602,4.13149059985939,-2.52652183186019));
#33611=CARTESIAN_POINT('Ctrl Pts',(13.2265218318602,3.46850940014061,-2.52652183186019));
#33612=CARTESIAN_POINT('Ctrl Pts',(13.2394248960124,3.11228552910995,-2.46983579880371));
#33613=CARTESIAN_POINT('Ctrl Pts',(13.2739820406732,2.63378649255743,-2.29979178340204));
#33614=CARTESIAN_POINT('Ctrl Pts',(13.2864350300733,2.49252191137357,-2.23676980098582));
#33615=CARTESIAN_POINT('Ctrl Pts',(13.3000000000008,2.35879859886251,-2.16400982469205));
#33616=CARTESIAN_POINT('',(13.3,2.358798598863,2.164009824691));
#33617=CARTESIAN_POINT('Ctrl Pts',(13.300000000001,2.35879859886292,-2.16400982469131));
#33618=CARTESIAN_POINT('Ctrl Pts',(13.3180935597627,2.21307419570177,-2.06695933461524));
#33619=CARTESIAN_POINT('Ctrl Pts',(13.3374024258682,2.07944582687445,-1.95640108904449));
#33620=CARTESIAN_POINT('Ctrl Pts',(13.3922809876029,1.73129519336893,-1.60825045553898));
#33621=CARTESIAN_POINT('Ctrl Pts',(13.4307628143448,1.53136831070873,-1.3166037527462));
#33622=CARTESIAN_POINT('Ctrl Pts',(13.4849916924495,1.26569150104105,-0.676325134116298));
#33623=CARTESIAN_POINT('Ctrl Pts',(13.500000000001,1.2,-0.327606623932291));
#33624=CARTESIAN_POINT('Ctrl Pts',(13.500000000001,1.2,0.327606623932291));
#33625=CARTESIAN_POINT('Ctrl Pts',(13.4849916924495,1.26569150104105,0.676325134116298));
#33626=CARTESIAN_POINT('Ctrl Pts',(13.4307628143448,1.53136831070873,1.3166037527462));
#33627=CARTESIAN_POINT('Ctrl Pts',(13.3922809876029,1.73129519336893,1.60825045553898));
#33628=CARTESIAN_POINT('Ctrl Pts',(13.3374024258682,2.07944582687445,1.95640108904449));
#33629=CARTESIAN_POINT('Ctrl Pts',(13.3180935597627,2.21307419570177,2.06695933461524));
#33630=CARTESIAN_POINT('Ctrl Pts',(13.300000000001,2.35879859886292,2.16400982469131));
#33631=CARTESIAN_POINT('Ctrl Pts',(13.3000000000008,2.35879859886251,2.16400982469205));
#33632=CARTESIAN_POINT('Ctrl Pts',(13.2864350300733,2.49252191137357,2.23676980098582));
#33633=CARTESIAN_POINT('Ctrl Pts',(13.2739820406732,2.63378649255743,2.29979178340204));
#33634=CARTESIAN_POINT('Ctrl Pts',(13.2394248960124,3.11228552910995,2.46983579880371));
#33635=CARTESIAN_POINT('Ctrl Pts',(13.2265218318602,3.46850940014061,2.52652183186019));
#33636=CARTESIAN_POINT('Ctrl Pts',(13.2265218318602,3.8,2.52652183186019));
#33637=CARTESIAN_POINT('Ctrl Pts',(13.2265218318602,4.13149059985939,2.52652183186019));
#33638=CARTESIAN_POINT('Ctrl Pts',(13.2394248960124,4.48771447089005,2.46983579880371));
#33639=CARTESIAN_POINT('Ctrl Pts',(13.2739820406732,4.96621350744257,2.29979178340204));
#33640=CARTESIAN_POINT('Ctrl Pts',(13.2864350300733,5.10747808862643,2.23676980098582));
#33641=CARTESIAN_POINT('Ctrl Pts',(13.3000000000008,5.24120140113749,2.16400982469205));
#33642=CARTESIAN_POINT('Origin',(13.875,3.8,0.));
#33643=CARTESIAN_POINT('',(13.3000000000008,6.40000000000084,3.18408167778415E-16));
#33644=CARTESIAN_POINT('Origin',(13.3,3.8,0.));
#33645=CARTESIAN_POINT('Origin',(13.3,3.8,0.));
#33646=CARTESIAN_POINT('Origin',(13.875,3.8,0.));
#33647=CARTESIAN_POINT('Origin',(13.3,3.8,0.));
#33648=CARTESIAN_POINT('Origin',(12.625,3.8,0.));
#33649=CARTESIAN_POINT('',(11.95,2.55,0.));
#33650=CARTESIAN_POINT('',(11.95,5.05,1.53080849893419E-16));
#33651=CARTESIAN_POINT('Origin',(11.95,3.8,0.));
#33652=CARTESIAN_POINT('',(12.625,5.725,2.35744508835865E-16));
#33653=CARTESIAN_POINT('Origin',(11.95,3.8,0.));
#33654=CARTESIAN_POINT('Origin',(13.875,3.8,0.));
#33655=CARTESIAN_POINT('',(6.,2.55,0.));
#33656=CARTESIAN_POINT('',(13.875,2.55,1.53080849893419E-16));
#33657=CARTESIAN_POINT('Origin',(6.,3.8,0.));
#33658=CARTESIAN_POINT('Origin',(6.,0.,0.));
#33659=CARTESIAN_POINT('',(6.,3.8,-2.5));
#33660=CARTESIAN_POINT('Origin',(6.,3.8,0.));
#33661=CARTESIAN_POINT('Origin',(-1.,3.8,0.));
#33662=CARTESIAN_POINT('',(-1.,3.8,-2.5));
#33663=CARTESIAN_POINT('',(-1.,3.8,-2.5));
#33664=CARTESIAN_POINT('Origin',(-1.,3.8,0.));
#33665=CARTESIAN_POINT('Origin',(-1.,0.,0.));
#33666=CARTESIAN_POINT('Ctrl Pts',(9.485442650021,5.952891693689,-8.860081849749));
#33667=CARTESIAN_POINT('Ctrl Pts',(9.534636054532,5.959034860707,-8.816948875496));
#33668=CARTESIAN_POINT('Ctrl Pts',(9.870556912557,6.001493104786,-8.517415431551));
#33669=CARTESIAN_POINT('Ctrl Pts',(10.43177183646,6.078357198741,-7.956077122609));
#33670=CARTESIAN_POINT('Ctrl Pts',(11.09306532507,6.178684101018,-7.159219782959));
#33671=CARTESIAN_POINT('Ctrl Pts',(11.62422729818,6.265537517347,-6.399074799972));
#33672=CARTESIAN_POINT('Ctrl Pts',(12.04988106646,6.339153757363,-5.681632943686));
#33673=CARTESIAN_POINT('Ctrl Pts',(12.39479790134,6.401396123129,-5.00006532987));
#33674=CARTESIAN_POINT('Ctrl Pts',(12.68337078438,6.455239570641,-4.329650458296));
#33675=CARTESIAN_POINT('Ctrl Pts',(12.92973905293,6.502503926928,-3.644849379563));
#33676=CARTESIAN_POINT('Ctrl Pts',(13.13522025712,6.54285063425,-2.938234819852));
#33677=CARTESIAN_POINT('Ctrl Pts',(13.29643076178,6.575090237291,-2.218196523314));
#33678=CARTESIAN_POINT('Ctrl Pts',(13.41211690496,6.598540633102,-1.491642412231));
#33679=CARTESIAN_POINT('Ctrl Pts',(13.48237446627,6.612910993203,-0.7590144441822));
#33680=CARTESIAN_POINT('Ctrl Pts',(13.50678376795,6.61792644257,-0.02280129264716));
#33681=CARTESIAN_POINT('Ctrl Pts',(13.48527073568,6.613505521845,0.7109530505647));
#33682=CARTESIAN_POINT('Ctrl Pts',(13.41877759765,6.599899443318,1.436789723415));
#33683=CARTESIAN_POINT('Ctrl Pts',(13.30878668262,6.57758461397,2.150825299771));
#33684=CARTESIAN_POINT('Ctrl Pts',(13.15883216383,6.547550459594,2.841355547203));
#33685=CARTESIAN_POINT('Ctrl Pts',(12.97830256373,6.511998053041,3.485919540467));
#33686=CARTESIAN_POINT('Ctrl Pts',(12.77805158862,6.4733296184,4.07466488761));
#33687=CARTESIAN_POINT('Ctrl Pts',(12.56058971477,6.432225904256,4.62210341788));
#33688=CARTESIAN_POINT('Ctrl Pts',(12.31982924549,6.387800142595,5.150989661439));
#33689=CARTESIAN_POINT('Ctrl Pts',(12.05172287785,6.33968980881,5.670016802825));
#33690=CARTESIAN_POINT('Ctrl Pts',(11.75719282679,6.28849176907,6.176788355475));
#33691=CARTESIAN_POINT('Ctrl Pts',(11.43474145404,6.234418256753,6.673056312275));
#33692=CARTESIAN_POINT('Ctrl Pts',(11.07576023228,6.176643934304,7.168730439045));
#33693=CARTESIAN_POINT('Ctrl Pts',(10.66606024847,6.113822407882,7.675609305722));
#33694=CARTESIAN_POINT('Ctrl Pts',(10.1860426261,6.04445748388,8.20437686418));
#33695=CARTESIAN_POINT('Ctrl Pts',(9.780289236406,5.990083979416,8.597903917999));
#33696=CARTESIAN_POINT('Ctrl Pts',(9.534645032455,5.959035996825,8.816940677232));
#33697=CARTESIAN_POINT('Ctrl Pts',(9.485454696088,5.952893121937,8.860071898555));
#33698=CARTESIAN_POINT('Ctrl Pts',(9.501283522908,6.25924448941,-8.919478697923));
#33699=CARTESIAN_POINT('Ctrl Pts',(9.550507806299,6.265441721484,-8.876058641547));
#33700=CARTESIAN_POINT('Ctrl Pts',(9.886639439875,6.308272767042,-8.574531191516));
#33701=CARTESIAN_POINT('Ctrl Pts',(10.44820557707,6.385801787616,-8.009451327147));
#33702=CARTESIAN_POINT('Ctrl Pts',(11.10991201118,6.486981590413,-7.207272704089));
#33703=CARTESIAN_POINT('Ctrl Pts',(11.64140552514,6.574564764989,-6.442044024142));
#33704=CARTESIAN_POINT('Ctrl Pts',(12.06732516279,6.648794492034,-5.719798235741));
#33705=CARTESIAN_POINT('Ctrl Pts',(12.41245772277,6.711552517154,-5.033662382996));
#33706=CARTESIAN_POINT('Ctrl Pts',(12.70121138752,6.76584007241,-4.358750315406));
#33707=CARTESIAN_POINT('Ctrl Pts',(12.94773428354,6.813492891526,-3.669352220712));
#33708=CARTESIAN_POINT('Ctrl Pts',(13.15334470394,6.854170257082,-2.957991205558));
#33709=CARTESIAN_POINT('Ctrl Pts',(13.31465676988,6.88667349715,-2.233113750652));
#33710=CARTESIAN_POINT('Ctrl Pts',(13.43041590509,6.910315353154,-1.50167473912));
#33711=CARTESIAN_POINT('Ctrl Pts',(13.50071784403,6.924802918115,-0.7641196938934));
#33712=CARTESIAN_POINT('Ctrl Pts',(13.52514257268,6.929859252279,-0.02295466127787));
#33713=CARTESIAN_POINT('Ctrl Pts',(13.50361594369,6.925402293752,0.7157350447915));
#33714=CARTESIAN_POINT('Ctrl Pts',(13.43708080358,6.911685249168,1.446453187537));
#33715=CARTESIAN_POINT('Ctrl Pts',(13.32702048293,6.889188248829,2.165289624432));
#33716=CARTESIAN_POINT('Ctrl Pts',(13.17697147856,6.858908536401,2.860460929475));
#33717=CARTESIAN_POINT('Ctrl Pts',(12.99632832114,6.823064867231,3.50935495712));
#33718=CARTESIAN_POINT('Ctrl Pts',(12.79595159765,6.784078877253,4.10205323945));
#33719=CARTESIAN_POINT('Ctrl Pts',(12.57835337903,6.742636698209,4.653165293559));
#33720=CARTESIAN_POINT('Ctrl Pts',(12.33744216991,6.697843973672,5.185598399135));
#33721=CARTESIAN_POINT('Ctrl Pts',(12.06916814928,6.649334755299,5.708103930231));
#33722=CARTESIAN_POINT('Ctrl Pts',(11.77445409949,6.597710356767,6.218269250769));
#33723=CARTESIAN_POINT('Ctrl Pts',(11.45180140757,6.543184206245,6.717858020621));
#33724=CARTESIAN_POINT('Ctrl Pts',(11.09259610083,6.484923277324,7.216846154425));
#33725=CARTESIAN_POINT('Ctrl Pts',(10.68264028709,6.421568601756,7.727110711857));
#33726=CARTESIAN_POINT('Ctrl Pts',(10.20232262365,6.351609196432,8.259406264638));
#33727=CARTESIAN_POINT('Ctrl Pts',(9.796315124191,6.296763464549,8.655555492532));
#33728=CARTESIAN_POINT('Ctrl Pts',(9.550516790186,6.265442867547,8.876050388876));
#33729=CARTESIAN_POINT('Ctrl Pts',(9.501295577027,6.259245930234,8.91946868085));
#33730=CARTESIAN_POINT('Ctrl Pts',(9.35997989658,6.507098481045,-8.792071395616));
#33731=CARTESIAN_POINT('Ctrl Pts',(9.408273439289,6.513077227545,-8.749258512838));
#33732=CARTESIAN_POINT('Ctrl Pts',(9.738051948008,6.554400160203,-8.451947043545));
#33733=CARTESIAN_POINT('Ctrl Pts',(10.28903193377,6.629221549912,-7.894765291821));
#33734=CARTESIAN_POINT('Ctrl Pts',(10.93829150539,6.726898620283,-7.10382265491));
#33735=CARTESIAN_POINT('Ctrl Pts',(11.45979182787,6.811464936495,-6.3493547208));
#33736=CARTESIAN_POINT('Ctrl Pts',(11.87769772134,6.883144779298,-5.637314350587));
#33737=CARTESIAN_POINT('Ctrl Pts',(12.21632796884,6.943749925877,-4.960922641443));
#33738=CARTESIAN_POINT('Ctrl Pts',(12.4996325731,6.9961762299,-4.295642816956));
#33739=CARTESIAN_POINT('Ctrl Pts',(12.74149474047,7.042195399749,-3.616131678469));
#33740=CARTESIAN_POINT('Ctrl Pts',(12.94321036984,7.08147790737,-2.915020481202));
#33741=CARTESIAN_POINT('Ctrl Pts',(13.10146121022,7.112866122033,-2.200631020283));
#33742=CARTESIAN_POINT('Ctrl Pts',(13.21502024463,7.135696584537,-1.479810217005));
#33743=CARTESIAN_POINT('Ctrl Pts',(13.28398456809,7.149686753743,-0.7529872864468));
#33744=CARTESIAN_POINT('Ctrl Pts',(13.30794430238,7.15456945535,-0.02262016733114));
#33745=CARTESIAN_POINT('Ctrl Pts',(13.28682750111,7.150265547977,0.7053073001723));
#33746=CARTESIAN_POINT('Ctrl Pts',(13.22155837359,7.137019453742,1.425391562183));
#33747=CARTESIAN_POINT('Ctrl Pts',(13.1135900535,7.115294579917,2.133790387283));
#33748=CARTESIAN_POINT('Ctrl Pts',(12.96638900092,7.086053660963,2.818899704123));
#33749=CARTESIAN_POINT('Ctrl Pts',(12.78916864978,7.051439169748,3.458437528109));
#33750=CARTESIAN_POINT('Ctrl Pts',(12.59258219107,7.013789778161,4.042624198806));
#33751=CARTESIAN_POINT('Ctrl Pts',(12.37909362994,6.973768350244,4.585852924676));
#33752=CARTESIAN_POINT('Ctrl Pts',(12.1427259698,6.930511582039,5.110699731971));
#33753=CARTESIAN_POINT('Ctrl Pts',(11.87950528854,6.883666724966,5.625789474164));
#33754=CARTESIAN_POINT('Ctrl Pts',(11.59033726588,6.833815414448,6.128740954401));
#33755=CARTESIAN_POINT('Ctrl Pts',(11.2737526677,6.781165017737,6.621289226868));
#33756=CARTESIAN_POINT('Ctrl Pts',(10.92130165418,6.724912967278,7.113266081009));
#33757=CARTESIAN_POINT('Ctrl Pts',(10.51905697905,6.663749998167,7.616378545751));
#33758=CARTESIAN_POINT('Ctrl Pts',(10.04778305149,6.596222248822,8.141226799633));
#33759=CARTESIAN_POINT('Ctrl Pts',(9.649434841825,6.543296109889,8.531838461027));
#33760=CARTESIAN_POINT('Ctrl Pts',(9.408282243416,6.513078333271,8.749250370185));
#33761=CARTESIAN_POINT('Ctrl Pts',(9.359991707996,6.507099872998,8.792061517141));
#33762=CARTESIAN_POINT('Ctrl Pts',(9.152731006141,6.53648541412,-8.560090306046));
#33763=CARTESIAN_POINT('Ctrl Pts',(9.199732900989,6.542114137906,-8.518386974692));
#33764=CARTESIAN_POINT('Ctrl Pts',(9.520694775513,6.581021399357,-8.228780423059));
#33765=CARTESIAN_POINT('Ctrl Pts',(10.05698368769,6.651510141599,-7.686038905367));
#33766=CARTESIAN_POINT('Ctrl Pts',(10.68896995904,6.743589556577,-6.915637669631));
#33767=CARTESIAN_POINT('Ctrl Pts',(11.19660209605,6.823339518226,-6.180829796028));
#33768=CARTESIAN_POINT('Ctrl Pts',(11.60338680859,6.890951834637,-5.487417482014));
#33769=CARTESIAN_POINT('Ctrl Pts',(11.93299338477,6.948125061152,-4.828793299445));
#33770=CARTESIAN_POINT('Ctrl Pts',(12.2087359823,6.997586031203,-4.18105837969));
#33771=CARTESIAN_POINT('Ctrl Pts',(12.44413016099,7.0410038186,-3.519536996875));
#33772=CARTESIAN_POINT('Ctrl Pts',(12.64044074188,7.078066211933,-2.837056522375));
#33773=CARTESIAN_POINT('Ctrl Pts',(12.79444332545,7.107680390949,-2.141713117333));
#33774=CARTESIAN_POINT('Ctrl Pts',(12.9049491405,7.129220290391,-1.440160498536));
#33775=CARTESIAN_POINT('Ctrl Pts',(12.97205717013,7.142419489043,-0.7328022253019));
#33776=CARTESIAN_POINT('Ctrl Pts',(12.99537160226,7.147026105496,-0.0220136976379));
#33777=CARTESIAN_POINT('Ctrl Pts',(12.97482354493,7.142965556986,0.686400021429));
#33778=CARTESIAN_POINT('Ctrl Pts',(12.91131134333,7.130468371904,1.38719829978));
#33779=CARTESIAN_POINT('Ctrl Pts',(12.80624622508,7.109971581401,2.076657613881));
#33780=CARTESIAN_POINT('Ctrl Pts',(12.66299745577,7.08238335636,2.743496037382));
#33781=CARTESIAN_POINT('Ctrl Pts',(12.49052714993,7.049725155911,3.366030037639));
#33782=CARTESIAN_POINT('Ctrl Pts',(12.299200682,7.01420385811,3.934734056953));
#33783=CARTESIAN_POINT('Ctrl Pts',(12.09141535314,6.97644542572,4.463610607139));
#33784=CARTESIAN_POINT('Ctrl Pts',(11.861353064,6.935636206461,4.974634253413));
#33785=CARTESIAN_POINT('Ctrl Pts',(11.60514522221,6.891444755714,5.476200276634));
#33786=CARTESIAN_POINT('Ctrl Pts',(11.32367377305,6.844421605485,5.965986216616));
#33787=CARTESIAN_POINT('Ctrl Pts',(11.0155102533,6.794764718208,6.445676711681));
#33788=CARTESIAN_POINT('Ctrl Pts',(10.67243260075,6.741720474333,6.924842172373));
#33789=CARTESIAN_POINT('Ctrl Pts',(10.28088916162,6.684059510856,7.414880816488));
#33790=CARTESIAN_POINT('Ctrl Pts',(9.822165799765,6.620420131763,7.926113063764));
#33791=CARTESIAN_POINT('Ctrl Pts',(9.434446872203,6.570566475392,8.306601436968));
#33792=CARTESIAN_POINT('Ctrl Pts',(9.199741455652,6.542115179046,8.518379035476));
#33793=CARTESIAN_POINT('Ctrl Pts',(9.15274248074,6.536486727296,8.560080681194));
#33794=CARTESIAN_POINT('Origin',(9.295100305717,6.057526619323,8.370118635987));
#33795=CARTESIAN_POINT('Ctrl Pts',(9.653942535497,6.031033711932,8.717909060576));
#33796=CARTESIAN_POINT('Ctrl Pts',(9.646944916628,6.030093928364,8.724648332143));
#33797=CARTESIAN_POINT('Ctrl Pts',(9.59719467314,6.023650265556,8.771170219865));
#33798=CARTESIAN_POINT('Ctrl Pts',(9.495042840547,6.013489241721,8.848779982819));
#33799=CARTESIAN_POINT('Ctrl Pts',(9.33375118979,6.004441014892,8.931245876486));
#33800=CARTESIAN_POINT('Ctrl Pts',(9.152585363009,6.001089741996,8.98551789411));
#33801=CARTESIAN_POINT('Ctrl Pts',(9.013899860845,6.003522469926,8.999282418285));
#33802=CARTESIAN_POINT('Ctrl Pts',(8.937785978944,6.00642658824,8.998158241186));
#33803=CARTESIAN_POINT('Ctrl Pts',(8.927957310455,6.006827995205,8.997866981941));
#33804=CARTESIAN_POINT('Ctrl Pts',(9.645773860495,6.31475659886,8.747934865266));
#33805=CARTESIAN_POINT('Ctrl Pts',(9.638958592229,6.313838584937,8.754518086709));
#33806=CARTESIAN_POINT('Ctrl Pts',(9.590505220355,6.307544168074,8.799962308943));
#33807=CARTESIAN_POINT('Ctrl Pts',(9.491021810395,6.297618091538,8.875768956116));
#33808=CARTESIAN_POINT('Ctrl Pts',(9.333955851884,6.288775548995,8.956311007241));
#33809=CARTESIAN_POINT('Ctrl Pts',(9.157544689065,6.285492132199,9.009313113419));
#33810=CARTESIAN_POINT('Ctrl Pts',(9.022499207939,6.287856157087,9.02275401755));
#33811=CARTESIAN_POINT('Ctrl Pts',(8.948380877393,6.290684710128,9.021654827436));
#33812=CARTESIAN_POINT('Ctrl Pts',(8.938809854365,6.291075723373,9.021370205509));
#33813=CARTESIAN_POINT('Ctrl Pts',(9.501656951024,6.529655143128,8.627454091879));
#33814=CARTESIAN_POINT('Ctrl Pts',(9.496360020516,6.528944036884,8.63258932645));
#33815=CARTESIAN_POINT('Ctrl Pts',(9.458705017816,6.524069354645,8.668034829828));
#33816=CARTESIAN_POINT('Ctrl Pts',(9.38144016242,6.516395155231,8.727123383244));
#33817=CARTESIAN_POINT('Ctrl Pts',(9.259559325096,6.509578980089,8.789847902424));
#33818=CARTESIAN_POINT('Ctrl Pts',(9.12273775328,6.507065811343,8.831104321855));
#33819=CARTESIAN_POINT('Ctrl Pts',(9.018000816625,6.508907798825,8.841565722931));
#33820=CARTESIAN_POINT('Ctrl Pts',(8.96049839471,6.511101044754,8.840709421231));
#33821=CARTESIAN_POINT('Ctrl Pts',(8.953072650201,6.511404160057,8.840487781273));
#33822=CARTESIAN_POINT('Ctrl Pts',(9.302738926203,6.554727598069,8.424305189807));
#33823=CARTESIAN_POINT('Ctrl Pts',(9.299441398479,6.554292035165,8.427515810797));
#33824=CARTESIAN_POINT('Ctrl Pts',(9.276006083907,6.551308174027,8.449671465829));
#33825=CARTESIAN_POINT('Ctrl Pts',(9.227999435144,6.546634829437,8.486540313026));
#33826=CARTESIAN_POINT('Ctrl Pts',(9.152451654413,6.542524729215,8.525586031012));
#33827=CARTESIAN_POINT('Ctrl Pts',(9.067763106405,6.541050501118,8.55123456792));
#33828=CARTESIAN_POINT('Ctrl Pts',(9.002937571468,6.542211057571,8.557738235401));
#33829=CARTESIAN_POINT('Ctrl Pts',(8.967315586768,6.543566973447,8.557205961694));
#33830=CARTESIAN_POINT('Ctrl Pts',(8.962714823604,6.5437541788,8.557068185445));
#33831=CARTESIAN_POINT('Ctrl Pts',(9.63127320806298,6.05752662158217,8.74023723823402));
#33832=CARTESIAN_POINT('Ctrl Pts',(9.59861968550863,6.05554784605247,8.76989447988101));
#33833=CARTESIAN_POINT('Ctrl Pts',(9.56377963052759,6.05376690177339,8.79757308911125));
#33834=CARTESIAN_POINT('Ctrl Pts',(9.52714118362392,6.05221803617318,8.8228771921826));
#33835=CARTESIAN_POINT('Ctrl Pts',(9.51544884961683,6.05172375064909,8.8309524259838));
#33836=CARTESIAN_POINT('Ctrl Pts',(9.50357367483786,6.05125305271542,8.83878608429263));
#33837=CARTESIAN_POINT('Ctrl Pts',(9.49152905935388,6.05080691142483,8.84636606478418));
#33838=CARTESIAN_POINT('Ctrl Pts',(9.46663316979638,6.04988474962462,8.86203367637514));
#33839=CARTESIAN_POINT('Ctrl Pts',(9.44101708626723,6.04907020633919,8.87662025026625));
#33840=CARTESIAN_POINT('Ctrl Pts',(9.41465075551265,6.04836152478895,8.89011896197565));
#33841=CARTESIAN_POINT('Ctrl Pts',(9.38828952944122,6.0476529804438,8.90361506025176));
#33842=CARTESIAN_POINT('Ctrl Pts',(9.36117771796724,6.04705018167203,8.91602418308567));
#33843=CARTESIAN_POINT('Ctrl Pts',(9.3332677890998,6.04656067319867,8.9272913800025));
#33844=CARTESIAN_POINT('Ctrl Pts',(9.30535515794258,6.04607111733021,8.9385596678297));
#33845=CARTESIAN_POINT('Ctrl Pts',(9.27665152939504,6.04569542348672,8.94868311708087));
#33846=CARTESIAN_POINT('Ctrl Pts',(9.24710436032083,6.04544064223698,8.95757570678599));
#33847=CARTESIAN_POINT('Ctrl Pts',(9.21968152314074,6.04520417881436,8.96582895226545));
#33848=CARTESIAN_POINT('Ctrl Pts',(9.19153146044287,6.04507191208051,8.97302179223174));
#33849=CARTESIAN_POINT('Ctrl Pts',(9.16261456287849,6.0450584487924,8.97903646990965));
#33850=CARTESIAN_POINT('Ctrl Pts',(9.16037449240832,6.04505740584807,8.97950240170001));
#33851=CARTESIAN_POINT('Ctrl Pts',(9.15812982412392,6.04505708043623,8.9799612379583));
#33852=CARTESIAN_POINT('Ctrl Pts',(9.15588054189446,6.045057481699,8.98041291090022));
#33853=CARTESIAN_POINT('Ctrl Pts',(9.12236154441565,6.04506346135141,8.98714377997617));
#33854=CARTESIAN_POINT('Ctrl Pts',(9.08782147666207,6.04522615909127,8.99228271987963));
#33855=CARTESIAN_POINT('Ctrl Pts',(9.05247524549954,6.04556133675228,8.99560506194131));
#33856=CARTESIAN_POINT('Ctrl Pts',(9.02184037719226,6.04585183797877,8.99848456304182));
#33857=CARTESIAN_POINT('Ctrl Pts',(8.99060061916653,6.04627189451713,8.9999993959498));
#33858=CARTESIAN_POINT('Ctrl Pts',(8.958927440406,6.046831514125,8.99999999999996));
#33859=CARTESIAN_POINT('Origin',(8.958927440522,17.50736,8.));
#33860=CARTESIAN_POINT('Ctrl Pts',(8.95892745008802,1.55316848604618,8.99999999999974));
#33861=CARTESIAN_POINT('Ctrl Pts',(9.00275855065562,1.553943645885,8.99999899837848));
#33862=CARTESIAN_POINT('Ctrl Pts',(9.04683010695701,1.55447030043154,8.99709917174271));
#33863=CARTESIAN_POINT('Ctrl Pts',(9.0905895416497,1.55473749600761,8.99129104676408));
#33864=CARTESIAN_POINT('Ctrl Pts',(9.10512924205577,1.55482627557374,8.98936121385597));
#33865=CARTESIAN_POINT('Ctrl Pts',(9.11963440887108,1.5548864802363,8.9871107249482));
#33866=CARTESIAN_POINT('Ctrl Pts',(9.13408467274677,1.55491791715508,8.98454047352005));
#33867=CARTESIAN_POINT('Ctrl Pts',(9.16305493722674,1.55498094270669,8.97938756667391));
#33868=CARTESIAN_POINT('Ctrl Pts',(9.1918032220189,1.55492530956165,8.97295449863129));
#33869=CARTESIAN_POINT('Ctrl Pts',(9.22036197221234,1.55475387971182,8.96521883852068));
#33870=CARTESIAN_POINT('Ctrl Pts',(9.24892072240577,1.55458244986199,8.95748317841007));
#33871=CARTESIAN_POINT('Ctrl Pts',(9.27729079577433,1.55429521929521,8.94844478328275));
#33872=CARTESIAN_POINT('Ctrl Pts',(9.3054821343589,1.55388503037883,8.93802976721407));
#33873=CARTESIAN_POINT('Ctrl Pts',(9.33223490527492,1.55349577287412,8.92814621599014));
#33874=CARTESIAN_POINT('Ctrl Pts',(9.35881934236324,1.55299579736816,8.91702531744028));
#33875=CARTESIAN_POINT('Ctrl Pts',(9.38522933679278,1.55237888045198,8.90457933423687));
#33876=CARTESIAN_POINT('Ctrl Pts',(9.41074299990903,1.5517829011377,8.89255575644138));
#33877=CARTESIAN_POINT('Ctrl Pts',(9.43609438980752,1.55107773409733,8.87929518309596));
#33878=CARTESIAN_POINT('Ctrl Pts',(9.46124299424961,1.55025083931054,8.86468504225787));
#33879=CARTESIAN_POINT('Ctrl Pts',(9.46492613223733,1.55012973646334,8.86254531459026));
#33880=CARTESIAN_POINT('Ctrl Pts',(9.46860484909312,1.55000601088045,8.86037658442236));
#33881=CARTESIAN_POINT('Ctrl Pts',(9.47227894057115,1.54987961105733,8.85817844146731));
#33882=CARTESIAN_POINT('Ctrl Pts',(9.50104973858653,1.54888980887034,8.84096538965656));
#33883=CARTESIAN_POINT('Ctrl Pts',(9.52953374654615,1.54774065894391,8.82194974148639));
#33884=CARTESIAN_POINT('Ctrl Pts',(9.55743303390829,1.54642756706802,8.80110722892218));
#33885=CARTESIAN_POINT('Ctrl Pts',(9.5826050168278,1.5452428369406,8.78230218335038));
#33886=CARTESIAN_POINT('Ctrl Pts',(9.60730057475277,1.54392470007601,8.76201029506294));
#33887=CARTESIAN_POINT('Ctrl Pts',(9.63127322651056,1.5424733773,8.74023722147852));
#33888=CARTESIAN_POINT('Ctrl Pts',(8.9279389474,1.593171467102,8.997867580782));
#33889=CARTESIAN_POINT('Ctrl Pts',(8.937774434699,1.593573040994,8.99815844767));
#33890=CARTESIAN_POINT('Ctrl Pts',(9.006501123144,1.596194951904,8.999171711777));
#33891=CARTESIAN_POINT('Ctrl Pts',(9.135111717268,1.598711309997,8.987844921877));
#33892=CARTESIAN_POINT('Ctrl Pts',(9.310266674501,1.596356340012,8.940309843117));
#33893=CARTESIAN_POINT('Ctrl Pts',(9.480507438288,1.587786189889,8.858829792006));
#33894=CARTESIAN_POINT('Ctrl Pts',(9.591735407857,1.577057308712,8.776278000932));
#33895=CARTESIAN_POINT('Ctrl Pts',(9.646942416699,1.569906309379,8.724650180619));
#33896=CARTESIAN_POINT('Ctrl Pts',(9.653937650666,1.568966676907,8.717912247757));
#33897=CARTESIAN_POINT('Ctrl Pts',(8.93879197217,1.308923750487,9.021370782115));
#33898=CARTESIAN_POINT('Ctrl Pts',(8.948369635441,1.309314926618,9.021655024549));
#33899=CARTESIAN_POINT('Ctrl Pts',(9.015294451232,1.311868617701,9.022645787154));
#33900=CARTESIAN_POINT('Ctrl Pts',(9.140529817566,1.314314972079,9.011585510257));
#33901=CARTESIAN_POINT('Ctrl Pts',(9.311087401957,1.312004268657,8.965163068201));
#33902=CARTESIAN_POINT('Ctrl Pts',(9.47686644203,1.303627875584,8.885584897535));
#33903=CARTESIAN_POINT('Ctrl Pts',(9.585188255283,1.293147013991,8.804951761537));
#33904=CARTESIAN_POINT('Ctrl Pts',(9.638956159986,1.286161646375,8.754519895411));
#33905=CARTESIAN_POINT('Ctrl Pts',(9.645769108012,1.285243780476,8.747937983081));
#33906=CARTESIAN_POINT('Ctrl Pts',(8.953058771447,1.088595421228,8.840488165336));
#33907=CARTESIAN_POINT('Ctrl Pts',(8.960489669369,1.088898666868,8.840709537911));
#33908=CARTESIAN_POINT('Ctrl Pts',(9.012411237366,1.090878811164,8.841481514187));
#33909=CARTESIAN_POINT('Ctrl Pts',(9.10954285353,1.092783101822,8.832872893528));
#33910=CARTESIAN_POINT('Ctrl Pts',(9.241820527383,1.091020419799,8.796738876884));
#33911=CARTESIAN_POINT('Ctrl Pts',(9.370449136028,1.084567200145,8.734771759971));
#33912=CARTESIAN_POINT('Ctrl Pts',(9.454572911059,1.076465913557,8.671926426951));
#33913=CARTESIAN_POINT('Ctrl Pts',(9.496358150974,1.071056145855,8.632590758479));
#33914=CARTESIAN_POINT('Ctrl Pts',(9.501653299641,1.070345156809,8.62745655615));
#33915=CARTESIAN_POINT('Ctrl Pts',(8.962706216611,1.05624554634,8.557068315928));
#33916=CARTESIAN_POINT('Ctrl Pts',(8.967310175283,1.0564328393,8.557205973027));
#33917=CARTESIAN_POINT('Ctrl Pts',(8.999474917003,1.057657053701,8.557686068968));
#33918=CARTESIAN_POINT('Ctrl Pts',(9.059598485478,1.058852437488,8.552333807117));
#33919=CARTESIAN_POINT('Ctrl Pts',(9.141467770911,1.057832960287,8.529870957179));
#33920=CARTESIAN_POINT('Ctrl Pts',(9.2211753306,1.053949459686,8.491307907635));
#33921=CARTESIAN_POINT('Ctrl Pts',(9.273434242506,1.049019449244,8.452103844583));
#33922=CARTESIAN_POINT('Ctrl Pts',(9.299440270493,1.045708085229,8.427516741922));
#33923=CARTESIAN_POINT('Ctrl Pts',(9.302736725367,1.0452725983,8.424306784914));
#33924=CARTESIAN_POINT('Ctrl Pts',(0.001363716877125,7.004096037298,1.995067420053));
#33925=CARTESIAN_POINT('Ctrl Pts',(-0.0002547629821602,7.033536439795,1.947200740707));
#33926=CARTESIAN_POINT('Ctrl Pts',(-0.004372367677244,7.10872651687,1.819803089527));
#33927=CARTESIAN_POINT('Ctrl Pts',(-0.01069751864402,7.22832969105,1.590379225774));
#33928=CARTESIAN_POINT('Ctrl Pts',(-0.01714467798322,7.357904932227,1.288569665529));
#33929=CARTESIAN_POINT('Ctrl Pts',(-0.02256867464758,7.474904436555,0.9310228511914));
#33930=CARTESIAN_POINT('Ctrl Pts',(-0.02637651263401,7.564389025907,0.5171914444451));
#33931=CARTESIAN_POINT('Ctrl Pts',(-0.02742725699744,7.593855284484,0.2127089892188));
#33932=CARTESIAN_POINT('Ctrl Pts',(-0.02749825835039,7.599065112105,0.05030904096556));
#33933=CARTESIAN_POINT('Ctrl Pts',(-0.02750035356636,7.599263124611,0.04357390005572));
#33934=CARTESIAN_POINT('Ctrl Pts',(-0.02360189154764,7.332522732615,2.008012314209));
#33935=CARTESIAN_POINT('Ctrl Pts',(-0.007100235964038,7.363321141605,1.961090142431));
#33936=CARTESIAN_POINT('Ctrl Pts',(0.03503481007398,7.438156938294,1.831220908937));
#33937=CARTESIAN_POINT('Ctrl Pts',(0.1002819388273,7.542515456862,1.58377920092));
#33938=CARTESIAN_POINT('Ctrl Pts',(0.1674804264521,7.633451595482,1.250318159269));
#33939=CARTESIAN_POINT('Ctrl Pts',(0.2248447651456,7.687511126466,0.8568392396603));
#33940=CARTESIAN_POINT('Ctrl Pts',(0.2662490974893,7.689939339522,0.4123496126132));
#33941=CARTESIAN_POINT('Ctrl Pts',(0.2789069387192,7.649350136403,0.0983060253891));
#33942=CARTESIAN_POINT('Ctrl Pts',(0.2806593262459,7.61693316005,-0.06530116546358));
#33943=CARTESIAN_POINT('Ctrl Pts',(0.2807233254674,7.615570360117,-0.07207992811569));
#33944=CARTESIAN_POINT('Ctrl Pts',(0.2095583867952,7.565232260888,2.019596510591));
#33945=CARTESIAN_POINT('Ctrl Pts',(0.2389857802897,7.583483482567,1.964918501646));
#33946=CARTESIAN_POINT('Ctrl Pts',(0.3101581568233,7.623781352774,1.8140793846));
#33947=CARTESIAN_POINT('Ctrl Pts',(0.4068616564539,7.663606955409,1.532524925837));
#33948=CARTESIAN_POINT('Ctrl Pts',(0.4886889080965,7.670258563261,1.166376398115));
#33949=CARTESIAN_POINT('Ctrl Pts',(0.5374668975788,7.630189595634,0.7523865517109));
#33950=CARTESIAN_POINT('Ctrl Pts',(0.5443422263585,7.535897759144,0.306016547344));
#33951=CARTESIAN_POINT('Ctrl Pts',(0.5164520353948,7.437358052934,0.005351407090497));
#33952=CARTESIAN_POINT('Ctrl Pts',(0.4928891039185,7.378812409657,-0.1483861234052));
#33953=CARTESIAN_POINT('Ctrl Pts',(0.4918968454424,7.376374277029,-0.1547511527335));
#33954=CARTESIAN_POINT('Ctrl Pts',(0.5381945238366,7.539889032304,2.021739002091));
#33955=CARTESIAN_POINT('Ctrl Pts',(0.5663364060878,7.540440651784,1.956015197361));
#33956=CARTESIAN_POINT('Ctrl Pts',(0.6290746726959,7.536110224441,1.780336254062));
#33957=CARTESIAN_POINT('Ctrl Pts',(0.6951750183964,7.507132098316,1.472370815215));
#33958=CARTESIAN_POINT('Ctrl Pts',(0.7224092873361,7.442649702456,1.095301225047));
#33959=CARTESIAN_POINT('Ctrl Pts',(0.6972159851596,7.342926709167,0.690529825709));
#33960=CARTESIAN_POINT('Ctrl Pts',(0.6139081869805,7.209721985333,0.2723690173976));
#33961=CARTESIAN_POINT('Ctrl Pts',(0.5194992042506,7.105762363827,-0.001310753365661));
#33962=CARTESIAN_POINT('Ctrl Pts',(0.461141932074,7.050813259361,-0.1409866863127));
#33963=CARTESIAN_POINT('Ctrl Pts',(0.4587078974377,7.048535413961,-0.1467692430359));
#33964=CARTESIAN_POINT('Ctrl Pts',(0.0865688256819392,7.3235406542984,1.99263811287353));
#33965=CARTESIAN_POINT('Ctrl Pts',(0.0896802537077462,7.32912623877558,
1.96759743689578));
#33966=CARTESIAN_POINT('Ctrl Pts',(0.0923915043624595,7.3347911606353,1.94236105944537));
#33967=CARTESIAN_POINT('Ctrl Pts',(0.0947293636910101,7.34039900203038,
1.91744867197809));
#33968=CARTESIAN_POINT('Ctrl Pts',(0.0949482417161692,7.34092402645549,
1.91511629290624));
#33969=CARTESIAN_POINT('Ctrl Pts',(0.0951638771415863,7.34144856040776,
1.91278677211149));
#33970=CARTESIAN_POINT('Ctrl Pts',(0.0953763099453126,7.3419724980081,1.91046054583049));
#33971=CARTESIAN_POINT('Ctrl Pts',(0.0969299050857642,7.34580423630613,
1.89344804219467));
#33972=CARTESIAN_POINT('Ctrl Pts',(0.0983102863785579,7.34959839588947,
1.87660634057612));
#33973=CARTESIAN_POINT('Ctrl Pts',(0.0995681453181531,7.35344107264442,
1.85954655396089));
#33974=CARTESIAN_POINT('Ctrl Pts',(0.0997992999342739,7.35414723487152,
1.85641150574363));
#33975=CARTESIAN_POINT('Ctrl Pts',(0.100026202607223,7.35485500173232,1.85326901614998));
#33976=CARTESIAN_POINT('Ctrl Pts',(0.100249016916711,7.35556486233215,1.85011657530178));
#33977=CARTESIAN_POINT('Ctrl Pts',(0.100750378724828,7.35716214302145,1.84302316443752));
#33978=CARTESIAN_POINT('Ctrl Pts',(0.101231115787448,7.35877004683759,1.83587940956835));
#33979=CARTESIAN_POINT('Ctrl Pts',(0.101692526905404,7.36039395275203,1.82865566109089));
#33980=CARTESIAN_POINT('Ctrl Pts',(0.103474856351766,7.36666674336496,1.80075191295082));
#33981=CARTESIAN_POINT('Ctrl Pts',(0.104977614729166,7.37319161572645,1.77167311737816));
#33982=CARTESIAN_POINT('Ctrl Pts',(0.10616646031735,7.37984389128196,1.74175841581746));
#33983=CARTESIAN_POINT('Ctrl Pts',(0.107355305905534,7.38649616683747,1.71184371425676));
#33984=CARTESIAN_POINT('Ctrl Pts',(0.108232329401721,7.39327388476653,1.68109269976559));
#33985=CARTESIAN_POINT('Ctrl Pts',(0.108791895149357,7.4001768310032,1.64928217769217));
#33986=CARTESIAN_POINT('Ctrl Pts',(0.109166261829539,7.40479511415763,1.62799996091283));
#33987=CARTESIAN_POINT('Ctrl Pts',(0.109398357722325,7.40947001886123,1.60624309301958));
#33988=CARTESIAN_POINT('Ctrl Pts',(0.109487433858617,7.41418919456437,1.58401272756834));
#33989=CARTESIAN_POINT('Ctrl Pts',(0.109531499792492,7.41652376915564,1.57301537345363));
#33990=CARTESIAN_POINT('Ctrl Pts',(0.109540579661707,7.41886914803633,1.561902154465));
#33991=CARTESIAN_POINT('Ctrl Pts',(0.109514929847241,7.4212239270889,1.55067260771111));
#33992=CARTESIAN_POINT('Ctrl Pts',(0.109437430765813,7.42833872371927,1.51674333467875));
#33993=CARTESIAN_POINT('Ctrl Pts',(0.109042119817046,7.43553816021822,1.48175438125156));
#33994=CARTESIAN_POINT('Ctrl Pts',(0.108313731955709,7.44279124618812,1.44554679740932));
#33995=CARTESIAN_POINT('Ctrl Pts',(0.107585344094372,7.45004433215802,1.40933921356709));
#33996=CARTESIAN_POINT('Ctrl Pts',(0.106523548757051,7.4573515698644,1.37191311297681));
#33997=CARTESIAN_POINT('Ctrl Pts',(0.105117873628984,7.46467568199902,1.33311770345657));
#33998=CARTESIAN_POINT('Ctrl Pts',(0.104377954802098,7.46853094581526,1.31269658813082));
#33999=CARTESIAN_POINT('Ctrl Pts',(0.103543023712786,7.47239091384454,1.29189575125132));
#34000=CARTESIAN_POINT('Ctrl Pts',(0.102611872470959,7.47624431142032,1.27071260516852));
#34001=CARTESIAN_POINT('Ctrl Pts',(0.101774051099112,7.47971148055266,1.2516526590353));
#34002=CARTESIAN_POINT('Ctrl Pts',(0.100858336039839,7.48317330483615,1.23228319638487));
#34003=CARTESIAN_POINT('Ctrl Pts',(0.0998645221405797,7.48662201250552,
1.21260136918125));
#34004=CARTESIAN_POINT('Ctrl Pts',(0.097766187543305,7.49390359975632,1.17104523981968));
#34005=CARTESIAN_POINT('Ctrl Pts',(0.0953185572951622,7.50112665999997,
1.12809788131681));
#34006=CARTESIAN_POINT('Ctrl Pts',(0.0925150010827101,7.50821076792826,
1.08370319344878));
#34007=CARTESIAN_POINT('Ctrl Pts',(0.089711444870258,7.51529487585655,1.03930850558076));
#34008=CARTESIAN_POINT('Ctrl Pts',(0.0865511551028964,7.52224148615219,
0.993466772008885));
#34009=CARTESIAN_POINT('Ctrl Pts',(0.0830270933744481,7.52899459767804,
0.945862005357544));
#34010=CARTESIAN_POINT('Ctrl Pts',(0.0821381954945036,7.530697980587,0.933854333695601));
#34011=CARTESIAN_POINT('Ctrl Pts',(0.081226180044907,7.53238887179564,0.921734422666414));
#34012=CARTESIAN_POINT('Ctrl Pts',(0.0802903601283761,7.53406600471985,
0.909495233375608));
#34013=CARTESIAN_POINT('Ctrl Pts',(0.0775160945255589,7.5390379144867,0.873211797581972));
#34014=CARTESIAN_POINT('Ctrl Pts',(0.0745326823159648,7.54389003125133,
0.835880050581168));
#34015=CARTESIAN_POINT('Ctrl Pts',(0.0713215509276857,7.54858645422804,
0.797314112004502));
#34016=CARTESIAN_POINT('Ctrl Pts',(0.0672743784190882,7.55450562465796,
0.748707254326407));
#34017=CARTESIAN_POINT('Ctrl Pts',(0.0628650243611779,7.56017951647996,
0.698140410147152));
#34018=CARTESIAN_POINT('Ctrl Pts',(0.0580773486278632,7.56549672991315,
0.645280546452683));
#34019=CARTESIAN_POINT('Ctrl Pts',(0.0577849862459548,7.56582142884245,
0.642052626159432));
#34020=CARTESIAN_POINT('Ctrl Pts',(0.057491216650073,7.56614478165179,0.638816155811791));
#34021=CARTESIAN_POINT('Ctrl Pts',(0.0571960377183247,7.5664667564898,0.635571059829908));
#34022=CARTESIAN_POINT('Ctrl Pts',(0.0532958632914503,7.5707209829749,0.592693879245485));
#34023=CARTESIAN_POINT('Ctrl Pts',(0.0491499956495321,7.57473650573253,
0.548310744947044));
#34024=CARTESIAN_POINT('Ctrl Pts',(0.0447657824929133,7.57841830892359,
0.502354796048155));
#34025=CARTESIAN_POINT('Ctrl Pts',(0.0433844758662343,7.57957831163429,
0.487875742571131));
#34026=CARTESIAN_POINT('Ctrl Pts',(0.0419795965094829,7.58070504176636,
0.473240574471837));
#34027=CARTESIAN_POINT('Ctrl Pts',(0.0405516110274916,7.58179564957126,
0.458447294243215));
#34028=CARTESIAN_POINT('Ctrl Pts',(0.0352357117822026,7.58585560765916,
0.403376995424063));
#34029=CARTESIAN_POINT('Ctrl Pts',(0.0295974679152405,7.58941730052929,
0.346115563689829));
#34030=CARTESIAN_POINT('Ctrl Pts',(0.0236363315001921,7.59231304495109,
0.28649801517568));
#34031=CARTESIAN_POINT('Ctrl Pts',(0.0229136519574967,7.59266410137872,
0.279270470006933));
#34032=CARTESIAN_POINT('Ctrl Pts',(0.0221862695618803,7.59300533008682,
0.272008321185318));
#34033=CARTESIAN_POINT('Ctrl Pts',(0.0214542211065908,7.59333639705194,
0.264711295552353));
#34034=CARTESIAN_POINT('Ctrl Pts',(0.0156433037850095,7.59596436894136,
0.206788336573017));
#34035=CARTESIAN_POINT('Ctrl Pts',(0.00953650453228541,7.59795273247266,
0.146666268293311));
#34036=CARTESIAN_POINT('Ctrl Pts',(0.00317281194423555,7.59911587089843,
0.0844485241839117));
#34037=CARTESIAN_POINT('Ctrl Pts',(0.00212199046213768,7.59930793719131,
0.0741746554868914));
#34038=CARTESIAN_POINT('Ctrl Pts',(0.00106426940600786,7.5994774832001,
0.0638436870231593));
#34039=CARTESIAN_POINT('Ctrl Pts',(-4.55832343463506E-8,7.59962364606423,
0.0534561336397867));
#34040=CARTESIAN_POINT('Origin',(-1.165507426858E-9,7.09967345946,0.04642263385286));
#34041=CARTESIAN_POINT('Ctrl Pts',(0.09332729536784,7.333647414405,2.027339375446));
#34042=CARTESIAN_POINT('Ctrl Pts',(0.0956460765109,7.337274567028,2.020940474449));
#34043=CARTESIAN_POINT('Ctrl Pts',(0.1067234777855,7.354783699243,1.98987166704));
#34044=CARTESIAN_POINT('Ctrl Pts',(0.1252614819808,7.385575923908,1.933661042191));
#34045=CARTESIAN_POINT('Ctrl Pts',(0.1483230597314,7.42617634589,1.855915420958));
#34046=CARTESIAN_POINT('Ctrl Pts',(0.1706856731413,7.467450488292,1.772637372698));
#34047=CARTESIAN_POINT('Ctrl Pts',(0.1930020158897,7.510044352663,1.681442257421));
#34048=CARTESIAN_POINT('Ctrl Pts',(0.2153249421398,7.553626038292,1.581617848906));
#34049=CARTESIAN_POINT('Ctrl Pts',(0.237760929357,7.597792410414,1.472368077024));
#34050=CARTESIAN_POINT('Ctrl Pts',(0.2604508155607,7.642090028244,1.352628361367));
#34051=CARTESIAN_POINT('Ctrl Pts',(0.2834723960102,7.685792567441,1.221593810851));
#34052=CARTESIAN_POINT('Ctrl Pts',(0.3069634986954,7.728092190564,1.078167578903));
#34053=CARTESIAN_POINT('Ctrl Pts',(0.3311487111769,7.768064414624,0.9208497005947));
#34054=CARTESIAN_POINT('Ctrl Pts',(0.3564829869057,7.804698725932,0.7467239997499));
#34055=CARTESIAN_POINT('Ctrl Pts',(0.383183258108,7.836191149907,0.5536747851937));
#34056=CARTESIAN_POINT('Ctrl Pts',(0.4118738384147,7.860119523589,0.3402017808901));
#34057=CARTESIAN_POINT('Ctrl Pts',(0.4323948723823,7.868947086026,0.183227181261));
#34058=CARTESIAN_POINT('Ctrl Pts',(0.4433244432103,7.871063970647,0.0981968847509));
#34059=CARTESIAN_POINT('Ctrl Pts',(0.4441525558925,7.871209365081,0.09174594482544));
#34060=CARTESIAN_POINT('Ctrl Pts',(0.00413371639593,7.185905309626,1.91818759396));
#34061=CARTESIAN_POINT('Ctrl Pts',(0.006375610685106,7.18924784677,1.912236954105));
#34062=CARTESIAN_POINT('Ctrl Pts',(0.01709859516906,7.205399755638,1.883314369697));
#34063=CARTESIAN_POINT('Ctrl Pts',(0.03514371433924,7.23393502954,1.830747145249));
#34064=CARTESIAN_POINT('Ctrl Pts',(0.05770123147572,7.271715716269,1.757747888332));
#34065=CARTESIAN_POINT('Ctrl Pts',(0.07967986153062,7.310277891777,1.67924388339));
#34066=CARTESIAN_POINT('Ctrl Pts',(0.1016848560021,7.350182806674,1.593045679998));
#34067=CARTESIAN_POINT('Ctrl Pts',(0.123750946579,7.391096468068,1.498504779354));
#34068=CARTESIAN_POINT('Ctrl Pts',(0.1459810956979,7.432635330052,1.394842391727));
#34069=CARTESIAN_POINT('Ctrl Pts',(0.1685009069597,7.474346978144,1.281076556188));
#34070=CARTESIAN_POINT('Ctrl Pts',(0.1913848392552,7.515534476051,1.156432362992));
#34071=CARTESIAN_POINT('Ctrl Pts',(0.2147620673246,7.555413295895,1.019885111452));
#34072=CARTESIAN_POINT('Ctrl Pts',(0.2388605698404,7.593100119069,0.8699663883089));
#34073=CARTESIAN_POINT('Ctrl Pts',(0.2641204729043,7.62760311364,0.7039575843834));
#34074=CARTESIAN_POINT('Ctrl Pts',(0.2907706259586,7.657204843238,0.5197608497961));
#34075=CARTESIAN_POINT('Ctrl Pts',(0.3194378379588,7.679569502558,0.3159115398518));
#34076=CARTESIAN_POINT('Ctrl Pts',(0.3399248718625,7.687650272031,0.1661433025018));
#34077=CARTESIAN_POINT('Ctrl Pts',(0.3508467599435,7.689487914492,0.08495485013407));
#34078=CARTESIAN_POINT('Ctrl Pts',(0.3516743579076,7.689612809971,0.07879497185148));
#34079=CARTESIAN_POINT('Ctrl Pts',(-0.1656119288838,7.120545824473,1.825386409491));
#34080=CARTESIAN_POINT('Ctrl Pts',(-0.1635163591258,7.123519766875,1.81996392764));
#34081=CARTESIAN_POINT('Ctrl Pts',(-0.1534678705812,7.137930212453,1.79353716736));
#34082=CARTESIAN_POINT('Ctrl Pts',(-0.1363607683355,7.163697474219,1.744942128327));
#34083=CARTESIAN_POINT('Ctrl Pts',(-0.1147625365556,7.198182465273,1.676772747774));
#34084=CARTESIAN_POINT('Ctrl Pts',(-0.09351467101442,7.233744731282,1.602739197824));
#34085=CARTESIAN_POINT('Ctrl Pts',(-0.07210220814429,7.270802639682,1.520912659697));
#34086=CARTESIAN_POINT('Ctrl Pts',(-0.05052490541031,7.308992126025,1.430734790665));
#34087=CARTESIAN_POINT('Ctrl Pts',(-0.0286864898805,7.347943299813,1.331405236481));
#34088=CARTESIAN_POINT('Ctrl Pts',(-0.006490350805654,7.387171471204,1.222048142703));
#34089=CARTESIAN_POINT('Ctrl Pts',(0.01613162121186,7.425990916832,1.101895162335));
#34090=CARTESIAN_POINT('Ctrl Pts',(0.03929213278287,7.463608317969,0.9700014892299));
#34091=CARTESIAN_POINT('Ctrl Pts',(0.06322561625506,7.499163150947,0.8248557918099));
#34092=CARTESIAN_POINT('Ctrl Pts',(0.0883439795788,7.531628832607,0.6639649220211));
#34093=CARTESIAN_POINT('Ctrl Pts',(0.1148987520299,7.559346495031,0.4851100355565));
#34094=CARTESIAN_POINT('Ctrl Pts',(0.1435214914534,7.579991317253,0.2867927966161));
#34095=CARTESIAN_POINT('Ctrl Pts',(0.163943819323,7.587052319387,0.1413866086485));
#34096=CARTESIAN_POINT('Ctrl Pts',(0.1748512775237,7.588418185354,0.0624210760095));
#34097=CARTESIAN_POINT('Ctrl Pts',(0.1756779116267,7.58850768362,0.05642892400282));
#34098=CARTESIAN_POINT('Ctrl Pts',(-0.3607780994109,7.158797009499,1.779076638338));
#34099=CARTESIAN_POINT('Ctrl Pts',(-0.3588507672437,7.161438093464,1.774090671374));
#34100=CARTESIAN_POINT('Ctrl Pts',(-0.3495777848353,7.174288444165,1.749698719792));
#34101=CARTESIAN_POINT('Ctrl Pts',(-0.3335491737094,7.197675652681,1.70411452853));
#34102=CARTESIAN_POINT('Ctrl Pts',(-0.3130538865687,7.229459393784,1.639289845029));
#34103=CARTESIAN_POINT('Ctrl Pts',(-0.2926462223267,7.262708145696,1.56797120654));
#34104=CARTESIAN_POINT('Ctrl Pts',(-0.2719150265568,7.297685667349,1.488471217684));
#34105=CARTESIAN_POINT('Ctrl Pts',(-0.2508997108556,7.333979610279,1.400318838748));
#34106=CARTESIAN_POINT('Ctrl Pts',(-0.2295116935927,7.371223370819,1.302660309974));
#34107=CARTESIAN_POINT('Ctrl Pts',(-0.2076876987406,7.408877164792,1.194714908186));
#34108=CARTESIAN_POINT('Ctrl Pts',(-0.1853669172732,7.4462446648,1.07569529903));
#34109=CARTESIAN_POINT('Ctrl Pts',(-0.1624555769196,7.482494516028,0.9447183706797));
#34110=CARTESIAN_POINT('Ctrl Pts',(-0.1387118251766,7.516763216746,0.8001693426502));
#34111=CARTESIAN_POINT('Ctrl Pts',(-0.1137561980987,7.547947286417,0.6397351948215));
#34112=CARTESIAN_POINT('Ctrl Pts',(-0.0873110901226,7.574399433416,0.4609765504098));
#34113=CARTESIAN_POINT('Ctrl Pts',(-0.05873948333615,7.593726880203,0.2623030025697));
#34114=CARTESIAN_POINT('Ctrl Pts',(-0.03839155165445,7.599826349973,0.1169978048482));
#34115=CARTESIAN_POINT('Ctrl Pts',(-0.02750058379875,7.600681132993,0.03791428735155));
#34116=CARTESIAN_POINT('Ctrl Pts',(-0.02667504964837,7.600731832416,0.03191205058198));
#34117=CARTESIAN_POINT('Ctrl Pts',(0.006092677290347,7.599378811355,0.0686831784786));
#34118=CARTESIAN_POINT('Ctrl Pts',(0.003734755645105,7.599467813605,0.06378738843317));
#34119=CARTESIAN_POINT('Ctrl Pts',(-0.0004662461470239,7.599626415391,0.05398924362921));
#34120=CARTESIAN_POINT('Ctrl Pts',(-0.005281917817338,7.599808258387,0.03903695947461));
#34121=CARTESIAN_POINT('Ctrl Pts',(-0.008492810869693,7.599929521181,0.02433820698079));
#34122=CARTESIAN_POINT('Ctrl Pts',(-0.01020745239528,7.599994282083,0.009761485286655));
#34123=CARTESIAN_POINT('Ctrl Pts',(-0.01046402051099,7.600003972854,-0.005086971198367));
#34124=CARTESIAN_POINT('Ctrl Pts',(-0.009120895515257,7.599953242924,-0.02060522202386));
#34125=CARTESIAN_POINT('Ctrl Pts',(-0.005888618218437,7.599831169114,-0.03701638653157));
#34126=CARTESIAN_POINT('Ctrl Pts',(-0.0007646346168158,7.599637680482,-0.05329605734118));
#34127=CARTESIAN_POINT('Ctrl Pts',(0.003740802961434,7.599467585381,-0.06380088841689));
#34128=CARTESIAN_POINT('Ctrl Pts',(0.006102566100798,7.599378439467,-0.06870005169305));
#34129=CARTESIAN_POINT('Ctrl Pts',(0.01191131196756,7.59942502026,0.0658677090234));
#34130=CARTESIAN_POINT('Ctrl Pts',(0.009633710571033,7.599510770099,0.06113683658055));
#34131=CARTESIAN_POINT('Ctrl Pts',(0.005585856903677,7.599663190864,0.05169022499271));
#34132=CARTESIAN_POINT('Ctrl Pts',(0.000963349003167,7.599837277401,0.03732842304098));
#34133=CARTESIAN_POINT('Ctrl Pts',(-0.002109362182591,7.599953011217,0.02325255344247));
#34134=CARTESIAN_POINT('Ctrl Pts',(-0.003746892804695,7.600014693386,0.009321455251517));
#34135=CARTESIAN_POINT('Ctrl Pts',(-0.003991703715731,7.600023915162,-0.004857311815456));
#34136=CARTESIAN_POINT('Ctrl Pts',(-0.002709569211279,7.599975619204,-0.01968209560348));
#34137=CARTESIAN_POINT('Ctrl Pts',(0.0003816499432407,7.599859185572,-0.03538922245973));
#34138=CARTESIAN_POINT('Ctrl Pts',(0.005298322938301,7.599674017825,-0.05102182560792));
#34139=CARTESIAN_POINT('Ctrl Pts',(0.009639551531228,7.599510550216,-0.0611499027721));
#34140=CARTESIAN_POINT('Ctrl Pts',(0.01192093360296,7.599424658936,-0.06588431051089));
#34141=CARTESIAN_POINT('Ctrl Pts',(0.01772876858228,7.599345883008,0.06305053973491));
#34142=CARTESIAN_POINT('Ctrl Pts',(0.01553153160734,7.599428378633,0.0584846866516));
#34143=CARTESIAN_POINT('Ctrl Pts',(0.01163691029,7.599574614956,0.04938982358297));
#34144=CARTESIAN_POINT('Ctrl Pts',(0.007207672391512,7.599740940741,0.03561886170935));
#34145=CARTESIAN_POINT('Ctrl Pts',(0.004273219066756,7.59985114252,0.02216624982538));
#34146=CARTESIAN_POINT('Ctrl Pts',(0.002712841755993,7.599909744253,0.00888116198926));
#34147=CARTESIAN_POINT('Ctrl Pts',(0.002479794515622,7.599918496774,-0.004627515069058));
#34148=CARTESIAN_POINT('Ctrl Pts',(0.0037009049865,7.599872636135,-0.01875841664829));
#34149=CARTESIAN_POINT('Ctrl Pts',(0.006650988422478,7.5997618458,-0.03376108270729));
#34150=CARTESIAN_POINT('Ctrl Pts',(0.01136023679858,7.599585003543,-0.0487462262884));
#34151=CARTESIAN_POINT('Ctrl Pts',(0.01553716609792,7.599428167097,-0.05849731878176));
#34152=CARTESIAN_POINT('Ctrl Pts',(0.0177381228957,7.599345532253,-0.06306686930571));
#34153=CARTESIAN_POINT('Ctrl Pts',(0.02354285942058,7.59914142936,0.0602327300384));
#34154=CARTESIAN_POINT('Ctrl Pts',(0.02142600081824,7.599220670193,0.05583193601436));
#34155=CARTESIAN_POINT('Ctrl Pts',(0.01768463845156,7.599360720975,0.04708890448941));
#34156=CARTESIAN_POINT('Ctrl Pts',(0.01344870410615,7.599519284634,0.03390891837772));
#34157=CARTESIAN_POINT('Ctrl Pts',(0.01065253264352,7.599623953398,0.02107970464507));
#34158=CARTESIAN_POINT('Ctrl Pts',(0.009169322037672,7.599679474151,0.00844077107666));
#34159=CARTESIAN_POINT('Ctrl Pts',(0.008948040510102,7.599687757336,-0.004397667376584));
#34160=CARTESIAN_POINT('Ctrl Pts',(0.01010811635383,7.599644332445,-0.01783453251719));
#34161=CARTESIAN_POINT('Ctrl Pts',(0.01291703957055,7.599539186405,-0.03213257955283));
#34162=CARTESIAN_POINT('Ctrl Pts',(0.01741882731943,7.599370671111,-0.04647011514499));
#34163=CARTESIAN_POINT('Ctrl Pts',(0.02143142880335,7.599220467005,-0.05584413397716));
#34164=CARTESIAN_POINT('Ctrl Pts',(0.02355194636561,7.599141089176,-0.06024878760501));
#34165=CARTESIAN_POINT('Origin',(-3.054477616688E-10,7.099673459428,-0.04642263614025));
#34166=CARTESIAN_POINT('Ctrl Pts',(-0.02750316139292,7.599262953893,-0.04358922770243));
#34167=CARTESIAN_POINT('Ctrl Pts',(-0.02750089427335,7.599065008369,-0.05032035313669));
#34168=CARTESIAN_POINT('Ctrl Pts',(-0.02742485534672,7.593772444205,-0.2152695514171));
#34169=CARTESIAN_POINT('Ctrl Pts',(-0.02635280173775,7.563632607212,-0.5234275620995));
#34170=CARTESIAN_POINT('Ctrl Pts',(-0.02245453925618,7.472273113365,-0.9410069594233));
#34171=CARTESIAN_POINT('Ctrl Pts',(-0.01694441566883,7.353683066177,-1.299793310531));
#34172=CARTESIAN_POINT('Ctrl Pts',(-0.0104233500914,7.222960376541,-1.601669677065));
#34173=CARTESIAN_POINT('Ctrl Pts',(-0.00415034249476,7.104640819788,-1.82694866898));
#34174=CARTESIAN_POINT('Ctrl Pts',(-0.000137982512947,7.031410069502,-1.950653360374));
#34175=CARTESIAN_POINT('Ctrl Pts',(0.00136439425857,7.004084473842,-1.995080420042));
#34176=CARTESIAN_POINT('Ctrl Pts',(0.2807219033003,7.615574941146,0.07206410546599));
#34177=CARTESIAN_POINT('Ctrl Pts',(0.2806561737659,7.616937054043,0.06529447791626));
#34178=CARTESIAN_POINT('Ctrl Pts',(0.2788362287103,7.649866050139,-0.1007651614224));
#34179=CARTESIAN_POINT('Ctrl Pts',(0.265938333337,7.690613712512,-0.4189036102997));
#34180=CARTESIAN_POINT('Ctrl Pts',(0.2235950281924,7.686867087972,-0.8676904200621));
#34181=CARTESIAN_POINT('Ctrl Pts',(0.1653583372218,7.630983300808,-1.262746140425));
#34182=CARTESIAN_POINT('Ctrl Pts',(0.09742648092697,7.538286908882,-1.596177405319));
#34183=CARTESIAN_POINT('Ctrl Pts',(0.03275103019119,7.434243995127,-1.838700874606));
#34184=CARTESIAN_POINT('Ctrl Pts',(-0.008292099066438,7.361100787874,-1.964475131896));
#34185=CARTESIAN_POINT('Ctrl Pts',(-0.02360837126205,7.33251617638,-2.008025395665));
#34186=CARTESIAN_POINT('Ctrl Pts',(0.4918992607783,7.376380576182,0.1547359142356));
#34187=CARTESIAN_POINT('Ctrl Pts',(0.4928878083094,7.378817517877,0.1483835574526));
#34188=CARTESIAN_POINT('Ctrl Pts',(0.5167500083095,7.438288421961,-0.007565532271832));
#34189=CARTESIAN_POINT('Ctrl Pts',(0.5448287089649,7.537827128944,-0.3123858450142));
#34190=CARTESIAN_POINT('Ctrl Pts',(0.536824011986,7.632025775638,-0.7634855185152));
#34191=CARTESIAN_POINT('Ctrl Pts',(0.4864905623783,7.670854401701,-1.179726783912));
#34192=CARTESIAN_POINT('Ctrl Pts',(0.403012509611,7.662572001204,-1.546392400176));
#34193=CARTESIAN_POINT('Ctrl Pts',(0.3064646604075,7.621844952183,-1.822739961704));
#34194=CARTESIAN_POINT('Ctrl Pts',(0.2368627668342,7.582171578457,-1.968863315844));
#34195=CARTESIAN_POINT('Ctrl Pts',(0.2095495364899,7.56523383601,-2.019612509741));
#34196=CARTESIAN_POINT('Ctrl Pts',(0.4587131901116,7.048540031596,0.1467549726054));
#34197=CARTESIAN_POINT('Ctrl Pts',(0.4611428327528,7.050816780058,0.140984574553));
#34198=CARTESIAN_POINT('Ctrl Pts',(0.5203496374819,7.106634506402,-0.0006860175177874));
#34199=CARTESIAN_POINT('Ctrl Pts',(0.615766516957,7.21185561697,-0.2781802504272));
#34200=CARTESIAN_POINT('Ctrl Pts',(0.6987262516412,7.34600605939,-0.7010848027864));
#34201=CARTESIAN_POINT('Ctrl Pts',(0.7224328581585,7.445482591648,-1.108648913658));
#34202=CARTESIAN_POINT('Ctrl Pts',(0.6931602429223,7.509115316905,-1.487044303164));
#34203=CARTESIAN_POINT('Ctrl Pts',(0.6260499982531,7.536574687926,-1.790200141908));
#34204=CARTESIAN_POINT('Ctrl Pts',(0.5643084424037,7.540405136517,-1.96075674842));
#34205=CARTESIAN_POINT('Ctrl Pts',(0.5381889316308,7.539895380596,-2.021758679482));
#34206=CARTESIAN_POINT('Ctrl Pts',(-9.09791454320777E-7,7.59962392227978,
-0.0534607251838897));
#34207=CARTESIAN_POINT('Ctrl Pts',(0.0065283531795287,7.59872753669475,
-0.117157269822079));
#34208=CARTESIAN_POINT('Ctrl Pts',(0.0127944512896137,7.59695439925381,
-0.178629296927244));
#34209=CARTESIAN_POINT('Ctrl Pts',(0.0187482387130406,7.59450601408332,
-0.237760296202854));
#34210=CARTESIAN_POINT('Ctrl Pts',(0.0205286496400157,7.59377385295613,
-0.255442734245402));
#34211=CARTESIAN_POINT('Ctrl Pts',(0.0222814724519866,7.59298124399135,
-0.272915929949871));
#34212=CARTESIAN_POINT('Ctrl Pts',(0.0240062157852462,7.59213345316372,
-0.290177057808215));
#34213=CARTESIAN_POINT('Ctrl Pts',(0.0299524098926225,7.58921062474841,
-0.34968621188274));
#34214=CARTESIAN_POINT('Ctrl Pts',(0.0355590332814241,7.58563490866102,
-0.406673539550654));
#34215=CARTESIAN_POINT('Ctrl Pts',(0.0408307692423231,7.58158039917757,
-0.461351966728956));
#34216=CARTESIAN_POINT('Ctrl Pts',(0.0422015720466334,7.58052611022773,
-0.475569928680623));
#34217=CARTESIAN_POINT('Ctrl Pts',(0.0435499057751943,7.57943924715598,
-0.489631862685936));
#34218=CARTESIAN_POINT('Ctrl Pts',(0.0448761834513,7.57832247795482,-0.503541692217891));
#34219=CARTESIAN_POINT('Ctrl Pts',(0.0450702352681292,7.57815907997537,
-0.50557688269202));
#34220=CARTESIAN_POINT('Ctrl Pts',(0.0452638122698697,7.57799504118337,
-0.507608814416376));
#34221=CARTESIAN_POINT('Ctrl Pts',(0.0454569139117579,7.57783036882969,
-0.509637503453062));
#34222=CARTESIAN_POINT('Ctrl Pts',(0.0504911583145555,7.57353728842532,
-0.562526315418047));
#34223=CARTESIAN_POINT('Ctrl Pts',(0.0552009765518408,7.56881802512354,
-0.613211073658562));
#34224=CARTESIAN_POINT('Ctrl Pts',(0.0595853187064746,7.56379768086552,
-0.661979072988505));
#34225=CARTESIAN_POINT('Ctrl Pts',(0.0606025057451536,7.56263293848711,
-0.67329346750224));
#34226=CARTESIAN_POINT('Ctrl Pts',(0.0616022346632844,7.56145177499226,
-0.684504695951582));
#34227=CARTESIAN_POINT('Ctrl Pts',(0.0625845886514869,7.56025538274919,
-0.695616355735607));
#34228=CARTESIAN_POINT('Ctrl Pts',(0.0673140541170907,7.5544954470591,-0.749112561630028));
#34229=CARTESIAN_POINT('Ctrl Pts',(0.0716395926981727,7.54838661205288,
-0.800300379710368));
#34230=CARTESIAN_POINT('Ctrl Pts',(0.075594696585323,7.54203220392621,-0.849588597925932));
#34231=CARTESIAN_POINT('Ctrl Pts',(0.0761378573316066,7.54115954288904,
-0.856357427810763));
#34232=CARTESIAN_POINT('Ctrl Pts',(0.0766740369073583,7.54028217083988,
-0.863090434326044));
#34233=CARTESIAN_POINT('Ctrl Pts',(0.0772033241581099,7.53940028223977,
-0.869788678684179));
#34234=CARTESIAN_POINT('Ctrl Pts',(0.0785440273151084,7.53716642750662,
-0.886755566408276));
#34235=CARTESIAN_POINT('Ctrl Pts',(0.0798407302385532,7.53490375412732,
-0.903499201470491));
#34236=CARTESIAN_POINT('Ctrl Pts',(0.0810937204904941,7.53261600119494,
-0.920028260064166));
#34237=CARTESIAN_POINT('Ctrl Pts',(0.0839373260662721,7.5274240477983,-0.957540222433014));
#34238=CARTESIAN_POINT('Ctrl Pts',(0.0865557106729754,7.52210382157748,
-0.993947062290873));
#34239=CARTESIAN_POINT('Ctrl Pts',(0.0889539161282571,7.51669797919463,
-1.02934740992906));
#34240=CARTESIAN_POINT('Ctrl Pts',(0.092408853249567,7.50891013704819,-1.08034636620825));
#34241=CARTESIAN_POINT('Ctrl Pts',(0.0954064872307011,7.5009451628879,-1.12925696355173));
#34242=CARTESIAN_POINT('Ctrl Pts',(0.0979571981160565,7.4929211943923,-1.1762068370932));
#34243=CARTESIAN_POINT('Ctrl Pts',(0.0999421648727422,7.48667693095503,
-1.21274329394743));
#34244=CARTESIAN_POINT('Ctrl Pts',(0.101656839723846,7.48039623554083,-1.24809198876685));
#34245=CARTESIAN_POINT('Ctrl Pts',(0.103114408059408,7.47412058325023,-1.28234280769482));
#34246=CARTESIAN_POINT('Ctrl Pts',(0.103529836038339,7.47233193191639,-1.29210478463738));
#34247=CARTESIAN_POINT('Ctrl Pts',(0.103924381198659,7.47054363202985,-1.30177759317101));
#34248=CARTESIAN_POINT('Ctrl Pts',(0.104298386010432,7.4687566434487,-1.31136316830816));
#34249=CARTESIAN_POINT('Ctrl Pts',(0.105984622059959,7.46069983650188,-1.35458063996335));
#34250=CARTESIAN_POINT('Ctrl Pts',(0.10725238266638,7.45267074068681,-1.39602675468791));
#34251=CARTESIAN_POINT('Ctrl Pts',(0.108116417619798,7.44468165502368,-1.43608914702523));
#34252=CARTESIAN_POINT('Ctrl Pts',(0.108980452573216,7.43669256936054,-1.47615153936256));
#34253=CARTESIAN_POINT('Ctrl Pts',(0.109440821161578,7.42874335524718,-1.51483017857665));
#34254=CARTESIAN_POINT('Ctrl Pts',(0.109518134026665,7.42097012443101,-1.55188588983467));
#34255=CARTESIAN_POINT('Ctrl Pts',(0.109549379528338,7.41782862273911,-1.56686171936613));
#34256=CARTESIAN_POINT('Ctrl Pts',(0.109517733599107,7.41471541142924,-1.58157153761866));
#34257=CARTESIAN_POINT('Ctrl Pts',(0.1094247017107,7.41162697964378,-1.59605530105345));
#34258=CARTESIAN_POINT('Ctrl Pts',(0.109287538484548,7.40707349508385,-1.61740969634247));
#34259=CARTESIAN_POINT('Ctrl Pts',(0.109017347905158,7.40257412495728,-1.63827290333177));
#34260=CARTESIAN_POINT('Ctrl Pts',(0.108614123231762,7.39811498650203,-1.65876475481342));
#34261=CARTESIAN_POINT('Ctrl Pts',(0.108197298559464,7.3935054498145,-1.67994775734813));
#34262=CARTESIAN_POINT('Ctrl Pts',(0.107636013113357,7.38893509013303,-1.70073180908713));
#34263=CARTESIAN_POINT('Ctrl Pts',(0.106916313695485,7.38432485973754,-1.72156283502745));
#34264=CARTESIAN_POINT('Ctrl Pts',(0.106467581648175,7.38145038454336,-1.73455096407919));
#34265=CARTESIAN_POINT('Ctrl Pts',(0.105956508353038,7.37856013433668,-1.74755699928645));
#34266=CARTESIAN_POINT('Ctrl Pts',(0.105370932926494,7.37563206590809,-1.76068425372961));
#34267=CARTESIAN_POINT('Ctrl Pts',(0.104614139175394,7.37184784992309,-1.77764982926665));
#34268=CARTESIAN_POINT('Ctrl Pts',(0.10373062228697,7.36799661236927,-1.79481376372923));
#34269=CARTESIAN_POINT('Ctrl Pts',(0.102682811222867,7.36401912913252,-1.81251182586846));
#34270=CARTESIAN_POINT('Ctrl Pts',(0.101740077804235,7.36044051987958,-1.82843507309811));
#34271=CARTESIAN_POINT('Ctrl Pts',(0.100664403176793,7.35675971869643,-1.84479084066697));
#34272=CARTESIAN_POINT('Ctrl Pts',(0.0993976726188921,7.35292665555006,
-1.86180605447627));
#34273=CARTESIAN_POINT('Ctrl Pts',(0.0992357132673436,7.35243657467393,
-1.86398155500227));
#34274=CARTESIAN_POINT('Ctrl Pts',(0.0990705841488978,7.35194399434768,
-1.86616780777751));
#34275=CARTESIAN_POINT('Ctrl Pts',(0.0989021290733927,7.35144880143277,
-1.86836524213778));
#34276=CARTESIAN_POINT('Ctrl Pts',(0.0971030163999783,7.3461601044533,-1.89183400373318));
#34277=CARTESIAN_POINT('Ctrl Pts',(0.0949363222751479,7.34058460186587,
-1.91658901567847));
#34278=CARTESIAN_POINT('Ctrl Pts',(0.0922869113983884,7.33481922105929,
-1.94227889863271));
#34279=CARTESIAN_POINT('Ctrl Pts',(0.0905915320651806,7.33112990750159,
-1.95871806139723));
#34280=CARTESIAN_POINT('Ctrl Pts',(0.0886979474294951,7.32736294710167,
-1.97553922387949));
#34281=CARTESIAN_POINT('Ctrl Pts',(0.0865694808503494,7.32354392192484,
-1.99264108439717));
#34282=CARTESIAN_POINT('Ctrl Pts',(0.4441505898026,7.871213650645,-0.09177744215336));
#34283=CARTESIAN_POINT('Ctrl Pts',(0.4433243095181,7.871068290275,-0.09821494507687));
#34284=CARTESIAN_POINT('Ctrl Pts',(0.431912656318,7.868855063663,-0.1870059243154));
#34285=CARTESIAN_POINT('Ctrl Pts',(0.4105084687883,7.85942783985,-0.3505980872272));
#34286=CARTESIAN_POINT('Ctrl Pts',(0.3806737777609,7.833726074243,-0.572222828126));
#34287=CARTESIAN_POINT('Ctrl Pts',(0.3530194781211,7.800140145157,-0.7712432567487));
#34288=CARTESIAN_POINT('Ctrl Pts',(0.3268098245238,7.761290681241,-0.9498918064517));
#34289=CARTESIAN_POINT('Ctrl Pts',(0.3017673989979,7.719035433425,-1.110873752664));
#34290=CARTESIAN_POINT('Ctrl Pts',(0.27750044695,7.674652834655,-1.256626058432));
#34291=CARTESIAN_POINT('Ctrl Pts',(0.2538473285845,7.629290513098,-1.388548718731));
#34292=CARTESIAN_POINT('Ctrl Pts',(0.2306285320351,7.583757910898,-1.508164313343));
#34293=CARTESIAN_POINT('Ctrl Pts',(0.2077459409351,7.538748776583,-1.616570111714));
#34294=CARTESIAN_POINT('Ctrl Pts',(0.1848495979167,7.494336451159,-1.715813080171));
#34295=CARTESIAN_POINT('Ctrl Pts',(0.1609461047851,7.449222130099,-1.810174952063));
#34296=CARTESIAN_POINT('Ctrl Pts',(0.1337042946379,7.399946526947,-1.90703230257));
#34297=CARTESIAN_POINT('Ctrl Pts',(0.1104061460154,7.3606094987,-1.979544729913));
#34298=CARTESIAN_POINT('Ctrl Pts',(0.09567837415138,7.337327167199,-2.020855911046));
#34299=CARTESIAN_POINT('Ctrl Pts',(0.09337813193118,7.333727280678,-2.027206328594));
#34300=CARTESIAN_POINT('Ctrl Pts',(0.3516735936866,7.689614433451,-0.07882304454856));
#34301=CARTESIAN_POINT('Ctrl Pts',(0.350847645443,7.689489554466,-0.08497125195246));
#34302=CARTESIAN_POINT('Ctrl Pts',(0.3394417549388,7.687568105211,-0.1697648837862));
#34303=CARTESIAN_POINT('Ctrl Pts',(0.3180756196168,7.678929865608,-0.3258309287609));
#34304=CARTESIAN_POINT('Ctrl Pts',(0.2882640593889,7.654890630862,-0.5374733705245));
#34305=CARTESIAN_POINT('Ctrl Pts',(0.2606668037202,7.623311287819,-0.72733912594));
#34306=CARTESIAN_POINT('Ctrl Pts',(0.2345362971087,7.586713311666,-0.8976506379897));
#34307=CARTESIAN_POINT('Ctrl Pts',(0.2095892877477,7.546871805083,-1.051034607769));
#34308=CARTESIAN_POINT('Ctrl Pts',(0.1854463195427,7.505030986202,-1.189768938416));
#34309=CARTESIAN_POINT('Ctrl Pts',(0.1619437477529,7.46228752288,-1.315220328419));
#34310=CARTESIAN_POINT('Ctrl Pts',(0.138910375472,7.419427010875,-1.428824558871));
#34311=CARTESIAN_POINT('Ctrl Pts',(0.1162527672911,7.377116859745,-1.53163170281));
#34312=CARTESIAN_POINT('Ctrl Pts',(0.09364048230928,7.335454123773,-1.625553474636));
#34313=CARTESIAN_POINT('Ctrl Pts',(0.0700942572526,7.293224081819,-1.714671038855));
#34314=CARTESIAN_POINT('Ctrl Pts',(0.04337896997814,7.247270768707,-1.805808681845));
#34315=CARTESIAN_POINT('Ctrl Pts',(0.02066764874285,7.210775637613,-1.87369224103));
#34316=CARTESIAN_POINT('Ctrl Pts',(0.006407516092696,7.189293884623,-1.912158009393));
#34317=CARTESIAN_POINT('Ctrl Pts',(0.004182600943529,7.185975364974,-1.918065761637));
#34318=CARTESIAN_POINT('Ctrl Pts',(0.1756764843762,7.588507551776,-0.05645169963136));
#34319=CARTESIAN_POINT('Ctrl Pts',(0.17485115759,7.588418024305,-0.06243513417407));
#34320=CARTESIAN_POINT('Ctrl Pts',(0.1634561005123,7.586989322095,-0.1449398854917));
#34321=CARTESIAN_POINT('Ctrl Pts',(0.1421623841087,7.579420771145,-0.2964239473798));
#34322=CARTESIAN_POINT('Ctrl Pts',(0.1123948451765,7.557190120433,-0.5023434273139));
#34323=CARTESIAN_POINT('Ctrl Pts',(0.08490615253084,7.527597874674,-0.6866379321841));
#34324=CARTESIAN_POINT('Ctrl Pts',(0.05892627421298,7.49314065782,-0.8516776174722));
#34325=CARTESIAN_POINT('Ctrl Pts',(0.03416085577375,7.455547930377,-1.000117458604));
#34326=CARTESIAN_POINT('Ctrl Pts',(0.01025384696161,7.416083886949,-1.134060645635));
#34327=CARTESIAN_POINT('Ctrl Pts',(-0.01296221266884,7.375817217032,-1.254905212899));
#34328=CARTESIAN_POINT('Ctrl Pts',(-0.03564269543798,7.335541213803,-1.36400630926));
#34329=CARTESIAN_POINT('Ctrl Pts',(-0.05787212820738,7.295916502886,-1.462390721413));
#34330=CARTESIAN_POINT('Ctrl Pts',(-0.07994380918605,7.257099508462,-1.551819675948));
#34331=CARTESIAN_POINT('Ctrl Pts',(-0.1028101008255,7.217967061454,-1.636246280066));
#34332=CARTESIAN_POINT('Ctrl Pts',(-0.1285233380393,7.175787023336,-1.721805374644));
#34333=CARTESIAN_POINT('Ctrl Pts',(-0.1501178409,7.142734270604,-1.784726132061));
#34334=CARTESIAN_POINT('Ctrl Pts',(-0.1634879877075,7.123558780129,-1.819892205208));
#34335=CARTESIAN_POINT('Ctrl Pts',(-0.1655695444196,7.12060357232,-1.825280786222));
#34336=CARTESIAN_POINT('Ctrl Pts',(-0.02667784573404,7.600731964282,-0.03192949709627));
#34337=CARTESIAN_POINT('Ctrl Pts',(-0.02750246349208,7.600681176477,-0.0379261987546));
#34338=CARTESIAN_POINT('Ctrl Pts',(-0.03888513505015,7.599786149475,-0.1205939522383));
#34339=CARTESIAN_POINT('Ctrl Pts',(-0.0600955870907,7.593220562632,-0.271928368777));
#34340=CARTESIAN_POINT('Ctrl Pts',(-0.0898125121055,7.572357130986,-0.4782430106894));
#34341=CARTESIAN_POINT('Ctrl Pts',(-0.1171763833487,7.544087095491,-0.6623591991885));
#34342=CARTESIAN_POINT('Ctrl Pts',(-0.1429830753057,7.510964602637,-0.8269045289223));
#34343=CARTESIAN_POINT('Ctrl Pts',(-0.1675397077981,7.474725301153,-0.974659914962));
#34344=CARTESIAN_POINT('Ctrl Pts',(-0.1911754199796,7.43670106516,-1.10759492696));
#34345=CARTESIAN_POINT('Ctrl Pts',(-0.2140620594393,7.39796467495,-1.227193389711));
#34346=CARTESIAN_POINT('Ctrl Pts',(-0.2363368040245,7.359346164853,-1.334762175216));
#34347=CARTESIAN_POINT('Ctrl Pts',(-0.2580739379069,7.321521134976,-1.43133625717));
#34348=CARTESIAN_POINT('Ctrl Pts',(-0.2795240541205,7.284721753007,-1.518560016082));
#34349=CARTESIAN_POINT('Ctrl Pts',(-0.3016085856319,7.247894134993,-1.60037260569));
#34350=CARTESIAN_POINT('Ctrl Pts',(-0.3261697059415,7.208712817874,-1.682306192782));
#34351=CARTESIAN_POINT('Ctrl Pts',(-0.3464801359011,7.178584859169,-1.741542105518));
#34352=CARTESIAN_POINT('Ctrl Pts',(-0.3588270127402,7.161472253843,-1.774025923849));
#34353=CARTESIAN_POINT('Ctrl Pts',(-0.3607437416807,7.158844301156,-1.778987451663));
#34354=CARTESIAN_POINT('Ctrl Pts',(-0.1093368573593,2.267338017643,-3.503111485524));
#34355=CARTESIAN_POINT('Ctrl Pts',(-0.1083830870411,2.261715711184,-3.504763464173));
#34356=CARTESIAN_POINT('Ctrl Pts',(-0.1024109572104,2.226653555098,-3.515107496462));
#34357=CARTESIAN_POINT('Ctrl Pts',(-0.09166803071108,2.165207556871,-3.533714790978));
#34358=CARTESIAN_POINT('Ctrl Pts',(-0.07707930366217,2.085794285077,-3.558983207447));
#34359=CARTESIAN_POINT('Ctrl Pts',(-0.06322441812029,2.014421046044,-3.582980573135));
#34360=CARTESIAN_POINT('Ctrl Pts',(-0.05003765588103,1.950448046759,-3.605820715331));
#34361=CARTESIAN_POINT('Ctrl Pts',(-0.03741167371015,1.893137336415,-3.627689557913));
#34362=CARTESIAN_POINT('Ctrl Pts',(-0.02742060432543,1.85109146855,-3.644994597799));
#34363=CARTESIAN_POINT('Ctrl Pts',(-0.0216547415189,1.828308833643,-3.654981365119));
#34364=CARTESIAN_POINT('Ctrl Pts',(-0.020047604698,1.822076746678,-3.657765007738));
#34365=CARTESIAN_POINT('Ctrl Pts',(-0.08914856077128,2.30389779074,-3.615858489728));
#34366=CARTESIAN_POINT('Ctrl Pts',(-0.08820964158498,2.298363302287,-3.617484745462));
#34367=CARTESIAN_POINT('Ctrl Pts',(-0.08233249861155,2.263860250828,-3.62766425569));
#34368=CARTESIAN_POINT('Ctrl Pts',(-0.07178380934417,2.203526797407,-3.645935121454));
#34369=CARTESIAN_POINT('Ctrl Pts',(-0.0575231657281,2.125905672972,-3.670635280746));
#34370=CARTESIAN_POINT('Ctrl Pts',(-0.04406846217497,2.056600282344,-3.6939395109));
#34371=CARTESIAN_POINT('Ctrl Pts',(-0.03135539063293,1.994934720186,-3.715959196734));
#34372=CARTESIAN_POINT('Ctrl Pts',(-0.01932659075308,1.940347123965,-3.736793689271));
#34373=CARTESIAN_POINT('Ctrl Pts',(-0.009956155822182,1.900928630607,-3.753023758685));
#34374=CARTESIAN_POINT('Ctrl Pts',(-0.004648641143993,1.87996086452,-3.762216643767));
#34375=CARTESIAN_POINT('Ctrl Pts',(-0.003177995106695,1.874260366703,-3.76476387742));
#34376=CARTESIAN_POINT('Ctrl Pts',(-0.04841933904592,2.342100691839,-3.722337292106));
#34377=CARTESIAN_POINT('Ctrl Pts',(-0.04749593845507,2.336657968252,-3.723936668845));
#34378=CARTESIAN_POINT('Ctrl Pts',(-0.04171805139089,2.302739149594,-3.733944262798));
#34379=CARTESIAN_POINT('Ctrl Pts',(-0.03137232907633,2.243568242753,-3.751863579488));
#34380=CARTESIAN_POINT('Ctrl Pts',(-0.0174545141457,2.167819811241,-3.775969942078));
#34381=CARTESIAN_POINT('Ctrl Pts',(-0.004417978201916,2.10067520558,-3.798549884687));
#34382=CARTESIAN_POINT('Ctrl Pts',(0.007800113273371,2.041420785091,-3.819712239893));
#34383=CARTESIAN_POINT('Ctrl Pts',(0.01920489134338,1.989678689559,-3.839465894962));
#34384=CARTESIAN_POINT('Ctrl Pts',(0.0279267982543,1.953005654392,-3.854572680865));
#34385=CARTESIAN_POINT('Ctrl Pts',(0.03275536498868,1.933934323872,-3.862936003777));
#34386=CARTESIAN_POINT('Ctrl Pts',(0.03408338585636,1.928789306735,-3.865236203394));
#34387=CARTESIAN_POINT('Ctrl Pts',(0.01154374246066,2.380720729223,-3.819130818924));
#34388=CARTESIAN_POINT('Ctrl Pts',(0.01245145500894,2.375370772478,-3.820703023177));
#34389=CARTESIAN_POINT('Ctrl Pts',(0.01812900239146,2.342042565842,-3.830536823706));
#34390=CARTESIAN_POINT('Ctrl Pts',(0.02826954156393,2.284046899391,-3.848100752769));
#34391=CARTESIAN_POINT('Ctrl Pts',(0.04184078447309,2.210191608676,-3.87160683501));
#34392=CARTESIAN_POINT('Ctrl Pts',(0.05445458684907,2.145231381526,-3.893454581602));
#34393=CARTESIAN_POINT('Ctrl Pts',(0.06617229358387,2.088414429887,-3.913750245015));
#34394=CARTESIAN_POINT('Ctrl Pts',(0.07694623617531,2.039548904977,-3.932411260981));
#34395=CARTESIAN_POINT('Ctrl Pts',(0.08501253379338,2.005651305572,-3.946382498285));
#34396=CARTESIAN_POINT('Ctrl Pts',(0.08935692296802,1.988497117739,-3.953907201063));
#34397=CARTESIAN_POINT('Ctrl Pts',(0.09054076134808,1.983913646559,-3.955957669285));
#34398=CARTESIAN_POINT('Ctrl Pts',(-1.96632830365993E-8,2.35518147812891,
-3.79999996594227));
#34399=CARTESIAN_POINT('Ctrl Pts',(-0.00357935201635383,2.31983212279541,
-3.79380037680371));
#34400=CARTESIAN_POINT('Ctrl Pts',(-0.00668325372236177,2.2859060985581,
-3.78742526700976));
#34401=CARTESIAN_POINT('Ctrl Pts',(-0.00933017063364458,2.25352492902307,
-3.7809687846852));
#34402=CARTESIAN_POINT('Ctrl Pts',(-0.0117790651800547,2.22356627443035,
-3.77499532768463));
#34403=CARTESIAN_POINT('Ctrl Pts',(-0.0138399798130133,2.19492932956879,
-3.76895400168668));
#34404=CARTESIAN_POINT('Ctrl Pts',(-0.0155599555445709,2.16735773225228,
-3.76283182924018));
#34405=CARTESIAN_POINT('Ctrl Pts',(-0.0156990395242569,2.16512818481697,
-3.76233676637821));
#34406=CARTESIAN_POINT('Ctrl Pts',(-0.0158358799969592,2.16290558066701,
-3.76184117210061));
#34407=CARTESIAN_POINT('Ctrl Pts',(-0.0159704944353338,2.16068977328618,
-3.76134503811409));
#34408=CARTESIAN_POINT('Ctrl Pts',(-0.0177698122251964,2.13107228434972,
-3.75471348566788));
#34409=CARTESIAN_POINT('Ctrl Pts',(-0.0191729161038338,2.10267382287069,
-3.74798548303885));
#34410=CARTESIAN_POINT('Ctrl Pts',(-0.0202111003075097,2.07533858847079,
-3.74115901064695));
#34411=CARTESIAN_POINT('Ctrl Pts',(-0.0211069940837041,2.05174983968905,
-3.73526815418081));
#34412=CARTESIAN_POINT('Ctrl Pts',(-0.0217311225486786,2.02895149477714,
-3.7293043052384));
#34413=CARTESIAN_POINT('Ctrl Pts',(-0.0220993771361064,2.00682851987961,
-3.72324124653658));
#34414=CARTESIAN_POINT('Ctrl Pts',(-0.0221578652114335,2.00331483595973,
-3.7222782805718));
#34415=CARTESIAN_POINT('Ctrl Pts',(-0.0222098601880988,1.99981809119264,
-3.72131282557032));
#34416=CARTESIAN_POINT('Ctrl Pts',(-0.0222553839599064,1.99633772653508,
-3.72034478903747));
#34417=CARTESIAN_POINT('Ctrl Pts',(-0.0225419057442877,1.97443268105259,
-3.71425206992115));
#34418=CARTESIAN_POINT('Ctrl Pts',(-0.022573946896536,1.95318010085027,
-3.70805690800793));
#34419=CARTESIAN_POINT('Ctrl Pts',(-0.0223572182489124,1.93246260055955,
-3.70170259035036));
#34420=CARTESIAN_POINT('Ctrl Pts',(-0.0223227123773963,1.92916411920508,
-3.70069090467305));
#34421=CARTESIAN_POINT('Ctrl Pts',(-0.0222818493864799,1.92587910948092,
-3.69967520097663));
#34422=CARTESIAN_POINT('Ctrl Pts',(-0.022234595528982,1.92260700285591,
-3.69865526715785));
#34423=CARTESIAN_POINT('Ctrl Pts',(-0.022234582589023,1.92260610682482,
-3.69865498785998));
#34424=CARTESIAN_POINT('Ctrl Pts',(-0.0222345696485847,1.92260521079469,
-3.69865470856179));
#34425=CARTESIAN_POINT('Ctrl Pts',(-0.022234556707667,1.92260431476553,
-3.69865442926329));
#34426=CARTESIAN_POINT('Ctrl Pts',(-0.0219659729272414,1.9040075734149,
-3.69285769595474));
#34427=CARTESIAN_POINT('Ctrl Pts',(-0.0214906543542213,1.88582902904627,
-3.68692322599305));
#34428=CARTESIAN_POINT('Ctrl Pts',(-0.0208084100576887,1.86814906504177,
-3.68086191629441));
#34429=CARTESIAN_POINT('Ctrl Pts',(-0.0206166125285239,1.8631787436642,
-3.67915791637882));
#34430=CARTESIAN_POINT('Ctrl Pts',(-0.0204084646838708,1.85824749485259,
-3.67744394818951));
#34431=CARTESIAN_POINT('Ctrl Pts',(-0.0201840086718301,1.85335644493182,
-3.67572031916525));
#34432=CARTESIAN_POINT('Ctrl Pts',(0.01313183742357,2.35893980927,-3.823805869142));
#34433=CARTESIAN_POINT('Ctrl Pts',(0.01303186504026,2.353957576536,-3.82385436109));
#34434=CARTESIAN_POINT('Ctrl Pts',(0.01123027883039,2.264631434664,-3.82471367541));
#34435=CARTESIAN_POINT('Ctrl Pts',(0.00760883944032,2.10029230713,-3.825952350518));
#34436=CARTESIAN_POINT('Ctrl Pts',(0.002704317644358,1.905594454076,-3.826393794893));
#34437=CARTESIAN_POINT('Ctrl Pts',(-0.0002703855987072,1.795386308729,-3.826069286647));
#34438=CARTESIAN_POINT('Ctrl Pts',(-0.001263515685753,1.759172878611,-3.825885856397));
#34439=CARTESIAN_POINT('Ctrl Pts',(-0.1220155422729,2.480509211462,-3.559282264932));
#34440=CARTESIAN_POINT('Ctrl Pts',(-0.1210052566975,2.475681572059,-3.558834796486));
#34441=CARTESIAN_POINT('Ctrl Pts',(-0.1028036746325,2.389157129411,-3.550915651626));
#34442=CARTESIAN_POINT('Ctrl Pts',(-0.06637047515481,2.230896427315,-3.539852558722));
#34443=CARTESIAN_POINT('Ctrl Pts',(-0.0174057286524,2.046314967408,-3.537170858724));
#34444=CARTESIAN_POINT('Ctrl Pts',(0.01211878202876,1.943696215842,-3.541453508649));
#34445=CARTESIAN_POINT('Ctrl Pts',(0.02195442675702,1.910230935709,-3.543633877626));
#34446=CARTESIAN_POINT('Ctrl Pts',(-0.4243708118278,2.566620235427,-3.494607553578));
#34447=CARTESIAN_POINT('Ctrl Pts',(-0.4230739478696,2.561902098825,-3.492966852937));
#34448=CARTESIAN_POINT('Ctrl Pts',(-0.3995937923515,2.477362178471,-3.463646745939));
#34449=CARTESIAN_POINT('Ctrl Pts',(-0.3487237350337,2.323406995932,-3.413015804336));
#34450=CARTESIAN_POINT('Ctrl Pts',(-0.2708767291174,2.145991261584,-3.365007313014));
#34451=CARTESIAN_POINT('Ctrl Pts',(-0.2195329377334,2.048748290915,-3.345376679566));
#34452=CARTESIAN_POINT('Ctrl Pts',(-0.201883686884,2.017229602646,-3.339993364004));
#34453=CARTESIAN_POINT('Ctrl Pts',(-0.690961983047,2.559466295669,-3.673198060413));
#34454=CARTESIAN_POINT('Ctrl Pts',(-0.6903946011995,2.554739061783,-3.670467876084));
#34455=CARTESIAN_POINT('Ctrl Pts',(-0.6799039890472,2.4700342711,-3.621490833275));
#34456=CARTESIAN_POINT('Ctrl Pts',(-0.6499063603548,2.315721394201,-3.530587976339));
#34457=CARTESIAN_POINT('Ctrl Pts',(-0.5875528502187,2.137710345031,-3.425477056041));
#34458=CARTESIAN_POINT('Ctrl Pts',(-0.5397170591296,2.04002076473,-3.369465755649));
#34459=CARTESIAN_POINT('Ctrl Pts',(-0.5225146677906,2.008340357318,-3.351668795621));
#34460=CARTESIAN_POINT('Origin',(-0.4330128001874,2.355181195091,-4.049999829751));
#34461=CARTESIAN_POINT('Ctrl Pts',(0.1654598430731,3.816833346673,-4.09081615578));
#34462=CARTESIAN_POINT('Ctrl Pts',(0.1654730735783,3.811222474592,-4.090839257127));
#34463=CARTESIAN_POINT('Ctrl Pts',(0.1656678347127,3.645978055895,-4.091179623035));
#34464=CARTESIAN_POINT('Ctrl Pts',(0.1547816615116,3.320020093713,-4.072101884476));
#34465=CARTESIAN_POINT('Ctrl Pts',(0.10512844909,2.829224950023,-3.985158819806));
#34466=CARTESIAN_POINT('Ctrl Pts',(0.04761048988404,2.502918756874,-3.884629417663));
#34467=CARTESIAN_POINT('Ctrl Pts',(0.01060629136168,2.333799331458,-3.820069159035));
#34468=CARTESIAN_POINT('Ctrl Pts',(0.009485886303509,2.328709728431,-3.818114554056));
#34469=CARTESIAN_POINT('Ctrl Pts',(0.07652291890888,3.815887979875,-3.897696692651));
#34470=CARTESIAN_POINT('Ctrl Pts',(0.0765359932756,3.810592215503,-3.897718314945));
#34471=CARTESIAN_POINT('Ctrl Pts',(0.07672846980537,3.654627998194,-3.898036866885));
#34472=CARTESIAN_POINT('Ctrl Pts',(0.0659656221111,3.34697569895,-3.880183328377));
#34473=CARTESIAN_POINT('Ctrl Pts',(0.01686163208697,2.883542177093,-3.798793107701));
#34474=CARTESIAN_POINT('Ctrl Pts',(-0.04004963525953,2.575146492001,-3.704622957279));
#34475=CARTESIAN_POINT('Ctrl Pts',(-0.07668074743997,2.415194449956,-3.644109787001));
#34476=CARTESIAN_POINT('Ctrl Pts',(-0.07778986621121,2.410380629126,-3.642277679727));
#34477=CARTESIAN_POINT('Ctrl Pts',(-0.1058150100366,3.8150580125,-3.788344136655));
#34478=CARTESIAN_POINT('Ctrl Pts',(-0.1058022557841,3.810038889687,-3.788364161843));
#34479=CARTESIAN_POINT('Ctrl Pts',(-0.1056144631364,3.662222079724,-3.788659126644));
#34480=CARTESIAN_POINT('Ctrl Pts',(-0.1161244696433,3.370640483808,-3.772131476753));
#34481=CARTESIAN_POINT('Ctrl Pts',(-0.164102447323,2.930897223765,-3.696717648248));
#34482=CARTESIAN_POINT('Ctrl Pts',(-0.2197698787915,2.637543693865,-3.60930318436));
#34483=CARTESIAN_POINT('Ctrl Pts',(-0.2556360916734,2.485096894578,-3.553035639014));
#34484=CARTESIAN_POINT('Ctrl Pts',(-0.2567220713694,2.480508670394,-3.551331993714));
#34485=CARTESIAN_POINT('Ctrl Pts',(-0.318063882194,3.814632439165,-3.800835044618));
#34486=CARTESIAN_POINT('Ctrl Pts',(-0.3180515005676,3.809755165178,-3.800853910757));
#34487=CARTESIAN_POINT('Ctrl Pts',(-0.317869160152,3.666116041517,-3.801131728292));
#34488=CARTESIAN_POINT('Ctrl Pts',(-0.3280848490852,3.382774370883,-3.785569981205));
#34489=CARTESIAN_POINT('Ctrl Pts',(-0.3747521019391,2.954801064162,-3.714475113467));
#34490=CARTESIAN_POINT('Ctrl Pts',(-0.4289716571276,2.668383658588,-3.631860441071));
#34491=CARTESIAN_POINT('Ctrl Pts',(-0.463947495668,2.519166636135,-3.578558730762));
#34492=CARTESIAN_POINT('Ctrl Pts',(-0.4650065405256,2.5146752703,-3.576944781249));
#34493=CARTESIAN_POINT('Origin',(-0.2886751345948,3.800000001415,-4.3));
#34494=CARTESIAN_POINT('Ctrl Pts',(0.009474644457224,5.271341047008,-3.81809495663));
#34495=CARTESIAN_POINT('Ctrl Pts',(0.01059883418097,5.266234517663,-3.820056164353));
#34496=CARTESIAN_POINT('Ctrl Pts',(0.04384970191935,5.114274997728,-3.878067830231));
#34497=CARTESIAN_POINT('Ctrl Pts',(0.09915364759026,4.8078509,-3.974708076039));
#34498=CARTESIAN_POINT('Ctrl Pts',(0.1527214809499,4.318896431654,-4.068489655631));
#34499=CARTESIAN_POINT('Ctrl Pts',(0.1656911193838,3.973918157182,-4.091220206062));
#34500=CARTESIAN_POINT('Ctrl Pts',(0.1654730928291,3.788778562717,-4.090839298714));
#34501=CARTESIAN_POINT('Ctrl Pts',(0.1654598555027,3.783168271439,-4.090816203677));
#34502=CARTESIAN_POINT('Ctrl Pts',(-0.07780099825573,5.189667390479,-3.64225930114));
#34503=CARTESIAN_POINT('Ctrl Pts',(-0.07668813259209,5.184837560174,-3.644097597763));
#34504=CARTESIAN_POINT('Ctrl Pts',(-0.04377252156913,5.041115244204,-3.698472705015));
#34505=CARTESIAN_POINT('Ctrl Pts',(0.01095113947594,4.751489226246,-3.78900612516));
#34506=CARTESIAN_POINT('Ctrl Pts',(0.06392901869112,4.289755505572,-3.876803425784));
#34507=CARTESIAN_POINT('Ctrl Pts',(0.07675145353046,3.96415083195,-3.898074824767));
#34508=CARTESIAN_POINT('Ctrl Pts',(0.07653600951855,3.789408763611,-3.897718345517));
#34509=CARTESIAN_POINT('Ctrl Pts',(0.07652293035462,3.784113547511,-3.897696729157));
#34510=CARTESIAN_POINT('Ctrl Pts',(-0.2567329809504,5.119537094511,-3.551314900398));
#34511=CARTESIAN_POINT('Ctrl Pts',(-0.2556433318048,5.114933610283,-3.553024302135));
#34512=CARTESIAN_POINT('Ctrl Pts',(-0.2234150620255,4.977955008216,-3.603584480384));
#34513=CARTESIAN_POINT('Ctrl Pts',(-0.1698810969299,4.702401341059,-3.687639726247));
#34514=CARTESIAN_POINT('Ctrl Pts',(-0.1181127380514,4.264172564127,-3.769003987438));
#34515=CARTESIAN_POINT('Ctrl Pts',(-0.1055920991109,3.955575758191,-3.788694233295));
#34516=CARTESIAN_POINT('Ctrl Pts',(-0.1058022484096,3.789962038378,-3.788364190614));
#34517=CARTESIAN_POINT('Ctrl Pts',(-0.1058150033097,3.784943435394,-3.788344170997));
#34518=CARTESIAN_POINT('Ctrl Pts',(-0.4650171874587,5.085369528077,-3.576928594638));
#34519=CARTESIAN_POINT('Ctrl Pts',(-0.4639545632973,5.080863223263,-3.578547998901));
#34520=CARTESIAN_POINT('Ctrl Pts',(-0.4325263870696,4.946786683863,-3.626443236047));
#34521=CARTESIAN_POINT('Ctrl Pts',(-0.380377277119,4.677679646005,-3.705904659284));
#34522=CARTESIAN_POINT('Ctrl Pts',(-0.3300168497897,4.251055587502,-3.7826271049));
#34523=CARTESIAN_POINT('Ctrl Pts',(-0.3178475137206,3.951178776577,-3.801164753472));
#34524=CARTESIAN_POINT('Ctrl Pts',(-0.3180514997547,3.790245736745,-3.800853950616));
#34525=CARTESIAN_POINT('Ctrl Pts',(-0.3180638771985,3.785368968127,-3.800835089823));
#34526=CARTESIAN_POINT('Origin',(1.,18.3911851122,3.532050807569));
#52141=UNCERTAINTY_MEASURE_WITH_UNIT(LENGTH_MEASURE(0.01),#52165,
'DISTANCE_ACCURACY_VALUE',
'Maximum model space distance between geometric entities at asserted c
onnectivities');
#52149=UNCERTAINTY_MEASURE_WITH_UNIT(LENGTH_MEASURE(0.01),#52165,
'DISTANCE_ACCURACY_VALUE',
'Maximum model space distance between geometric entities at asserted c
onnectivities');
#52156=(
GEOMETRIC_REPRESENTATION_CONTEXT(3)
GLOBAL_UNCERTAINTY_ASSIGNED_CONTEXT((#52141))
GLOBAL_UNIT_ASSIGNED_CONTEXT((#52165,#52167,#52168))
REPRESENTATION_CONTEXT('','3D')
);
#52164=(
GEOMETRIC_REPRESENTATION_CONTEXT(3)
GLOBAL_UNCERTAINTY_ASSIGNED_CONTEXT((#52149))
GLOBAL_UNIT_ASSIGNED_CONTEXT((#52165,#52167,#52168))
REPRESENTATION_CONTEXT('','3D')
);
#52165=(
LENGTH_UNIT()
NAMED_UNIT(*)
SI_UNIT(.MILLI.,.METRE.)
);
#52167=(
NAMED_UNIT(*)
PLANE_ANGLE_UNIT()
SI_UNIT($,.RADIAN.)
);
#52168=(
NAMED_UNIT(*)
SI_UNIT($,.STERADIAN.)
SOLID_ANGLE_UNIT()
);
#52175=SHAPE_DEFINITION_REPRESENTATION(#52189,#52216);
#52189=PRODUCT_DEFINITION_SHAPE('',$,#52231);
#52216=SHAPE_REPRESENTATION('',(#9776),#52156);
#52224=PRODUCT_DEFINITION_CONTEXT('part definition',#52268,'design');
#52231=PRODUCT_DEFINITION('Tuning Key / Button','Tuning Key / Button',#52245,
#52224);
#52245=PRODUCT_DEFINITION_FORMATION('',$,#52276);
#52268=APPLICATION_CONTEXT('Managed model based 3d engineering');
#52269=PRODUCT_CONTEXT('part definition',#52268,'mechanical');
#52276=PRODUCT('Tuning Key / Button','Tuning Key / Button',
'NOT SPECIFIED',(#52269));
#52312=COLOUR_RGB('Grey',0.48,0.52,0.57);
#52313=FILL_AREA_STYLE_COLOUR('',#52312);
#52314=FILL_AREA_STYLE('',(#52313));
#52315=SURFACE_STYLE_FILL_AREA(#52314);
#52316=SURFACE_SIDE_STYLE('',(#52315));
#52317=SURFACE_STYLE_USAGE(.BOTH.,#52316);
#52318=PRESENTATION_STYLE_ASSIGNMENT((#52317));
ENDSEC;
END-ISO-10303-21;
